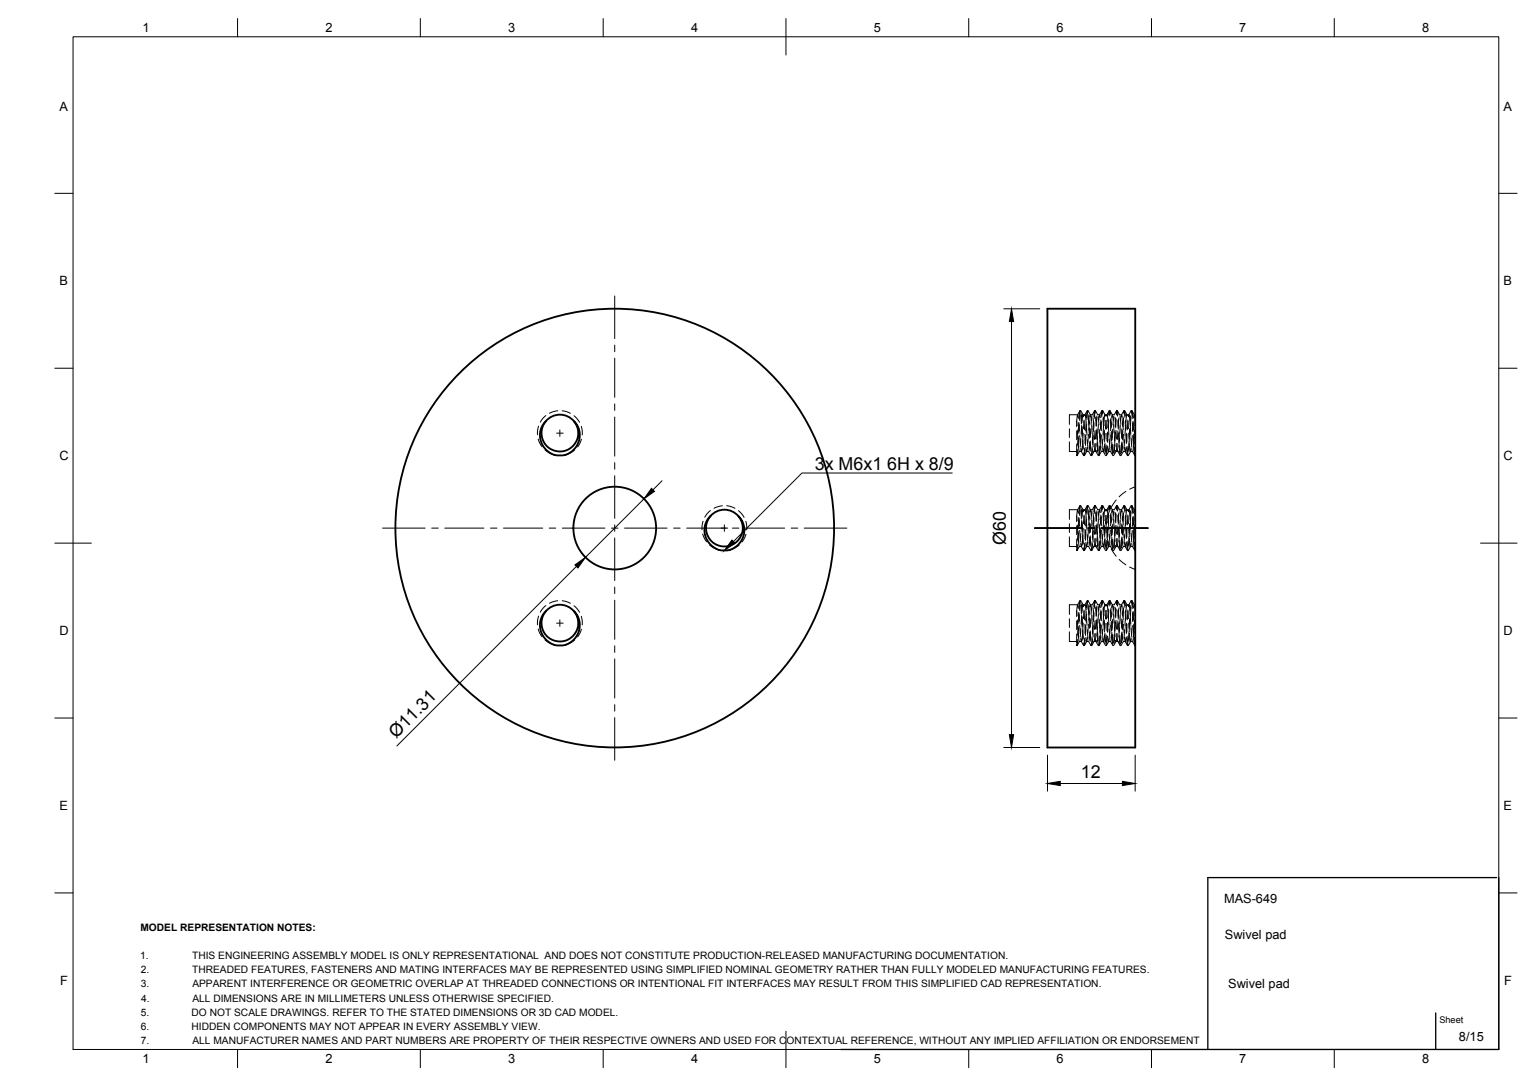
ISO-10303-21;
HEADER;
/* Generated by software containing ST-Developer
 * from STEP Tools, Inc. (www.steptools.com) 
 */

FILE_DESCRIPTION(
/* description */ ('Independent equipment support assembly with bolted 600 x 500 mm welde
d perimeter frame, four adjustable legs and swivel feet. Nominal overa
ll height 518 mm. No load rating assigned.'),
/* implementation_level */ '2;1');

FILE_NAME(
/* name */ 'Swivel pad.step',
/* time_stamp */ '2026-11-07T17:30:39-08:00',
/* author */ (''),
/* organization */ (''),
/* preprocessor_version */ 'ST-DEVELOPER v20.2',
/* originating_system */ 'Autodesk Translation Framework v15.17.0.0',
/* authorisation */ '');

FILE_SCHEMA (('AUTOMOTIVE_DESIGN { 1 0 10303 214 3 1 1 }'));
ENDSEC;

DATA;
#10=MECHANICAL_DESIGN_GEOMETRIC_PRESENTATION_REPRESENTATION('',(#2217),#63755);
#11=SPHERICAL_SURFACE('',#15224,6.);
#273=B_SPLINE_SURFACE_WITH_KNOTS('',3,3,((#49030,#49031,#49032,#49033,#49034,
#49035,#49036,#49037,#49038,#49039,#49040,#49041,#49042,#49043,#49044,#49045,
#49046,#49047,#49048,#49049,#49050,#49051,#49052,#49053,#49054,#49055,#49056,
#49057,#49058,#49059,#49060,#49061,#49062,#49063,#49064,#49065,#49066,#49067,
#49068,#49069,#49070,#49071,#49072,#49073,#49074,#49075,#49076,#49077,#49078,
#49079,#49080,#49081,#49082,#49083,#49084,#49085),(#49086,#49087,#49088,
#49089,#49090,#49091,#49092,#49093,#49094,#49095,#49096,#49097,#49098,#49099,
#49100,#49101,#49102,#49103,#49104,#49105,#49106,#49107,#49108,#49109,#49110,
#49111,#49112,#49113,#49114,#49115,#49116,#49117,#49118,#49119,#49120,#49121,
#49122,#49123,#49124,#49125,#49126,#49127,#49128,#49129,#49130,#49131,#49132,
#49133,#49134,#49135,#49136,#49137,#49138,#49139,#49140,#49141),(#49142,
#49143,#49144,#49145,#49146,#49147,#49148,#49149,#49150,#49151,#49152,#49153,
#49154,#49155,#49156,#49157,#49158,#49159,#49160,#49161,#49162,#49163,#49164,
#49165,#49166,#49167,#49168,#49169,#49170,#49171,#49172,#49173,#49174,#49175,
#49176,#49177,#49178,#49179,#49180,#49181,#49182,#49183,#49184,#49185,#49186,
#49187,#49188,#49189,#49190,#49191,#49192,#49193,#49194,#49195,#49196,#49197),
(#49198,#49199,#49200,#49201,#49202,#49203,#49204,#49205,#49206,#49207,
#49208,#49209,#49210,#49211,#49212,#49213,#49214,#49215,#49216,#49217,#49218,
#49219,#49220,#49221,#49222,#49223,#49224,#49225,#49226,#49227,#49228,#49229,
#49230,#49231,#49232,#49233,#49234,#49235,#49236,#49237,#49238,#49239,#49240,
#49241,#49242,#49243,#49244,#49245,#49246,#49247,#49248,#49249,#49250,#49251,
#49252,#49253)),.UNSPECIFIED.,.F.,.F.,.F.,(4,4),(4,1,1,1,1,1,1,1,1,1,1,
1,1,1,1,1,1,1,1,1,1,1,1,1,1,1,1,1,1,1,1,1,1,1,1,1,1,1,1,1,1,1,1,1,1,1,1,
1,1,1,1,1,1,4),(0.,0.0642013499338865),(11.8589888623078,12.8454497557128,
13.8319106491178,14.8183715425228,15.8048324359278,16.7912933293328,17.7777542227378,
18.7642151161428,19.7506760095478,20.7371369029528,21.7235977963578,22.7100586897628,
23.6965195831678,24.6829804765729,25.6694413699779,26.6559022633829,27.6423631567879,
28.6288240501929,29.6152849435979,30.6017458370029,31.5882067304079,32.5746676238129,
33.5611285172179,34.5475894106229,35.5340503040279,36.5205111974329,37.5069720908379,
38.4934329842429,39.4798938776479,40.4663547710529,41.4528156644579,42.4392765578629,
43.4257374512679,44.4121983446729,45.3986592380779,46.3851201314829,47.3715810248879,
48.3580419182929,49.3445028116979,50.3309637051029,51.3174245985079,52.3038854919129,
53.2903463853179,54.2768072787229,55.2632681721279,56.2497290655329,57.2361899589379,
58.2226508523429,59.2091117457479,60.1955726391529,61.1820335325579,62.1684944259629,
63.154955319368,64.141416212773),.UNSPECIFIED.);
#274=B_SPLINE_SURFACE_WITH_KNOTS('',3,3,((#49370,#49371,#49372,#49373,#49374,
#49375,#49376,#49377,#49378,#49379,#49380,#49381,#49382,#49383,#49384,#49385,
#49386,#49387,#49388,#49389,#49390,#49391,#49392,#49393,#49394,#49395,#49396,
#49397,#49398,#49399,#49400,#49401,#49402,#49403,#49404,#49405,#49406,#49407,
#49408,#49409,#49410,#49411,#49412,#49413,#49414,#49415,#49416,#49417,#49418,
#49419,#49420,#49421,#49422,#49423,#49424,#49425),(#49426,#49427,#49428,
#49429,#49430,#49431,#49432,#49433,#49434,#49435,#49436,#49437,#49438,#49439,
#49440,#49441,#49442,#49443,#49444,#49445,#49446,#49447,#49448,#49449,#49450,
#49451,#49452,#49453,#49454,#49455,#49456,#49457,#49458,#49459,#49460,#49461,
#49462,#49463,#49464,#49465,#49466,#49467,#49468,#49469,#49470,#49471,#49472,
#49473,#49474,#49475,#49476,#49477,#49478,#49479,#49480,#49481),(#49482,
#49483,#49484,#49485,#49486,#49487,#49488,#49489,#49490,#49491,#49492,#49493,
#49494,#49495,#49496,#49497,#49498,#49499,#49500,#49501,#49502,#49503,#49504,
#49505,#49506,#49507,#49508,#49509,#49510,#49511,#49512,#49513,#49514,#49515,
#49516,#49517,#49518,#49519,#49520,#49521,#49522,#49523,#49524,#49525,#49526,
#49527,#49528,#49529,#49530,#49531,#49532,#49533,#49534,#49535,#49536,#49537),
(#49538,#49539,#49540,#49541,#49542,#49543,#49544,#49545,#49546,#49547,
#49548,#49549,#49550,#49551,#49552,#49553,#49554,#49555,#49556,#49557,#49558,
#49559,#49560,#49561,#49562,#49563,#49564,#49565,#49566,#49567,#49568,#49569,
#49570,#49571,#49572,#49573,#49574,#49575,#49576,#49577,#49578,#49579,#49580,
#49581,#49582,#49583,#49584,#49585,#49586,#49587,#49588,#49589,#49590,#49591,
#49592,#49593)),.UNSPECIFIED.,.F.,.F.,.F.,(4,4),(4,1,1,1,1,1,1,1,1,1,1,
1,1,1,1,1,1,1,1,1,1,1,1,1,1,1,1,1,1,1,1,1,1,1,1,1,1,1,1,1,1,1,1,1,1,1,1,
1,1,1,1,1,1,4),(0.,0.0642013499338865),(14.3984001269719,15.3848610203769,
16.3713219137819,17.3577828071869,18.3442437005919,19.3307045939969,20.3171654874019,
21.3036263808069,22.2900872742119,23.2765481676169,24.2630090610219,25.2494699544269,
26.2359308478319,27.2223917412369,28.2088526346419,29.1953135280469,30.1817744214519,
31.1682353148569,32.1546962082619,33.1411571016669,34.1276179950719,35.1140788884769,
36.1005397818819,37.0870006752869,38.0734615686919,39.0599224620969,40.0463833555019,
41.0328442489069,42.0193051423119,43.0057660357169,43.9922269291219,44.9786878225269,
45.9651487159319,46.9516096093369,47.9380705027419,48.9245313961469,49.9109922895519,
50.897453182957,51.883914076362,52.870374969767,53.856835863172,54.843296756577,
55.829757649982,56.816218543387,57.802679436792,58.789140330197,59.775601223602,
60.762062117007,61.748523010412,62.734983903817,63.721444797222,64.707905690627,
65.694366584032,66.680827477437),.UNSPECIFIED.);
#275=B_SPLINE_SURFACE_WITH_KNOTS('',3,3,((#49922,#49923,#49924,#49925,#49926,
#49927,#49928,#49929,#49930,#49931,#49932,#49933,#49934,#49935,#49936,#49937,
#49938,#49939,#49940,#49941,#49942,#49943,#49944,#49945,#49946,#49947,#49948,
#49949,#49950,#49951,#49952,#49953,#49954,#49955,#49956,#49957,#49958,#49959,
#49960,#49961,#49962,#49963,#49964,#49965,#49966,#49967,#49968,#49969,#49970,
#49971,#49972,#49973,#49974,#49975,#49976,#49977),(#49978,#49979,#49980,
#49981,#49982,#49983,#49984,#49985,#49986,#49987,#49988,#49989,#49990,#49991,
#49992,#49993,#49994,#49995,#49996,#49997,#49998,#49999,#50000,#50001,#50002,
#50003,#50004,#50005,#50006,#50007,#50008,#50009,#50010,#50011,#50012,#50013,
#50014,#50015,#50016,#50017,#50018,#50019,#50020,#50021,#50022,#50023,#50024,
#50025,#50026,#50027,#50028,#50029,#50030,#50031,#50032,#50033),(#50034,
#50035,#50036,#50037,#50038,#50039,#50040,#50041,#50042,#50043,#50044,#50045,
#50046,#50047,#50048,#50049,#50050,#50051,#50052,#50053,#50054,#50055,#50056,
#50057,#50058,#50059,#50060,#50061,#50062,#50063,#50064,#50065,#50066,#50067,
#50068,#50069,#50070,#50071,#50072,#50073,#50074,#50075,#50076,#50077,#50078,
#50079,#50080,#50081,#50082,#50083,#50084,#50085,#50086,#50087,#50088,#50089),
(#50090,#50091,#50092,#50093,#50094,#50095,#50096,#50097,#50098,#50099,
#50100,#50101,#50102,#50103,#50104,#50105,#50106,#50107,#50108,#50109,#50110,
#50111,#50112,#50113,#50114,#50115,#50116,#50117,#50118,#50119,#50120,#50121,
#50122,#50123,#50124,#50125,#50126,#50127,#50128,#50129,#50130,#50131,#50132,
#50133,#50134,#50135,#50136,#50137,#50138,#50139,#50140,#50141,#50142,#50143,
#50144,#50145)),.UNSPECIFIED.,.F.,.F.,.F.,(4,4),(4,1,1,1,1,1,1,1,1,1,1,
1,1,1,1,1,1,1,1,1,1,1,1,1,1,1,1,1,1,1,1,1,1,1,1,1,1,1,1,1,1,1,1,1,1,1,1,
1,1,1,1,1,1,4),(0.,0.0642013499338863),(11.8589888623078,12.8454497557128,
13.8319106491178,14.8183715425228,15.8048324359278,16.7912933293328,17.7777542227378,
18.7642151161428,19.7506760095478,20.7371369029528,21.7235977963578,22.7100586897628,
23.6965195831678,24.6829804765729,25.6694413699779,26.6559022633829,27.6423631567879,
28.6288240501929,29.6152849435979,30.6017458370029,31.5882067304079,32.5746676238129,
33.5611285172179,34.5475894106229,35.5340503040279,36.5205111974329,37.5069720908379,
38.4934329842429,39.4798938776479,40.4663547710529,41.4528156644579,42.4392765578629,
43.4257374512679,44.4121983446729,45.3986592380779,46.3851201314829,47.3715810248879,
48.3580419182929,49.3445028116979,50.3309637051029,51.3174245985079,52.3038854919129,
53.2903463853179,54.2768072787229,55.2632681721279,56.2497290655329,57.2361899589379,
58.2226508523429,59.2091117457479,60.1955726391529,61.1820335325579,62.1684944259629,
63.154955319368,64.141416212773),.UNSPECIFIED.);
#276=B_SPLINE_SURFACE_WITH_KNOTS('',3,3,((#50262,#50263,#50264,#50265,#50266,
#50267,#50268,#50269,#50270,#50271,#50272,#50273,#50274,#50275,#50276,#50277,
#50278,#50279,#50280,#50281,#50282,#50283,#50284,#50285,#50286,#50287,#50288,
#50289,#50290,#50291,#50292,#50293,#50294,#50295,#50296,#50297,#50298,#50299,
#50300,#50301,#50302,#50303,#50304,#50305,#50306,#50307,#50308,#50309,#50310,
#50311,#50312,#50313,#50314,#50315,#50316,#50317),(#50318,#50319,#50320,
#50321,#50322,#50323,#50324,#50325,#50326,#50327,#50328,#50329,#50330,#50331,
#50332,#50333,#50334,#50335,#50336,#50337,#50338,#50339,#50340,#50341,#50342,
#50343,#50344,#50345,#50346,#50347,#50348,#50349,#50350,#50351,#50352,#50353,
#50354,#50355,#50356,#50357,#50358,#50359,#50360,#50361,#50362,#50363,#50364,
#50365,#50366,#50367,#50368,#50369,#50370,#50371,#50372,#50373),(#50374,
#50375,#50376,#50377,#50378,#50379,#50380,#50381,#50382,#50383,#50384,#50385,
#50386,#50387,#50388,#50389,#50390,#50391,#50392,#50393,#50394,#50395,#50396,
#50397,#50398,#50399,#50400,#50401,#50402,#50403,#50404,#50405,#50406,#50407,
#50408,#50409,#50410,#50411,#50412,#50413,#50414,#50415,#50416,#50417,#50418,
#50419,#50420,#50421,#50422,#50423,#50424,#50425,#50426,#50427,#50428,#50429),
(#50430,#50431,#50432,#50433,#50434,#50435,#50436,#50437,#50438,#50439,
#50440,#50441,#50442,#50443,#50444,#50445,#50446,#50447,#50448,#50449,#50450,
#50451,#50452,#50453,#50454,#50455,#50456,#50457,#50458,#50459,#50460,#50461,
#50462,#50463,#50464,#50465,#50466,#50467,#50468,#50469,#50470,#50471,#50472,
#50473,#50474,#50475,#50476,#50477,#50478,#50479,#50480,#50481,#50482,#50483,
#50484,#50485)),.UNSPECIFIED.,.F.,.F.,.F.,(4,4),(4,1,1,1,1,1,1,1,1,1,1,
1,1,1,1,1,1,1,1,1,1,1,1,1,1,1,1,1,1,1,1,1,1,1,1,1,1,1,1,1,1,1,1,1,1,1,1,
1,1,1,1,1,1,4),(0.,0.0642013499338863),(14.3984001269719,15.3848610203769,
16.3713219137819,17.3577828071869,18.3442437005919,19.3307045939969,20.3171654874019,
21.3036263808069,22.2900872742119,23.2765481676169,24.2630090610219,25.2494699544269,
26.2359308478319,27.2223917412369,28.2088526346419,29.1953135280469,30.1817744214519,
31.1682353148569,32.1546962082619,33.1411571016669,34.1276179950719,35.1140788884769,
36.1005397818819,37.0870006752869,38.0734615686919,39.0599224620969,40.0463833555019,
41.0328442489069,42.0193051423119,43.0057660357169,43.9922269291219,44.9786878225269,
45.9651487159319,46.9516096093369,47.9380705027419,48.9245313961469,49.9109922895519,
50.897453182957,51.883914076362,52.870374969767,53.856835863172,54.843296756577,
55.829757649982,56.816218543387,57.802679436792,58.789140330197,59.775601223602,
60.762062117007,61.748523010412,62.734983903817,63.721444797222,64.707905690627,
65.694366584032,66.680827477437),.UNSPECIFIED.);
#277=B_SPLINE_SURFACE_WITH_KNOTS('',3,3,((#50814,#50815,#50816,#50817,#50818,
#50819,#50820,#50821,#50822,#50823,#50824,#50825,#50826,#50827,#50828,#50829,
#50830,#50831,#50832,#50833,#50834,#50835,#50836,#50837,#50838,#50839,#50840,
#50841,#50842,#50843,#50844,#50845,#50846,#50847,#50848,#50849,#50850,#50851,
#50852,#50853,#50854,#50855,#50856,#50857,#50858,#50859,#50860,#50861,#50862,
#50863,#50864,#50865,#50866,#50867,#50868,#50869),(#50870,#50871,#50872,
#50873,#50874,#50875,#50876,#50877,#50878,#50879,#50880,#50881,#50882,#50883,
#50884,#50885,#50886,#50887,#50888,#50889,#50890,#50891,#50892,#50893,#50894,
#50895,#50896,#50897,#50898,#50899,#50900,#50901,#50902,#50903,#50904,#50905,
#50906,#50907,#50908,#50909,#50910,#50911,#50912,#50913,#50914,#50915,#50916,
#50917,#50918,#50919,#50920,#50921,#50922,#50923,#50924,#50925),(#50926,
#50927,#50928,#50929,#50930,#50931,#50932,#50933,#50934,#50935,#50936,#50937,
#50938,#50939,#50940,#50941,#50942,#50943,#50944,#50945,#50946,#50947,#50948,
#50949,#50950,#50951,#50952,#50953,#50954,#50955,#50956,#50957,#50958,#50959,
#50960,#50961,#50962,#50963,#50964,#50965,#50966,#50967,#50968,#50969,#50970,
#50971,#50972,#50973,#50974,#50975,#50976,#50977,#50978,#50979,#50980,#50981),
(#50982,#50983,#50984,#50985,#50986,#50987,#50988,#50989,#50990,#50991,
#50992,#50993,#50994,#50995,#50996,#50997,#50998,#50999,#51000,#51001,#51002,
#51003,#51004,#51005,#51006,#51007,#51008,#51009,#51010,#51011,#51012,#51013,
#51014,#51015,#51016,#51017,#51018,#51019,#51020,#51021,#51022,#51023,#51024,
#51025,#51026,#51027,#51028,#51029,#51030,#51031,#51032,#51033,#51034,#51035,
#51036,#51037)),.UNSPECIFIED.,.F.,.F.,.F.,(4,4),(4,1,1,1,1,1,1,1,1,1,1,
1,1,1,1,1,1,1,1,1,1,1,1,1,1,1,1,1,1,1,1,1,1,1,1,1,1,1,1,1,1,1,1,1,1,1,1,
1,1,1,1,1,1,4),(0.,0.0642013499338863),(11.8589888623078,12.8454497557128,
13.8319106491178,14.8183715425228,15.8048324359278,16.7912933293328,17.7777542227378,
18.7642151161429,19.7506760095479,20.7371369029529,21.7235977963579,22.7100586897629,
23.6965195831679,24.6829804765729,25.6694413699779,26.6559022633829,27.6423631567879,
28.6288240501929,29.6152849435979,30.6017458370029,31.5882067304079,32.5746676238129,
33.5611285172179,34.5475894106229,35.5340503040279,36.5205111974329,37.5069720908379,
38.4934329842429,39.4798938776479,40.4663547710529,41.4528156644579,42.4392765578629,
43.4257374512679,44.4121983446729,45.3986592380779,46.3851201314829,47.3715810248879,
48.3580419182929,49.3445028116979,50.3309637051029,51.3174245985079,52.3038854919129,
53.2903463853179,54.2768072787229,55.2632681721279,56.2497290655329,57.2361899589379,
58.222650852343,59.209111745748,60.195572639153,61.182033532558,62.168494425963,
63.154955319368,64.141416212773),.UNSPECIFIED.);
#278=B_SPLINE_SURFACE_WITH_KNOTS('',3,3,((#51154,#51155,#51156,#51157,#51158,
#51159,#51160,#51161,#51162,#51163,#51164,#51165,#51166,#51167,#51168,#51169,
#51170,#51171,#51172,#51173,#51174,#51175,#51176,#51177,#51178,#51179,#51180,
#51181,#51182,#51183,#51184,#51185,#51186,#51187,#51188,#51189,#51190,#51191,
#51192,#51193,#51194,#51195,#51196,#51197,#51198,#51199,#51200,#51201,#51202,
#51203,#51204,#51205,#51206,#51207,#51208,#51209),(#51210,#51211,#51212,
#51213,#51214,#51215,#51216,#51217,#51218,#51219,#51220,#51221,#51222,#51223,
#51224,#51225,#51226,#51227,#51228,#51229,#51230,#51231,#51232,#51233,#51234,
#51235,#51236,#51237,#51238,#51239,#51240,#51241,#51242,#51243,#51244,#51245,
#51246,#51247,#51248,#51249,#51250,#51251,#51252,#51253,#51254,#51255,#51256,
#51257,#51258,#51259,#51260,#51261,#51262,#51263,#51264,#51265),(#51266,
#51267,#51268,#51269,#51270,#51271,#51272,#51273,#51274,#51275,#51276,#51277,
#51278,#51279,#51280,#51281,#51282,#51283,#51284,#51285,#51286,#51287,#51288,
#51289,#51290,#51291,#51292,#51293,#51294,#51295,#51296,#51297,#51298,#51299,
#51300,#51301,#51302,#51303,#51304,#51305,#51306,#51307,#51308,#51309,#51310,
#51311,#51312,#51313,#51314,#51315,#51316,#51317,#51318,#51319,#51320,#51321),
(#51322,#51323,#51324,#51325,#51326,#51327,#51328,#51329,#51330,#51331,
#51332,#51333,#51334,#51335,#51336,#51337,#51338,#51339,#51340,#51341,#51342,
#51343,#51344,#51345,#51346,#51347,#51348,#51349,#51350,#51351,#51352,#51353,
#51354,#51355,#51356,#51357,#51358,#51359,#51360,#51361,#51362,#51363,#51364,
#51365,#51366,#51367,#51368,#51369,#51370,#51371,#51372,#51373,#51374,#51375,
#51376,#51377)),.UNSPECIFIED.,.F.,.F.,.F.,(4,4),(4,1,1,1,1,1,1,1,1,1,1,
1,1,1,1,1,1,1,1,1,1,1,1,1,1,1,1,1,1,1,1,1,1,1,1,1,1,1,1,1,1,1,1,1,1,1,1,
1,1,1,1,1,1,4),(0.,0.0642013499338863),(14.3984001269719,15.3848610203769,
16.3713219137819,17.3577828071869,18.3442437005919,19.3307045939969,20.3171654874019,
21.3036263808069,22.2900872742119,23.2765481676169,24.2630090610219,25.2494699544269,
26.2359308478319,27.2223917412369,28.2088526346419,29.1953135280469,30.1817744214519,
31.1682353148569,32.1546962082619,33.1411571016669,34.1276179950719,35.1140788884769,
36.1005397818819,37.0870006752869,38.0734615686919,39.0599224620969,40.0463833555019,
41.0328442489069,42.0193051423119,43.0057660357169,43.9922269291219,44.978687822527,
45.965148715932,46.951609609337,47.938070502742,48.924531396147,49.910992289552,
50.897453182957,51.883914076362,52.870374969767,53.856835863172,54.843296756577,
55.829757649982,56.816218543387,57.802679436792,58.789140330197,59.775601223602,
60.762062117007,61.748523010412,62.734983903817,63.721444797222,64.707905690627,
65.694366584032,66.680827477437),.UNSPECIFIED.);
#427=CIRCLE('',#15147,2.5175);
#428=CIRCLE('',#15148,2.5175);
#429=CIRCLE('',#15149,2.5175);
#430=CIRCLE('',#15157,2.5175);
#431=CIRCLE('',#15159,3.0735);
#432=CIRCLE('',#15167,3.0735);
#433=CIRCLE('',#15169,2.5175);
#434=CIRCLE('',#15170,2.5175);
#435=CIRCLE('',#15171,2.5175);
#436=CIRCLE('',#15179,2.5175);
#437=CIRCLE('',#15181,3.0735);
#438=CIRCLE('',#15189,3.0735);
#439=CIRCLE('',#15191,2.5175);
#440=CIRCLE('',#15192,2.5175);
#441=CIRCLE('',#15193,2.5175);
#442=CIRCLE('',#15201,2.5175);
#443=CIRCLE('',#15203,3.0735);
#444=CIRCLE('',#15211,3.0735);
#445=CIRCLE('',#15225,5.65685424949238);
#446=CIRCLE('',#15226,6.);
#447=CIRCLE('',#15228,30.);
#448=CIRCLE('',#15229,30.);
#1113=B_SPLINE_CURVE_WITH_KNOTS('',3,(#47159,#47160,#47161,#47162),
 .UNSPECIFIED.,.F.,.F.,(4,4),(51.5750455984138,52.2824273504651),
 .UNSPECIFIED.);
#1114=B_SPLINE_CURVE_WITH_KNOTS('',3,(#47170,#47171,#47172,#47173,#47174,
#47175,#47176,#47177,#47178,#47179),.UNSPECIFIED.,.F.,.F.,(4,3,3,4),(-50.2654824574367,
-49.3230446702501,-48.3365837768451,-47.8312715558982),.UNSPECIFIED.);
#1115=B_SPLINE_CURVE_WITH_KNOTS('',3,(#47184,#47185,#47186,#47187,#47188,
#47189,#47190,#47191,#47192,#47193,#47194,#47195,#47196,#47197,#47198,#47199,
#47200,#47201,#47202,#47203,#47204,#47205,#47206,#47207,#47208),
 .UNSPECIFIED.,.F.,.F.,(4,3,3,3,3,3,3,3,4),(45.2918602912342,45.3772010966301,
46.3636619900351,47.3501228834401,48.3365837768451,49.3230446702501,50.3095055636551,
51.2959664570601,51.5750455984138),.UNSPECIFIED.);
#1116=B_SPLINE_CURVE_WITH_KNOTS('',3,(#47209,#47210,#47211,#47212,#47213,
#47214,#47215,#47216,#47217,#47218,#47219,#47220,#47221,#47222,#47223,#47224,
#47225,#47226,#47227,#47228,#47229,#47230),.UNSPECIFIED.,.F.,.F.,(4,3,3,
3,3,3,3,4),(-47.8312715558982,-47.3501228834401,-46.3636619900351,-45.3772010966301,
-44.3907402032251,-43.4042793098201,-42.4178184164151,-41.5480862487186),
 .UNSPECIFIED.);
#1117=B_SPLINE_CURVE_WITH_KNOTS('',3,(#47235,#47236,#47237,#47238,#47239,
#47240,#47241,#47242,#47243,#47244,#47245,#47246,#47247,#47248,#47249,#47250,
#47251,#47252,#47253,#47254,#47255,#47256),.UNSPECIFIED.,.F.,.F.,(4,3,3,
3,3,3,3,4),(39.0086749840546,39.4584357362001,40.4448966296051,41.4313575230101,
42.4178184164151,43.4042793098201,44.3907402032251,45.2918602912342),
 .UNSPECIFIED.);
#1118=B_SPLINE_CURVE_WITH_KNOTS('',3,(#47257,#47258,#47259,#47260,#47261,
#47262,#47263,#47264,#47265,#47266,#47267,#47268,#47269,#47270,#47271,#47272,
#47273,#47274,#47275,#47276,#47277,#47278,#47279,#47280,#47281),
 .UNSPECIFIED.,.F.,.F.,(4,3,3,3,3,3,3,3,4),(-41.5480862487186,-41.4313575230101,
-40.4448966296051,-39.4584357362001,-38.4719748427951,-37.4855139493901,
-36.4990530559851,-35.5125921625801,-35.264900941539),.UNSPECIFIED.);
#1119=B_SPLINE_CURVE_WITH_KNOTS('',3,(#47286,#47287,#47288,#47289,#47290,
#47291,#47292,#47293,#47294,#47295,#47296,#47297,#47298,#47299,#47300,#47301,
#47302,#47303,#47304,#47305,#47306,#47307),.UNSPECIFIED.,.F.,.F.,(4,3,3,
3,3,3,3,4),(32.725489676875,33.5396703757701,34.5261312691751,35.5125921625801,
36.4990530559851,37.4855139493901,38.4719748427951,39.0086749840546),
 .UNSPECIFIED.);
#1120=B_SPLINE_CURVE_WITH_KNOTS('',3,(#47308,#47309,#47310,#47311,#47312,
#47313,#47314,#47315,#47316,#47317,#47318,#47319,#47320,#47321,#47322,#47323,
#47324,#47325,#47326,#47327,#47328,#47329),.UNSPECIFIED.,.F.,.F.,(4,3,3,
3,3,3,3,4),(-35.264900941539,-34.5261312691751,-33.5396703757701,-32.5532094823651,
-31.5667485889601,-30.5802876955551,-29.5938268021501,-28.9817156343595),
 .UNSPECIFIED.);
#1121=B_SPLINE_CURVE_WITH_KNOTS('',3,(#47334,#47335,#47336,#47337,#47338,
#47339,#47340,#47341,#47342,#47343,#47344,#47345,#47346,#47347,#47348,#47349,
#47350,#47351,#47352,#47353,#47354,#47355,#47356,#47357,#47358),
 .UNSPECIFIED.,.F.,.F.,(4,3,3,3,3,3,3,3,4),(26.4423043696954,26.6344441219351,
27.6209050153401,28.6073659087451,29.5938268021501,30.5802876955551,31.5667485889601,
32.5532094823651,32.725489676875),.UNSPECIFIED.);
#1122=B_SPLINE_CURVE_WITH_KNOTS('',3,(#47359,#47360,#47361,#47362,#47363,
#47364,#47365,#47366,#47367,#47368,#47369,#47370,#47371,#47372,#47373,#47374,
#47375,#47376,#47377,#47378,#47379,#47380),.UNSPECIFIED.,.F.,.F.,(4,3,3,
3,3,3,3,4),(-28.9817156343595,-28.6073659087451,-27.6209050153401,-26.6344441219351,
-25.6479832285301,-24.6615223351251,-23.6750614417201,-22.6985303271799),
 .UNSPECIFIED.);
#1123=B_SPLINE_CURVE_WITH_KNOTS('',3,(#47385,#47386,#47387,#47388,#47389,
#47390,#47391,#47392,#47393,#47394,#47395,#47396,#47397,#47398,#47399,#47400,
#47401,#47402,#47403,#47404,#47405,#47406),.UNSPECIFIED.,.F.,.F.,(4,3,3,
3,3,3,3,4),(20.1591190625158,20.7156787615051,21.7021396549101,22.6886005483151,
23.6750614417201,24.6615223351251,25.6479832285301,26.4423043696954),
 .UNSPECIFIED.);
#1124=B_SPLINE_CURVE_WITH_KNOTS('',3,(#47407,#47408,#47409,#47410,#47411,
#47412,#47413,#47414,#47415,#47416,#47417,#47418,#47419,#47420,#47421,#47422,
#47423,#47424,#47425,#47426,#47427,#47428,#47429,#47430,#47431),
 .UNSPECIFIED.,.F.,.F.,(4,3,3,3,3,3,3,3,4),(-22.6985303271799,-22.6886005483151,
-21.7021396549101,-20.7156787615051,-19.7292178681001,-18.7427569746951,
-17.75629608129,-16.769835187885,-16.4153450200003),.UNSPECIFIED.);
#1125=B_SPLINE_CURVE_WITH_KNOTS('',3,(#47436,#47437,#47438,#47439,#47440,
#47441,#47442,#47443,#47444,#47445,#47446,#47447,#47448,#47449,#47450,#47451,
#47452,#47453,#47454,#47455,#47456,#47457),.UNSPECIFIED.,.F.,.F.,(4,3,3,
3,3,3,3,4),(13.8759337553362,14.796913401075,15.78337429448,16.769835187885,
17.75629608129,18.7427569746951,19.7292178681001,20.1591190625158),
 .UNSPECIFIED.);
#1126=B_SPLINE_CURVE_WITH_KNOTS('',3,(#47458,#47459,#47460,#47461,#47462,
#47463,#47464,#47465,#47466,#47467,#47468,#47469,#47470,#47471,#47472,#47473,
#47474,#47475,#47476,#47477,#47478,#47479),.UNSPECIFIED.,.F.,.F.,(4,3,3,
3,3,3,3,4),(-16.4153450200003,-15.78337429448,-14.796913401075,-13.81045250767,
-12.823991614265,-11.83753072086,-10.851069827455,-10.1321597128207),
 .UNSPECIFIED.);
#1127=B_SPLINE_CURVE_WITH_KNOTS('',3,(#47485,#47486,#47487,#47488,#47489,
#47490,#47491,#47492,#47493,#47494,#47495,#47496,#47497),.UNSPECIFIED.,
 .F.,.F.,(4,3,3,3,4),(-3.84897440564112,-2.95938268021501,-1.97292178681001,
-0.986460893405003,0.),.UNSPECIFIED.);
#1128=B_SPLINE_CURVE_WITH_KNOTS('',3,(#47500,#47501,#47502,#47503,#47504,
#47505,#47506,#47507,#47508,#47509,#47510,#47511,#47512,#47513,#47514,#47515,
#47516,#47517,#47518),.UNSPECIFIED.,.F.,.F.,(4,3,3,3,3,3,4),(2.01694489302844,
2.95938268021501,3.94584357362001,4.93230446702501,5.91876536043001,6.90522625383502,
7.59274844815664),.UNSPECIFIED.);
#1129=B_SPLINE_CURVE_WITH_KNOTS('',3,(#47524,#47525,#47526,#47527,#47528,
#47529,#47530,#47531),.UNSPECIFIED.,.F.,.F.,(4,1,1,1,1,4),(59.6902604182061,
60.195572639153,61.182033532558,62.168494425963,63.154955319368,64.141416212773),
 .UNSPECIFIED.);
#1130=B_SPLINE_CURVE_WITH_KNOTS('',3,(#47534,#47535,#47536,#47537,#47538,
#47539,#47540,#47541,#47542),.UNSPECIFIED.,.F.,.F.,(4,1,1,1,1,1,4),(59.6902604182061,
59.775601223602,60.762062117007,61.748523010412,62.734983903817,63.721444797222,
64.6638825844085),.UNSPECIFIED.);
#1131=B_SPLINE_CURVE_WITH_KNOTS('',3,(#47547,#47548,#47549,#47550,#47551,
#47552,#47553,#47554,#47555,#47556),.UNSPECIFIED.,.F.,.F.,(4,1,1,1,1,1,
1,4),(53.4070751110265,54.2768072787229,55.2632681721279,56.2497290655329,
57.2361899589379,58.222650852343,59.209111745748,59.6902604182061),
 .UNSPECIFIED.);
#1132=B_SPLINE_CURVE_WITH_KNOTS('',3,(#47557,#47558,#47559,#47560,#47561,
#47562,#47563,#47564,#47565,#47566),.UNSPECIFIED.,.F.,.F.,(4,1,1,1,1,1,
1,4),(53.4070751110265,53.856835863172,54.843296756577,55.829757649982,
56.816218543387,57.802679436792,58.789140330197,59.6902604182061),
 .UNSPECIFIED.);
#1133=B_SPLINE_CURVE_WITH_KNOTS('',3,(#47571,#47572,#47573,#47574,#47575,
#47576,#47577,#47578,#47579,#47580,#47581),.UNSPECIFIED.,.F.,.F.,(4,1,1,
1,1,1,1,1,4),(47.1238898038469,47.3715810248879,48.3580419182929,49.3445028116979,
50.3309637051029,51.3174245985079,52.3038854919129,53.2903463853179,53.4070751110265),
 .UNSPECIFIED.);
#1134=B_SPLINE_CURVE_WITH_KNOTS('',3,(#47582,#47583,#47584,#47585,#47586,
#47587,#47588,#47589,#47590,#47591),.UNSPECIFIED.,.F.,.F.,(4,1,1,1,1,1,
1,4),(47.1238898038469,47.938070502742,48.924531396147,49.910992289552,
50.897453182957,51.883914076362,52.870374969767,53.4070751110265),
 .UNSPECIFIED.);
#1135=B_SPLINE_CURVE_WITH_KNOTS('',3,(#47596,#47597,#47598,#47599,#47600,
#47601,#47602,#47603,#47604,#47605),.UNSPECIFIED.,.F.,.F.,(4,1,1,1,1,1,
1,4),(40.8407044966673,41.4528156644579,42.4392765578629,43.4257374512679,
44.4121983446729,45.3986592380779,46.3851201314829,47.1238898038469),
 .UNSPECIFIED.);
#1136=B_SPLINE_CURVE_WITH_KNOTS('',3,(#47606,#47607,#47608,#47609,#47610,
#47611,#47612,#47613,#47614,#47615,#47616),.UNSPECIFIED.,.F.,.F.,(4,1,1,
1,1,1,1,1,4),(40.8407044966673,41.0328442489069,42.0193051423119,43.0057660357169,
43.9922269291219,44.978687822527,45.965148715932,46.951609609337,47.1238898038469),
 .UNSPECIFIED.);
#1137=B_SPLINE_CURVE_WITH_KNOTS('',3,(#47621,#47622,#47623,#47624,#47625,
#47626,#47627,#47628,#47629,#47630),.UNSPECIFIED.,.F.,.F.,(4,1,1,1,1,1,
1,4),(34.5575191894877,35.5340503040279,36.5205111974329,37.5069720908379,
38.4934329842429,39.4798938776479,40.4663547710529,40.8407044966673),
 .UNSPECIFIED.);
#1138=B_SPLINE_CURVE_WITH_KNOTS('',3,(#47631,#47632,#47633,#47634,#47635,
#47636,#47637,#47638,#47639,#47640),.UNSPECIFIED.,.F.,.F.,(4,1,1,1,1,1,
1,4),(34.5575191894877,35.1140788884769,36.1005397818819,37.0870006752869,
38.0734615686919,39.0599224620969,40.0463833555019,40.8407044966673),
 .UNSPECIFIED.);
#1139=B_SPLINE_CURVE_WITH_KNOTS('',3,(#47645,#47646,#47647,#47648,#47649,
#47650,#47651,#47652,#47653,#47654,#47655),.UNSPECIFIED.,.F.,.F.,(4,1,1,
1,1,1,1,1,4),(28.2743338823081,28.6288240501929,29.6152849435979,30.6017458370029,
31.5882067304079,32.5746676238129,33.5611285172179,34.5475894106229,34.5575191894877),
 .UNSPECIFIED.);
#1140=B_SPLINE_CURVE_WITH_KNOTS('',3,(#47656,#47657,#47658,#47659,#47660,
#47661,#47662,#47663,#47664,#47665),.UNSPECIFIED.,.F.,.F.,(4,1,1,1,1,1,
1,4),(28.2743338823081,29.1953135280469,30.1817744214519,31.1682353148569,
32.1546962082619,33.1411571016669,34.1276179950719,34.5575191894877),
 .UNSPECIFIED.);
#1141=B_SPLINE_CURVE_WITH_KNOTS('',3,(#47670,#47671,#47672,#47673,#47674,
#47675,#47676,#47677,#47678,#47679),.UNSPECIFIED.,.F.,.F.,(4,1,1,1,1,1,
1,4),(21.9911485751285,22.7100586897629,23.6965195831679,24.6829804765729,
25.6694413699779,26.6559022633829,27.6423631567879,28.2743338823081),
 .UNSPECIFIED.);
#1142=B_SPLINE_CURVE_WITH_KNOTS('',3,(#47680,#47681,#47682,#47683,#47684,
#47685,#47686,#47687,#47688,#47689,#47690),.UNSPECIFIED.,.F.,.F.,(4,1,1,
1,1,1,1,1,4),(21.9911485751285,22.2900872742119,23.2765481676169,24.2630090610219,
25.2494699544269,26.2359308478319,27.2223917412369,28.2088526346419,28.2743338823081),
 .UNSPECIFIED.);
#1143=B_SPLINE_CURVE_WITH_KNOTS('',3,(#47696,#47697,#47698,#47699,#47700),
 .UNSPECIFIED.,.F.,.F.,(4,1,4),(14.3984001269719,15.3848610203769,15.7079632679489),
 .UNSPECIFIED.);
#1144=B_SPLINE_CURVE_WITH_KNOTS('',3,(#47703,#47704,#47705,#47706,#47707),
 .UNSPECIFIED.,.F.,.F.,(4,1,4),(13.8759337553363,14.8183715425228,15.7079632679489),
 .UNSPECIFIED.);
#1145=B_SPLINE_CURVE_WITH_KNOTS('',3,(#47713,#47714,#47715,#47716),
 .UNSPECIFIED.,.F.,.F.,(4,4),(51.5750455984138,52.2824273504651),
 .UNSPECIFIED.);
#1146=B_SPLINE_CURVE_WITH_KNOTS('',3,(#47724,#47725,#47726,#47727,#47728,
#47729,#47730,#47731,#47732,#47733),.UNSPECIFIED.,.F.,.F.,(4,3,3,4),(-50.2654824574367,
-49.3230446702501,-48.3365837768451,-47.8312715558982),.UNSPECIFIED.);
#1147=B_SPLINE_CURVE_WITH_KNOTS('',3,(#47738,#47739,#47740,#47741,#47742,
#47743,#47744,#47745,#47746,#47747,#47748,#47749,#47750,#47751,#47752,#47753,
#47754,#47755,#47756,#47757,#47758,#47759,#47760,#47761,#47762),
 .UNSPECIFIED.,.F.,.F.,(4,3,3,3,3,3,3,3,4),(45.2918602912342,45.3772010966301,
46.3636619900351,47.3501228834401,48.3365837768451,49.3230446702501,50.3095055636551,
51.2959664570601,51.5750455984138),.UNSPECIFIED.);
#1148=B_SPLINE_CURVE_WITH_KNOTS('',3,(#47763,#47764,#47765,#47766,#47767,
#47768,#47769,#47770,#47771,#47772,#47773,#47774,#47775,#47776,#47777,#47778,
#47779,#47780,#47781,#47782,#47783,#47784),.UNSPECIFIED.,.F.,.F.,(4,3,3,
3,3,3,3,4),(-47.8312715558982,-47.3501228834401,-46.3636619900351,-45.3772010966301,
-44.3907402032251,-43.4042793098201,-42.4178184164151,-41.5480862487186),
 .UNSPECIFIED.);
#1149=B_SPLINE_CURVE_WITH_KNOTS('',3,(#47789,#47790,#47791,#47792,#47793,
#47794,#47795,#47796,#47797,#47798,#47799,#47800,#47801,#47802,#47803,#47804,
#47805,#47806,#47807,#47808,#47809,#47810),.UNSPECIFIED.,.F.,.F.,(4,3,3,
3,3,3,3,4),(39.0086749840546,39.4584357362001,40.4448966296051,41.4313575230101,
42.4178184164151,43.4042793098201,44.3907402032251,45.2918602912342),
 .UNSPECIFIED.);
#1150=B_SPLINE_CURVE_WITH_KNOTS('',3,(#47811,#47812,#47813,#47814,#47815,
#47816,#47817,#47818,#47819,#47820,#47821,#47822,#47823,#47824,#47825,#47826,
#47827,#47828,#47829,#47830,#47831,#47832,#47833,#47834,#47835),
 .UNSPECIFIED.,.F.,.F.,(4,3,3,3,3,3,3,3,4),(-41.5480862487186,-41.4313575230101,
-40.4448966296051,-39.4584357362001,-38.4719748427951,-37.4855139493901,
-36.4990530559851,-35.5125921625801,-35.2649009415391),.UNSPECIFIED.);
#1151=B_SPLINE_CURVE_WITH_KNOTS('',3,(#47840,#47841,#47842,#47843,#47844,
#47845,#47846,#47847,#47848,#47849,#47850,#47851,#47852,#47853,#47854,#47855,
#47856,#47857,#47858,#47859,#47860,#47861),.UNSPECIFIED.,.F.,.F.,(4,3,3,
3,3,3,3,4),(32.725489676875,33.5396703757701,34.5261312691751,35.5125921625801,
36.4990530559851,37.4855139493901,38.4719748427951,39.0086749840546),
 .UNSPECIFIED.);
#1152=B_SPLINE_CURVE_WITH_KNOTS('',3,(#47862,#47863,#47864,#47865,#47866,
#47867,#47868,#47869,#47870,#47871,#47872,#47873,#47874,#47875,#47876,#47877,
#47878,#47879,#47880,#47881,#47882,#47883),.UNSPECIFIED.,.F.,.F.,(4,3,3,
3,3,3,3,4),(-35.2649009415391,-34.5261312691751,-33.5396703757701,-32.5532094823651,
-31.5667485889601,-30.5802876955551,-29.5938268021501,-28.9817156343595),
 .UNSPECIFIED.);
#1153=B_SPLINE_CURVE_WITH_KNOTS('',3,(#47888,#47889,#47890,#47891,#47892,
#47893,#47894,#47895,#47896,#47897,#47898,#47899,#47900,#47901,#47902,#47903,
#47904,#47905,#47906,#47907,#47908,#47909,#47910,#47911,#47912),
 .UNSPECIFIED.,.F.,.F.,(4,3,3,3,3,3,3,3,4),(26.4423043696954,26.6344441219351,
27.6209050153401,28.6073659087451,29.5938268021501,30.5802876955551,31.5667485889601,
32.5532094823651,32.725489676875),.UNSPECIFIED.);
#1154=B_SPLINE_CURVE_WITH_KNOTS('',3,(#47913,#47914,#47915,#47916,#47917,
#47918,#47919,#47920,#47921,#47922,#47923,#47924,#47925,#47926,#47927,#47928,
#47929,#47930,#47931,#47932,#47933,#47934),.UNSPECIFIED.,.F.,.F.,(4,3,3,
3,3,3,3,4),(-28.9817156343595,-28.6073659087451,-27.6209050153401,-26.6344441219351,
-25.6479832285301,-24.6615223351251,-23.6750614417201,-22.6985303271799),
 .UNSPECIFIED.);
#1155=B_SPLINE_CURVE_WITH_KNOTS('',3,(#47939,#47940,#47941,#47942,#47943,
#47944,#47945,#47946,#47947,#47948,#47949,#47950,#47951,#47952,#47953,#47954,
#47955,#47956,#47957,#47958,#47959,#47960),.UNSPECIFIED.,.F.,.F.,(4,3,3,
3,3,3,3,4),(20.1591190625158,20.7156787615051,21.7021396549101,22.6886005483151,
23.6750614417201,24.6615223351251,25.6479832285301,26.4423043696954),
 .UNSPECIFIED.);
#1156=B_SPLINE_CURVE_WITH_KNOTS('',3,(#47961,#47962,#47963,#47964,#47965,
#47966,#47967,#47968,#47969,#47970,#47971,#47972,#47973,#47974,#47975,#47976,
#47977,#47978,#47979,#47980,#47981,#47982,#47983,#47984,#47985),
 .UNSPECIFIED.,.F.,.F.,(4,3,3,3,3,3,3,3,4),(-22.6985303271799,-22.6886005483151,
-21.70213965491,-20.715678761505,-19.7292178681,-18.742756974695,-17.75629608129,
-16.769835187885,-16.4153450200003),.UNSPECIFIED.);
#1157=B_SPLINE_CURVE_WITH_KNOTS('',3,(#47990,#47991,#47992,#47993,#47994,
#47995,#47996,#47997,#47998,#47999,#48000,#48001,#48002,#48003,#48004,#48005,
#48006,#48007,#48008,#48009,#48010,#48011),.UNSPECIFIED.,.F.,.F.,(4,3,3,
3,3,3,3,4),(13.8759337553362,14.796913401075,15.78337429448,16.769835187885,
17.7562960812901,18.7427569746951,19.7292178681001,20.1591190625158),
 .UNSPECIFIED.);
#1158=B_SPLINE_CURVE_WITH_KNOTS('',3,(#48012,#48013,#48014,#48015,#48016,
#48017,#48018,#48019,#48020,#48021,#48022,#48023,#48024,#48025,#48026,#48027,
#48028,#48029,#48030,#48031,#48032,#48033),.UNSPECIFIED.,.F.,.F.,(4,3,3,
3,3,3,3,4),(-16.4153450200003,-15.78337429448,-14.796913401075,-13.81045250767,
-12.823991614265,-11.83753072086,-10.851069827455,-10.1321597128207),
 .UNSPECIFIED.);
#1159=B_SPLINE_CURVE_WITH_KNOTS('',3,(#48039,#48040,#48041,#48042,#48043,
#48044,#48045,#48046,#48047,#48048,#48049,#48050,#48051),.UNSPECIFIED.,
 .F.,.F.,(4,3,3,3,4),(-3.84897440564113,-2.95938268021501,-1.97292178681,
-0.986460893405001,0.),.UNSPECIFIED.);
#1160=B_SPLINE_CURVE_WITH_KNOTS('',3,(#48054,#48055,#48056,#48057,#48058,
#48059,#48060,#48061,#48062,#48063,#48064,#48065,#48066,#48067,#48068,#48069,
#48070,#48071,#48072),.UNSPECIFIED.,.F.,.F.,(4,3,3,3,3,3,4),(2.01694489302845,
2.95938268021501,3.94584357362001,4.93230446702501,5.91876536043002,6.90522625383501,
7.59274844815666),.UNSPECIFIED.);
#1161=B_SPLINE_CURVE_WITH_KNOTS('',3,(#48078,#48079,#48080,#48081,#48082,
#48083,#48084,#48085),.UNSPECIFIED.,.F.,.F.,(4,1,1,1,1,4),(59.6902604182061,
60.1955726391529,61.1820335325579,62.1684944259629,63.154955319368,64.141416212773),
 .UNSPECIFIED.);
#1162=B_SPLINE_CURVE_WITH_KNOTS('',3,(#48088,#48089,#48090,#48091,#48092,
#48093,#48094,#48095,#48096),.UNSPECIFIED.,.F.,.F.,(4,1,1,1,1,1,4),(59.6902604182061,
59.775601223602,60.762062117007,61.748523010412,62.734983903817,63.721444797222,
64.6638825844085),.UNSPECIFIED.);
#1163=B_SPLINE_CURVE_WITH_KNOTS('',3,(#48101,#48102,#48103,#48104,#48105,
#48106,#48107,#48108,#48109,#48110),.UNSPECIFIED.,.F.,.F.,(4,1,1,1,1,1,
1,4),(53.4070751110265,54.2768072787229,55.2632681721279,56.2497290655329,
57.2361899589379,58.2226508523429,59.2091117457479,59.6902604182061),
 .UNSPECIFIED.);
#1164=B_SPLINE_CURVE_WITH_KNOTS('',3,(#48111,#48112,#48113,#48114,#48115,
#48116,#48117,#48118,#48119,#48120),.UNSPECIFIED.,.F.,.F.,(4,1,1,1,1,1,
1,4),(53.4070751110265,53.856835863172,54.843296756577,55.829757649982,
56.816218543387,57.802679436792,58.789140330197,59.6902604182061),
 .UNSPECIFIED.);
#1165=B_SPLINE_CURVE_WITH_KNOTS('',3,(#48125,#48126,#48127,#48128,#48129,
#48130,#48131,#48132,#48133,#48134,#48135),.UNSPECIFIED.,.F.,.F.,(4,1,1,
1,1,1,1,1,4),(47.1238898038469,47.3715810248879,48.3580419182929,49.3445028116979,
50.3309637051029,51.3174245985079,52.3038854919129,53.2903463853179,53.4070751110265),
 .UNSPECIFIED.);
#1166=B_SPLINE_CURVE_WITH_KNOTS('',3,(#48136,#48137,#48138,#48139,#48140,
#48141,#48142,#48143,#48144,#48145),.UNSPECIFIED.,.F.,.F.,(4,1,1,1,1,1,
1,4),(47.1238898038469,47.9380705027419,48.9245313961469,49.9109922895519,
50.897453182957,51.883914076362,52.870374969767,53.4070751110265),
 .UNSPECIFIED.);
#1167=B_SPLINE_CURVE_WITH_KNOTS('',3,(#48150,#48151,#48152,#48153,#48154,
#48155,#48156,#48157,#48158,#48159),.UNSPECIFIED.,.F.,.F.,(4,1,1,1,1,1,
1,4),(40.8407044966673,41.4528156644579,42.4392765578629,43.4257374512679,
44.4121983446729,45.3986592380779,46.3851201314829,47.1238898038469),
 .UNSPECIFIED.);
#1168=B_SPLINE_CURVE_WITH_KNOTS('',3,(#48160,#48161,#48162,#48163,#48164,
#48165,#48166,#48167,#48168,#48169,#48170),.UNSPECIFIED.,.F.,.F.,(4,1,1,
1,1,1,1,1,4),(40.8407044966673,41.0328442489069,42.0193051423119,43.0057660357169,
43.9922269291219,44.9786878225269,45.9651487159319,46.9516096093369,47.1238898038469),
 .UNSPECIFIED.);
#1169=B_SPLINE_CURVE_WITH_KNOTS('',3,(#48175,#48176,#48177,#48178,#48179,
#48180,#48181,#48182,#48183,#48184),.UNSPECIFIED.,.F.,.F.,(4,1,1,1,1,1,
1,4),(34.5575191894877,35.5340503040279,36.5205111974329,37.5069720908379,
38.4934329842429,39.4798938776479,40.4663547710529,40.8407044966673),
 .UNSPECIFIED.);
#1170=B_SPLINE_CURVE_WITH_KNOTS('',3,(#48185,#48186,#48187,#48188,#48189,
#48190,#48191,#48192,#48193,#48194),.UNSPECIFIED.,.F.,.F.,(4,1,1,1,1,1,
1,4),(34.5575191894877,35.1140788884769,36.1005397818819,37.0870006752869,
38.0734615686919,39.0599224620969,40.0463833555019,40.8407044966673),
 .UNSPECIFIED.);
#1171=B_SPLINE_CURVE_WITH_KNOTS('',3,(#48199,#48200,#48201,#48202,#48203,
#48204,#48205,#48206,#48207,#48208,#48209),.UNSPECIFIED.,.F.,.F.,(4,1,1,
1,1,1,1,1,4),(28.2743338823081,28.6288240501929,29.6152849435979,30.6017458370029,
31.5882067304079,32.5746676238129,33.5611285172179,34.5475894106229,34.5575191894877),
 .UNSPECIFIED.);
#1172=B_SPLINE_CURVE_WITH_KNOTS('',3,(#48210,#48211,#48212,#48213,#48214,
#48215,#48216,#48217,#48218,#48219),.UNSPECIFIED.,.F.,.F.,(4,1,1,1,1,1,
1,4),(28.2743338823081,29.1953135280469,30.1817744214519,31.1682353148569,
32.1546962082619,33.1411571016669,34.1276179950719,34.5575191894877),
 .UNSPECIFIED.);
#1173=B_SPLINE_CURVE_WITH_KNOTS('',3,(#48224,#48225,#48226,#48227,#48228,
#48229,#48230,#48231,#48232,#48233),.UNSPECIFIED.,.F.,.F.,(4,1,1,1,1,1,
1,4),(21.9911485751285,22.7100586897628,23.6965195831678,24.6829804765729,
25.6694413699779,26.6559022633829,27.6423631567879,28.2743338823081),
 .UNSPECIFIED.);
#1174=B_SPLINE_CURVE_WITH_KNOTS('',3,(#48234,#48235,#48236,#48237,#48238,
#48239,#48240,#48241,#48242,#48243,#48244),.UNSPECIFIED.,.F.,.F.,(4,1,1,
1,1,1,1,1,4),(21.9911485751285,22.2900872742119,23.2765481676169,24.2630090610219,
25.2494699544269,26.2359308478319,27.2223917412369,28.2088526346419,28.2743338823081),
 .UNSPECIFIED.);
#1175=B_SPLINE_CURVE_WITH_KNOTS('',3,(#48250,#48251,#48252,#48253,#48254),
 .UNSPECIFIED.,.F.,.F.,(4,1,4),(14.3984001269719,15.3848610203769,15.7079632679489),
 .UNSPECIFIED.);
#1176=B_SPLINE_CURVE_WITH_KNOTS('',3,(#48257,#48258,#48259,#48260,#48261),
 .UNSPECIFIED.,.F.,.F.,(4,1,4),(13.8759337553363,14.8183715425228,15.7079632679489),
 .UNSPECIFIED.);
#1177=B_SPLINE_CURVE_WITH_KNOTS('',3,(#48267,#48268,#48269,#48270),
 .UNSPECIFIED.,.F.,.F.,(4,4),(51.5750455984138,52.2824273504651),
 .UNSPECIFIED.);
#1178=B_SPLINE_CURVE_WITH_KNOTS('',3,(#48278,#48279,#48280,#48281,#48282,
#48283,#48284,#48285,#48286,#48287),.UNSPECIFIED.,.F.,.F.,(4,3,3,4),(-50.2654824574367,
-49.3230446702501,-48.3365837768451,-47.8312715558982),.UNSPECIFIED.);
#1179=B_SPLINE_CURVE_WITH_KNOTS('',3,(#48292,#48293,#48294,#48295,#48296,
#48297,#48298,#48299,#48300,#48301,#48302,#48303,#48304,#48305,#48306,#48307,
#48308,#48309,#48310,#48311,#48312,#48313,#48314,#48315,#48316),
 .UNSPECIFIED.,.F.,.F.,(4,3,3,3,3,3,3,3,4),(45.2918602912342,45.3772010966301,
46.3636619900351,47.3501228834401,48.3365837768451,49.3230446702501,50.3095055636551,
51.2959664570601,51.5750455984138),.UNSPECIFIED.);
#1180=B_SPLINE_CURVE_WITH_KNOTS('',3,(#48317,#48318,#48319,#48320,#48321,
#48322,#48323,#48324,#48325,#48326,#48327,#48328,#48329,#48330,#48331,#48332,
#48333,#48334,#48335,#48336,#48337,#48338),.UNSPECIFIED.,.F.,.F.,(4,3,3,
3,3,3,3,4),(-47.8312715558982,-47.3501228834401,-46.3636619900351,-45.3772010966301,
-44.3907402032251,-43.4042793098201,-42.4178184164151,-41.5480862487186),
 .UNSPECIFIED.);
#1181=B_SPLINE_CURVE_WITH_KNOTS('',3,(#48343,#48344,#48345,#48346,#48347,
#48348,#48349,#48350,#48351,#48352,#48353,#48354,#48355,#48356,#48357,#48358,
#48359,#48360,#48361,#48362,#48363,#48364),.UNSPECIFIED.,.F.,.F.,(4,3,3,
3,3,3,3,4),(39.0086749840546,39.4584357362001,40.4448966296051,41.4313575230101,
42.4178184164151,43.4042793098201,44.3907402032251,45.2918602912342),
 .UNSPECIFIED.);
#1182=B_SPLINE_CURVE_WITH_KNOTS('',3,(#48365,#48366,#48367,#48368,#48369,
#48370,#48371,#48372,#48373,#48374,#48375,#48376,#48377,#48378,#48379,#48380,
#48381,#48382,#48383,#48384,#48385,#48386,#48387,#48388,#48389),
 .UNSPECIFIED.,.F.,.F.,(4,3,3,3,3,3,3,3,4),(-41.5480862487186,-41.4313575230101,
-40.4448966296051,-39.4584357362001,-38.4719748427951,-37.4855139493901,
-36.4990530559851,-35.5125921625801,-35.2649009415391),.UNSPECIFIED.);
#1183=B_SPLINE_CURVE_WITH_KNOTS('',3,(#48394,#48395,#48396,#48397,#48398,
#48399,#48400,#48401,#48402,#48403,#48404,#48405,#48406,#48407,#48408,#48409,
#48410,#48411,#48412,#48413,#48414,#48415),.UNSPECIFIED.,.F.,.F.,(4,3,3,
3,3,3,3,4),(32.725489676875,33.5396703757701,34.5261312691751,35.5125921625801,
36.4990530559851,37.4855139493901,38.4719748427951,39.0086749840546),
 .UNSPECIFIED.);
#1184=B_SPLINE_CURVE_WITH_KNOTS('',3,(#48416,#48417,#48418,#48419,#48420,
#48421,#48422,#48423,#48424,#48425,#48426,#48427,#48428,#48429,#48430,#48431,
#48432,#48433,#48434,#48435,#48436,#48437),.UNSPECIFIED.,.F.,.F.,(4,3,3,
3,3,3,3,4),(-35.2649009415391,-34.5261312691751,-33.5396703757701,-32.5532094823651,
-31.5667485889601,-30.5802876955551,-29.5938268021501,-28.9817156343595),
 .UNSPECIFIED.);
#1185=B_SPLINE_CURVE_WITH_KNOTS('',3,(#48442,#48443,#48444,#48445,#48446,
#48447,#48448,#48449,#48450,#48451,#48452,#48453,#48454,#48455,#48456,#48457,
#48458,#48459,#48460,#48461,#48462,#48463,#48464,#48465,#48466),
 .UNSPECIFIED.,.F.,.F.,(4,3,3,3,3,3,3,3,4),(26.4423043696954,26.6344441219351,
27.6209050153401,28.6073659087451,29.5938268021501,30.5802876955551,31.5667485889601,
32.5532094823651,32.725489676875),.UNSPECIFIED.);
#1186=B_SPLINE_CURVE_WITH_KNOTS('',3,(#48467,#48468,#48469,#48470,#48471,
#48472,#48473,#48474,#48475,#48476,#48477,#48478,#48479,#48480,#48481,#48482,
#48483,#48484,#48485,#48486,#48487,#48488),.UNSPECIFIED.,.F.,.F.,(4,3,3,
3,3,3,3,4),(-28.9817156343595,-28.6073659087451,-27.6209050153401,-26.6344441219351,
-25.6479832285301,-24.6615223351251,-23.6750614417201,-22.6985303271799),
 .UNSPECIFIED.);
#1187=B_SPLINE_CURVE_WITH_KNOTS('',3,(#48493,#48494,#48495,#48496,#48497,
#48498,#48499,#48500,#48501,#48502,#48503,#48504,#48505,#48506,#48507,#48508,
#48509,#48510,#48511,#48512,#48513,#48514),.UNSPECIFIED.,.F.,.F.,(4,3,3,
3,3,3,3,4),(20.1591190625158,20.7156787615051,21.7021396549101,22.6886005483151,
23.6750614417201,24.6615223351251,25.6479832285301,26.4423043696954),
 .UNSPECIFIED.);
#1188=B_SPLINE_CURVE_WITH_KNOTS('',3,(#48515,#48516,#48517,#48518,#48519,
#48520,#48521,#48522,#48523,#48524,#48525,#48526,#48527,#48528,#48529,#48530,
#48531,#48532,#48533,#48534,#48535,#48536,#48537,#48538,#48539),
 .UNSPECIFIED.,.F.,.F.,(4,3,3,3,3,3,3,3,4),(-22.6985303271799,-22.6886005483151,
-21.7021396549101,-20.7156787615051,-19.7292178681001,-18.742756974695,
-17.75629608129,-16.769835187885,-16.4153450200003),.UNSPECIFIED.);
#1189=B_SPLINE_CURVE_WITH_KNOTS('',3,(#48544,#48545,#48546,#48547,#48548,
#48549,#48550,#48551,#48552,#48553,#48554,#48555,#48556,#48557,#48558,#48559,
#48560,#48561,#48562,#48563,#48564,#48565),.UNSPECIFIED.,.F.,.F.,(4,3,3,
3,3,3,3,4),(13.8759337553362,14.796913401075,15.78337429448,16.769835187885,
17.75629608129,18.7427569746951,19.7292178681001,20.1591190625158),
 .UNSPECIFIED.);
#1190=B_SPLINE_CURVE_WITH_KNOTS('',3,(#48566,#48567,#48568,#48569,#48570,
#48571,#48572,#48573,#48574,#48575,#48576,#48577,#48578,#48579,#48580,#48581,
#48582,#48583,#48584,#48585,#48586,#48587),.UNSPECIFIED.,.F.,.F.,(4,3,3,
3,3,3,3,4),(-16.4153450200003,-15.78337429448,-14.796913401075,-13.81045250767,
-12.823991614265,-11.83753072086,-10.851069827455,-10.1321597128207),
 .UNSPECIFIED.);
#1191=B_SPLINE_CURVE_WITH_KNOTS('',3,(#48593,#48594,#48595,#48596,#48597,
#48598,#48599,#48600,#48601,#48602,#48603,#48604,#48605),.UNSPECIFIED.,
 .F.,.F.,(4,3,3,3,4),(-3.84897440564113,-2.95938268021501,-1.97292178681001,
-0.986460893405003,0.),.UNSPECIFIED.);
#1192=B_SPLINE_CURVE_WITH_KNOTS('',3,(#48608,#48609,#48610,#48611,#48612,
#48613,#48614,#48615,#48616,#48617,#48618,#48619,#48620,#48621,#48622,#48623,
#48624,#48625,#48626),.UNSPECIFIED.,.F.,.F.,(4,3,3,3,3,3,4),(2.01694489302845,
2.95938268021501,3.94584357362001,4.93230446702502,5.91876536043002,6.90522625383502,
7.59274844815666),.UNSPECIFIED.);
#1193=B_SPLINE_CURVE_WITH_KNOTS('',3,(#48632,#48633,#48634,#48635,#48636,
#48637,#48638,#48639),.UNSPECIFIED.,.F.,.F.,(4,1,1,1,1,4),(59.6902604182061,
60.1955726391529,61.1820335325579,62.1684944259629,63.154955319368,64.141416212773),
 .UNSPECIFIED.);
#1194=B_SPLINE_CURVE_WITH_KNOTS('',3,(#48642,#48643,#48644,#48645,#48646,
#48647,#48648,#48649,#48650),.UNSPECIFIED.,.F.,.F.,(4,1,1,1,1,1,4),(59.6902604182061,
59.775601223602,60.762062117007,61.748523010412,62.734983903817,63.721444797222,
64.6638825844085),.UNSPECIFIED.);
#1195=B_SPLINE_CURVE_WITH_KNOTS('',3,(#48655,#48656,#48657,#48658,#48659,
#48660,#48661,#48662,#48663,#48664),.UNSPECIFIED.,.F.,.F.,(4,1,1,1,1,1,
1,4),(53.4070751110265,54.2768072787229,55.2632681721279,56.2497290655329,
57.2361899589379,58.2226508523429,59.2091117457479,59.6902604182061),
 .UNSPECIFIED.);
#1196=B_SPLINE_CURVE_WITH_KNOTS('',3,(#48665,#48666,#48667,#48668,#48669,
#48670,#48671,#48672,#48673,#48674),.UNSPECIFIED.,.F.,.F.,(4,1,1,1,1,1,
1,4),(53.4070751110265,53.856835863172,54.843296756577,55.829757649982,
56.816218543387,57.802679436792,58.789140330197,59.6902604182061),
 .UNSPECIFIED.);
#1197=B_SPLINE_CURVE_WITH_KNOTS('',3,(#48679,#48680,#48681,#48682,#48683,
#48684,#48685,#48686,#48687,#48688,#48689),.UNSPECIFIED.,.F.,.F.,(4,1,1,
1,1,1,1,1,4),(47.1238898038469,47.3715810248879,48.3580419182929,49.3445028116979,
50.3309637051029,51.3174245985079,52.3038854919129,53.2903463853179,53.4070751110265),
 .UNSPECIFIED.);
#1198=B_SPLINE_CURVE_WITH_KNOTS('',3,(#48690,#48691,#48692,#48693,#48694,
#48695,#48696,#48697,#48698,#48699),.UNSPECIFIED.,.F.,.F.,(4,1,1,1,1,1,
1,4),(47.1238898038469,47.9380705027419,48.9245313961469,49.9109922895519,
50.897453182957,51.883914076362,52.870374969767,53.4070751110265),
 .UNSPECIFIED.);
#1199=B_SPLINE_CURVE_WITH_KNOTS('',3,(#48704,#48705,#48706,#48707,#48708,
#48709,#48710,#48711,#48712,#48713),.UNSPECIFIED.,.F.,.F.,(4,1,1,1,1,1,
1,4),(40.8407044966673,41.4528156644579,42.4392765578629,43.4257374512679,
44.4121983446729,45.3986592380779,46.3851201314829,47.1238898038469),
 .UNSPECIFIED.);
#1200=B_SPLINE_CURVE_WITH_KNOTS('',3,(#48714,#48715,#48716,#48717,#48718,
#48719,#48720,#48721,#48722,#48723,#48724),.UNSPECIFIED.,.F.,.F.,(4,1,1,
1,1,1,1,1,4),(40.8407044966673,41.0328442489069,42.0193051423119,43.0057660357169,
43.9922269291219,44.9786878225269,45.9651487159319,46.9516096093369,47.1238898038469),
 .UNSPECIFIED.);
#1201=B_SPLINE_CURVE_WITH_KNOTS('',3,(#48729,#48730,#48731,#48732,#48733,
#48734,#48735,#48736,#48737,#48738),.UNSPECIFIED.,.F.,.F.,(4,1,1,1,1,1,
1,4),(34.5575191894877,35.5340503040279,36.5205111974329,37.5069720908379,
38.4934329842429,39.4798938776479,40.4663547710529,40.8407044966673),
 .UNSPECIFIED.);
#1202=B_SPLINE_CURVE_WITH_KNOTS('',3,(#48739,#48740,#48741,#48742,#48743,
#48744,#48745,#48746,#48747,#48748),.UNSPECIFIED.,.F.,.F.,(4,1,1,1,1,1,
1,4),(34.5575191894877,35.1140788884769,36.1005397818819,37.0870006752869,
38.0734615686919,39.0599224620969,40.0463833555019,40.8407044966673),
 .UNSPECIFIED.);
#1203=B_SPLINE_CURVE_WITH_KNOTS('',3,(#48753,#48754,#48755,#48756,#48757,
#48758,#48759,#48760,#48761,#48762,#48763),.UNSPECIFIED.,.F.,.F.,(4,1,1,
1,1,1,1,1,4),(28.2743338823081,28.6288240501929,29.6152849435979,30.6017458370029,
31.5882067304079,32.5746676238129,33.5611285172179,34.5475894106229,34.5575191894877),
 .UNSPECIFIED.);
#1204=B_SPLINE_CURVE_WITH_KNOTS('',3,(#48764,#48765,#48766,#48767,#48768,
#48769,#48770,#48771,#48772,#48773),.UNSPECIFIED.,.F.,.F.,(4,1,1,1,1,1,
1,4),(28.2743338823081,29.1953135280469,30.1817744214519,31.1682353148569,
32.1546962082619,33.1411571016669,34.1276179950719,34.5575191894877),
 .UNSPECIFIED.);
#1205=B_SPLINE_CURVE_WITH_KNOTS('',3,(#48778,#48779,#48780,#48781,#48782,
#48783,#48784,#48785,#48786,#48787),.UNSPECIFIED.,.F.,.F.,(4,1,1,1,1,1,
1,4),(21.9911485751285,22.7100586897628,23.6965195831678,24.6829804765729,
25.6694413699779,26.6559022633829,27.6423631567879,28.2743338823081),
 .UNSPECIFIED.);
#1206=B_SPLINE_CURVE_WITH_KNOTS('',3,(#48788,#48789,#48790,#48791,#48792,
#48793,#48794,#48795,#48796,#48797,#48798),.UNSPECIFIED.,.F.,.F.,(4,1,1,
1,1,1,1,1,4),(21.9911485751285,22.2900872742119,23.2765481676169,24.2630090610219,
25.2494699544269,26.2359308478319,27.2223917412369,28.2088526346419,28.2743338823081),
 .UNSPECIFIED.);
#1207=B_SPLINE_CURVE_WITH_KNOTS('',3,(#48804,#48805,#48806,#48807,#48808),
 .UNSPECIFIED.,.F.,.F.,(4,1,4),(14.3984001269719,15.3848610203769,15.7079632679489),
 .UNSPECIFIED.);
#1208=B_SPLINE_CURVE_WITH_KNOTS('',3,(#48811,#48812,#48813,#48814,#48815),
 .UNSPECIFIED.,.F.,.F.,(4,1,4),(13.8759337553363,14.8183715425228,15.7079632679489),
 .UNSPECIFIED.);
#1209=B_SPLINE_CURVE_WITH_KNOTS('',3,(#48817,#48818,#48819,#48820,#48821,
#48822,#48823,#48824,#48825,#48826,#48827,#48828,#48829,#48830,#48831,#48832,
#48833,#48834,#48835,#48836,#48837,#48838,#48839,#48840,#48841,#48842,#48843,
#48844,#48845,#48846,#48847,#48848,#48849,#48850,#48851,#48852,#48853,#48854,
#48855,#48856,#48857,#48858,#48859,#48860,#48861,#48862,#48863,#48864,#48865,
#48866,#48867,#48868,#48869,#48870,#48871,#48872,#48873,#48874,#48875,#48876,
#48877,#48878,#48879,#48880,#48881,#48882,#48883,#48884,#48885,#48886,#48887,
#48888,#48889,#48890,#48891,#48892,#48893,#48894,#48895,#48896,#48897,#48898,
#48899,#48900,#48901,#48902,#48903,#48904,#48905,#48906,#48907,#48908,#48909,
#48910),.UNSPECIFIED.,.F.,.F.,(4,3,3,3,3,3,3,3,3,3,3,3,3,3,3,3,3,3,3,3,
3,3,3,3,3,3,3,3,3,3,3,4),(-0.569248610399453,-0.543562558043411,-0.517250584660783,
-0.510351573265488,-0.504796629765234,-0.477730613871864,-0.456104856148543,
-0.448985761186696,-0.442526474182097,-0.414793258161359,-0.386635508597981,
-0.358697135593994,-0.34520398971682,-0.340863862860947,-0.336326730527656,
-0.307401056922635,-0.304724552085299,-0.276937944371136,-0.248514561286397,
-0.23265772508323,-0.228221590562879,-0.199230787763733,-0.169668272024871,
-0.139872989252767,-0.12408548320274,-0.117715318700335,-0.113354339820942,
-0.0828129568830819,-0.0522455401301121,-0.022270235741096,-0.0135729408525504,
0.),.UNSPECIFIED.);
#1210=B_SPLINE_CURVE_WITH_KNOTS('',3,(#48911,#48912,#48913,#48914,#48915,
#48916,#48917,#48918,#48919,#48920,#48921,#48922,#48923,#48924,#48925,#48926,
#48927,#48928,#48929,#48930,#48931,#48932,#48933,#48934,#48935,#48936,#48937,
#48938,#48939,#48940,#48941,#48942,#48943,#48944,#48945,#48946,#48947,#48948,
#48949,#48950,#48951,#48952,#48953,#48954,#48955,#48956,#48957,#48958,#48959,
#48960,#48961,#48962,#48963,#48964,#48965,#48966,#48967,#48968,#48969,#48970,
#48971,#48972,#48973,#48974,#48975,#48976,#48977,#48978,#48979,#48980,#48981,
#48982,#48983,#48984,#48985,#48986,#48987,#48988,#48989,#48990,#48991,#48992,
#48993,#48994,#48995,#48996,#48997,#48998,#48999,#49000,#49001,#49002,#49003,
#49004,#49005,#49006,#49007),.UNSPECIFIED.,.F.,.F.,(4,3,3,3,3,3,3,3,3,3,
3,3,3,3,3,3,3,3,3,3,3,3,3,3,3,3,3,3,3,3,3,3,4),(-0.566847306048093,-0.536658716403432,
-0.50605373953314,-0.497358803993733,-0.490469668716376,-0.460327091817824,
-0.43729948162817,-0.425273577512184,-0.420376587364543,-0.390957251202536,
-0.362079079161669,-0.333750895422636,-0.319339724142124,-0.312267998605923,
-0.308232630749578,-0.280241862158672,-0.276106210300586,-0.247648696044962,
-0.218090837421661,-0.209492455589693,-0.204737921056362,-0.200614185310069,
-0.172780910553805,-0.145025994944757,-0.117750394973387,-0.104429823984033,
-0.100024823328952,-0.0958388020470428,-0.0691739371857627,-0.0429558817167698,
-0.017514133983365,-0.0111858270585532,0.),.UNSPECIFIED.);
#1211=B_SPLINE_CURVE_WITH_KNOTS('',3,(#49009,#49010,#49011,#49012,#49013,
#49014,#49015,#49016,#49017,#49018,#49019),.UNSPECIFIED.,.F.,.F.,(4,1,1,
1,1,1,1,1,4),(15.7079632679489,15.8048324359278,16.7912933293328,17.7777542227378,
18.7642151161428,19.7506760095478,20.7371369029528,21.7235977963578,21.9911485751285),
 .UNSPECIFIED.);
#1212=B_SPLINE_CURVE_WITH_KNOTS('',3,(#49020,#49021,#49022,#49023,#49024,
#49025,#49026,#49027,#49028,#49029),.UNSPECIFIED.,.F.,.F.,(4,1,1,1,1,1,
1,4),(15.7079632679489,16.3713219137819,17.3577828071869,18.3442437005919,
19.3307045939969,20.3171654874019,21.3036263808069,21.9911485751285),
 .UNSPECIFIED.);
#1213=B_SPLINE_CURVE_WITH_KNOTS('',3,(#49254,#49255,#49256,#49257,#49258,
#49259,#49260,#49261,#49262,#49263,#49264,#49265,#49266,#49267,#49268,#49269,
#49270,#49271,#49272,#49273,#49274,#49275,#49276,#49277,#49278,#49279,#49280,
#49281,#49282,#49283,#49284,#49285,#49286,#49287,#49288,#49289,#49290,#49291,
#49292,#49293,#49294,#49295,#49296,#49297,#49298,#49299,#49300,#49301,#49302,
#49303,#49304,#49305,#49306,#49307,#49308,#49309,#49310,#49311,#49312,#49313,
#49314,#49315,#49316,#49317,#49318,#49319,#49320,#49321,#49322,#49323,#49324,
#49325,#49326,#49327,#49328,#49329,#49330,#49331,#49332,#49333,#49334,#49335,
#49336,#49337,#49338,#49339,#49340,#49341,#49342,#49343,#49344),
 .UNSPECIFIED.,.F.,.F.,(4,3,3,3,3,3,3,3,3,3,3,3,3,3,3,3,3,3,3,3,3,3,3,3,
3,3,3,3,3,3,4),(0.,0.0253755398454445,0.0514213153132464,0.077957584539944,
0.0899764747654525,0.096803871475702,0.102648438541228,0.129953427359202,
0.157705320199216,0.184206857431119,0.195897861719558,0.201348082731475,
0.206600886453667,0.235230947526492,0.263711469126827,0.291580359310597,
0.307939787194046,0.312151069047901,0.340175334720984,0.369258031218753,
0.398694002185391,0.41802365259294,0.423204309536776,0.428148753834381,
0.459444366737233,0.482916076414372,0.491343338637999,0.498388095452059,
0.528903290158942,0.553331205445788,0.566847306048063),.UNSPECIFIED.);
#1214=B_SPLINE_CURVE_WITH_KNOTS('',3,(#49345,#49346,#49347,#49348,#49349,
#49350,#49351,#49352,#49353,#49354,#49355,#49356,#49357,#49358,#49359,#49360,
#49361,#49362,#49363,#49364,#49365,#49366,#49367,#49368,#49369),
 .UNSPECIFIED.,.F.,.F.,(4,3,3,3,3,3,3,3,4),(-10.1321597128207,-9.86460893405002,
-8.87814804064502,-7.89168714724002,-6.90522625383502,-5.91876536043002,
-4.93230446702501,-3.94584357362001,-3.84897440564113),.UNSPECIFIED.);
#1215=B_SPLINE_CURVE_WITH_KNOTS('',3,(#49594,#49595,#49596,#49597,#49598,
#49599,#49600,#49601,#49602,#49603,#49604,#49605,#49606,#49607,#49608,#49609,
#49610,#49611,#49612,#49613,#49614,#49615,#49616,#49617,#49618),
 .UNSPECIFIED.,.F.,.F.,(4,3,3,3,3,3,3,3,4),(7.59274844815666,7.89168714724002,
8.87814804064503,9.86460893405003,10.851069827455,11.83753072086,12.823991614265,
13.81045250767,13.8759337553362),.UNSPECIFIED.);
#1216=B_SPLINE_CURVE_WITH_KNOTS('',3,(#49619,#49620,#49621,#49622,#49623,
#49624,#49625,#49626,#49627,#49628,#49629,#49630,#49631,#49632,#49633,#49634,
#49635,#49636,#49637,#49638,#49639,#49640,#49641,#49642,#49643,#49644,#49645,
#49646,#49647,#49648,#49649,#49650,#49651,#49652,#49653,#49654,#49655,#49656,
#49657,#49658,#49659,#49660,#49661,#49662,#49663,#49664,#49665,#49666,#49667,
#49668,#49669,#49670,#49671,#49672,#49673,#49674,#49675,#49676,#49677,#49678,
#49679,#49680,#49681,#49682,#49683,#49684,#49685,#49686,#49687,#49688,#49689,
#49690,#49691,#49692,#49693,#49694,#49695,#49696,#49697,#49698,#49699,#49700,
#49701,#49702,#49703,#49704,#49705,#49706),.UNSPECIFIED.,.F.,.F.,(4,3,3,
3,3,3,3,3,3,3,3,3,3,3,3,3,3,3,3,3,3,3,3,3,3,3,3,3,3,4),(0.,0.0297349244535721,
0.060121569348429,0.0891410162773849,0.114533032340221,0.120626667476319,
0.15038169425931,0.17997017941563,0.208046920756741,0.230390549968388,0.234466744960236,
0.263371944870156,0.292277144780076,0.321216417936983,0.336017031727334,
0.340284462229876,0.344592011030409,0.372696707961539,0.400818636707195,
0.428516289762568,0.439576354164994,0.44540318305,0.450327524863458,0.477288294894219,
0.497472780816313,0.505235740104314,0.511959381000542,0.537907915849272,
0.558026238582596,0.569248610399449),.UNSPECIFIED.);
#1217=B_SPLINE_CURVE_WITH_KNOTS('',3,(#49709,#49710,#49711,#49712,#49713,
#49714,#49715,#49716,#49717,#49718,#49719,#49720,#49721,#49722,#49723,#49724,
#49725,#49726,#49727,#49728,#49729,#49730,#49731,#49732,#49733,#49734,#49735,
#49736,#49737,#49738,#49739,#49740,#49741,#49742,#49743,#49744,#49745,#49746,
#49747,#49748,#49749,#49750,#49751,#49752,#49753,#49754,#49755,#49756,#49757,
#49758,#49759,#49760,#49761,#49762,#49763,#49764,#49765,#49766,#49767,#49768,
#49769,#49770,#49771,#49772,#49773,#49774,#49775,#49776,#49777,#49778,#49779,
#49780,#49781,#49782,#49783,#49784,#49785,#49786,#49787,#49788,#49789,#49790,
#49791,#49792,#49793,#49794,#49795,#49796,#49797,#49798,#49799,#49800,#49801,
#49802),.UNSPECIFIED.,.F.,.F.,(4,3,3,3,3,3,3,3,3,3,3,3,3,3,3,3,3,3,3,3,
3,3,3,3,3,3,3,3,3,3,3,4),(-0.569248610399449,-0.543563182261633,-0.517251726319563,
-0.510354426439678,-0.50479695498386,-0.477731372271303,-0.456105519748053,
-0.448988869091777,-0.442526350881559,-0.414793531524841,-0.386635753667763,
-0.358697146614525,-0.34520399798222,-0.340863870845798,-0.33632674866549,
-0.307401034118885,-0.304724552085303,-0.276937498904782,-0.248513836066906,
-0.232656079580101,-0.228221193819419,-0.199230039362694,-0.1696673522492,
-0.139872047864531,-0.124084659488033,-0.117720027272243,-0.113355233265148,
-0.0828137979174933,-0.0522463837565239,-0.0222709947806455,-0.0135729408525504,
0.),.UNSPECIFIED.);
#1218=B_SPLINE_CURVE_WITH_KNOTS('',3,(#49803,#49804,#49805,#49806,#49807,
#49808,#49809,#49810,#49811,#49812,#49813,#49814,#49815,#49816,#49817,#49818,
#49819,#49820,#49821,#49822,#49823,#49824,#49825,#49826,#49827,#49828,#49829,
#49830,#49831,#49832,#49833,#49834,#49835,#49836,#49837,#49838,#49839,#49840,
#49841,#49842,#49843,#49844,#49845,#49846,#49847,#49848,#49849,#49850,#49851,
#49852,#49853,#49854,#49855,#49856,#49857,#49858,#49859,#49860,#49861,#49862,
#49863,#49864,#49865,#49866,#49867,#49868,#49869,#49870,#49871,#49872,#49873,
#49874,#49875,#49876,#49877,#49878,#49879,#49880,#49881,#49882,#49883,#49884,
#49885,#49886,#49887,#49888,#49889,#49890,#49891,#49892,#49893,#49894,#49895,
#49896,#49897,#49898,#49899),.UNSPECIFIED.,.F.,.F.,(4,3,3,3,3,3,3,3,3,3,
3,3,3,3,3,3,3,3,3,3,3,3,3,3,3,3,3,3,3,3,3,3,4),(-0.566847306048093,-0.536659041927388,
-0.506054142756331,-0.497359284644658,-0.490469768799004,-0.460327170439997,
-0.43729955042257,-0.425273732599625,-0.420376646332479,-0.390957260247852,
-0.362078935948881,-0.333750632250775,-0.319339526763226,-0.312267682102884,
-0.308232073167884,-0.280241164390834,-0.276106210300581,-0.247648676940529,
-0.218090820705282,-0.209492305755956,-0.204738428044034,-0.200614618605046,
-0.172781361973988,-0.145026407762726,-0.11775064123255,-0.1044300394608,
-0.100025210256123,-0.0958388268874492,-0.0691738559200647,-0.0429555864020897,
-0.0175134923892686,-0.011185827058555,0.),.UNSPECIFIED.);
#1219=B_SPLINE_CURVE_WITH_KNOTS('',3,(#49901,#49902,#49903,#49904,#49905,
#49906,#49907,#49908,#49909,#49910,#49911),.UNSPECIFIED.,.F.,.F.,(4,1,1,
1,1,1,1,1,4),(15.7079632679489,15.8048324359278,16.7912933293328,17.7777542227378,
18.7642151161428,19.7506760095478,20.7371369029528,21.7235977963578,21.9911485751285),
 .UNSPECIFIED.);
#1220=B_SPLINE_CURVE_WITH_KNOTS('',3,(#49912,#49913,#49914,#49915,#49916,
#49917,#49918,#49919,#49920,#49921),.UNSPECIFIED.,.F.,.F.,(4,1,1,1,1,1,
1,4),(15.7079632679489,16.3713219137819,17.3577828071869,18.3442437005919,
19.3307045939969,20.3171654874019,21.3036263808069,21.9911485751285),
 .UNSPECIFIED.);
#1221=B_SPLINE_CURVE_WITH_KNOTS('',3,(#50146,#50147,#50148,#50149,#50150,
#50151,#50152,#50153,#50154,#50155,#50156,#50157,#50158,#50159,#50160,#50161,
#50162,#50163,#50164,#50165,#50166,#50167,#50168,#50169,#50170,#50171,#50172,
#50173,#50174,#50175,#50176,#50177,#50178,#50179,#50180,#50181,#50182,#50183,
#50184,#50185,#50186,#50187,#50188,#50189,#50190,#50191,#50192,#50193,#50194,
#50195,#50196,#50197,#50198,#50199,#50200,#50201,#50202,#50203,#50204,#50205,
#50206,#50207,#50208,#50209,#50210,#50211,#50212,#50213,#50214,#50215,#50216,
#50217,#50218,#50219,#50220,#50221,#50222,#50223,#50224,#50225,#50226,#50227,
#50228,#50229,#50230,#50231,#50232,#50233,#50234,#50235,#50236),
 .UNSPECIFIED.,.F.,.F.,(4,3,3,3,3,3,3,3,3,3,3,3,3,3,3,3,3,3,3,3,3,3,3,3,
3,3,3,3,3,3,4),(0.,0.0253750087516075,0.0514203072172438,0.0779567024559424,
0.0899762332180016,0.0968038780381036,0.10264843024679,0.129953053284425,
0.157704773943122,0.18420644773905,0.195897666391424,0.201348497446843,
0.206600974226724,0.235231090538335,0.263711469126833,0.291580637154729,
0.307940047672921,0.312151253621455,0.340175922185425,0.369258810210864,
0.398694834915773,0.418024381232026,0.42320553295956,0.428148997028943,
0.459444549133158,0.482916213211318,0.491343671374895,0.498388182075807,
0.528903373982295,0.5533312054458,0.566847306048075),.UNSPECIFIED.);
#1222=B_SPLINE_CURVE_WITH_KNOTS('',3,(#50237,#50238,#50239,#50240,#50241,
#50242,#50243,#50244,#50245,#50246,#50247,#50248,#50249,#50250,#50251,#50252,
#50253,#50254,#50255,#50256,#50257,#50258,#50259,#50260,#50261),
 .UNSPECIFIED.,.F.,.F.,(4,3,3,3,3,3,3,3,4),(-10.1321597128207,-9.86460893405002,
-8.87814804064502,-7.89168714724002,-6.90522625383502,-5.91876536043002,
-4.93230446702501,-3.94584357362001,-3.84897440564113),.UNSPECIFIED.);
#1223=B_SPLINE_CURVE_WITH_KNOTS('',3,(#50486,#50487,#50488,#50489,#50490,
#50491,#50492,#50493,#50494,#50495,#50496,#50497,#50498,#50499,#50500,#50501,
#50502,#50503,#50504,#50505,#50506,#50507,#50508,#50509,#50510),
 .UNSPECIFIED.,.F.,.F.,(4,3,3,3,3,3,3,3,4),(7.59274844815666,7.89168714724002,
8.87814804064502,9.86460893405003,10.851069827455,11.83753072086,12.823991614265,
13.81045250767,13.8759337553362),.UNSPECIFIED.);
#1224=B_SPLINE_CURVE_WITH_KNOTS('',3,(#50511,#50512,#50513,#50514,#50515,
#50516,#50517,#50518,#50519,#50520,#50521,#50522,#50523,#50524,#50525,#50526,
#50527,#50528,#50529,#50530,#50531,#50532,#50533,#50534,#50535,#50536,#50537,
#50538,#50539,#50540,#50541,#50542,#50543,#50544,#50545,#50546,#50547,#50548,
#50549,#50550,#50551,#50552,#50553,#50554,#50555,#50556,#50557,#50558,#50559,
#50560,#50561,#50562,#50563,#50564,#50565,#50566,#50567,#50568,#50569,#50570,
#50571,#50572,#50573,#50574,#50575,#50576,#50577,#50578,#50579,#50580,#50581,
#50582,#50583,#50584,#50585,#50586,#50587,#50588,#50589,#50590,#50591,#50592,
#50593,#50594,#50595,#50596,#50597,#50598),.UNSPECIFIED.,.F.,.F.,(4,3,3,
3,3,3,3,3,3,3,3,3,3,3,3,3,3,3,3,3,3,3,3,3,3,3,3,3,3,4),(0.,0.0297343797035864,
0.060120761877283,0.0891403097401323,0.114532414120125,0.120626668186271,
0.150381698992516,0.17997034368319,0.208047043957412,0.230390900373193,
0.234467387186734,0.263372265983406,0.292277144780078,0.32121640004702,
0.336017014955494,0.340284508571086,0.34459204647613,0.372696730262498,
0.400818675119593,0.428516484798209,0.439577058767134,0.445404835481582,
0.450327801888399,0.477288765031749,0.497473133419461,0.505236404100872,
0.511959471749983,0.53790833305976,0.558026238582597,0.56924861039945),
 .UNSPECIFIED.);
#1225=B_SPLINE_CURVE_WITH_KNOTS('',3,(#50601,#50602,#50603,#50604,#50605,
#50606,#50607,#50608,#50609,#50610,#50611,#50612,#50613,#50614,#50615,#50616,
#50617,#50618,#50619,#50620,#50621,#50622,#50623,#50624,#50625,#50626,#50627,
#50628,#50629,#50630,#50631,#50632,#50633,#50634,#50635,#50636,#50637,#50638,
#50639,#50640,#50641,#50642,#50643,#50644,#50645,#50646,#50647,#50648,#50649,
#50650,#50651,#50652,#50653,#50654,#50655,#50656,#50657,#50658,#50659,#50660,
#50661,#50662,#50663,#50664,#50665,#50666,#50667,#50668,#50669,#50670,#50671,
#50672,#50673,#50674,#50675,#50676,#50677,#50678,#50679,#50680,#50681,#50682,
#50683,#50684,#50685,#50686,#50687,#50688,#50689,#50690,#50691,#50692,#50693,
#50694),.UNSPECIFIED.,.F.,.F.,(4,3,3,3,3,3,3,3,3,3,3,3,3,3,3,3,3,3,3,3,
3,3,3,3,3,3,3,3,3,3,3,4),(-0.569248610399439,-0.54356321026788,-0.51725177755219,
-0.510354554433286,-0.504796969238609,-0.477731405971173,-0.456105549235436,
-0.448989007169752,-0.44252634525638,-0.41479354371395,-0.386635764628684,
-0.358697147124577,-0.345203998364752,-0.340863871144016,-0.336326749475397,
-0.307401033120815,-0.304724552085278,-0.27693747898326,-0.248513803621531,
-0.232656005969356,-0.228221175977861,-0.199230005786307,-0.169667310992576,
-0.139872005633123,-0.124084622535551,-0.117720237608985,-0.113355273030534,
-0.0828138353231538,-0.052246421283799,-0.0222710285652406,-0.0135729408525455,
0.),.UNSPECIFIED.);
#1226=B_SPLINE_CURVE_WITH_KNOTS('',3,(#50695,#50696,#50697,#50698,#50699,
#50700,#50701,#50702,#50703,#50704,#50705,#50706,#50707,#50708,#50709,#50710,
#50711,#50712,#50713,#50714,#50715,#50716,#50717,#50718,#50719,#50720,#50721,
#50722,#50723,#50724,#50725,#50726,#50727,#50728,#50729,#50730,#50731,#50732,
#50733,#50734,#50735,#50736,#50737,#50738,#50739,#50740,#50741,#50742,#50743,
#50744,#50745,#50746,#50747,#50748,#50749,#50750,#50751,#50752,#50753,#50754,
#50755,#50756,#50757,#50758,#50759,#50760,#50761,#50762,#50763,#50764,#50765,
#50766,#50767,#50768,#50769,#50770,#50771,#50772,#50773,#50774,#50775,#50776,
#50777,#50778,#50779,#50780,#50781,#50782,#50783,#50784,#50785,#50786,#50787,
#50788,#50789,#50790,#50791),.UNSPECIFIED.,.F.,.F.,(4,3,3,3,3,3,3,3,3,3,
3,3,3,3,3,3,3,3,3,3,3,3,3,3,3,3,3,3,3,3,3,3,4),(-0.566847306048084,-0.536659061903649,
-0.506054167513983,-0.49735931415594,-0.490469774907708,-0.46032717525434,
-0.437299554635119,-0.425273742105126,-0.42037664994689,-0.390957260822939,
-0.362078927205336,-0.333750616169337,-0.319339514702147,-0.312267662800037,
-0.308232039095118,-0.280241121737425,-0.276106210300576,-0.247648675773662,
-0.218090819684273,-0.209492296602851,-0.204738459070877,-0.200614645085577,
-0.172781389578512,-0.145026433045361,-0.117750656382618,-0.10443005271711,
-0.100025234036307,-0.0958388284225397,-0.0691738510173895,-0.0429555684736812,
-0.0175134533592336,-0.0111858270585534,0.),.UNSPECIFIED.);
#1227=B_SPLINE_CURVE_WITH_KNOTS('',3,(#50793,#50794,#50795,#50796,#50797,
#50798,#50799,#50800,#50801,#50802,#50803),.UNSPECIFIED.,.F.,.F.,(4,1,1,
1,1,1,1,1,4),(15.7079632679489,15.8048324359278,16.7912933293328,17.7777542227378,
18.7642151161429,19.7506760095479,20.7371369029529,21.7235977963579,21.9911485751285),
 .UNSPECIFIED.);
#1228=B_SPLINE_CURVE_WITH_KNOTS('',3,(#50804,#50805,#50806,#50807,#50808,
#50809,#50810,#50811,#50812,#50813),.UNSPECIFIED.,.F.,.F.,(4,1,1,1,1,1,
1,4),(15.7079632679489,16.3713219137819,17.3577828071869,18.3442437005919,
19.3307045939969,20.3171654874019,21.3036263808069,21.9911485751285),
 .UNSPECIFIED.);
#1229=B_SPLINE_CURVE_WITH_KNOTS('',3,(#51038,#51039,#51040,#51041,#51042,
#51043,#51044,#51045,#51046,#51047,#51048,#51049,#51050,#51051,#51052,#51053,
#51054,#51055,#51056,#51057,#51058,#51059,#51060,#51061,#51062,#51063,#51064,
#51065,#51066,#51067,#51068,#51069,#51070,#51071,#51072,#51073,#51074,#51075,
#51076,#51077,#51078,#51079,#51080,#51081,#51082,#51083,#51084,#51085,#51086,
#51087,#51088,#51089,#51090,#51091,#51092,#51093,#51094,#51095,#51096,#51097,
#51098,#51099,#51100,#51101,#51102,#51103,#51104,#51105,#51106,#51107,#51108,
#51109,#51110,#51111,#51112,#51113,#51114,#51115,#51116,#51117,#51118,#51119,
#51120,#51121,#51122,#51123,#51124,#51125,#51126,#51127,#51128),
 .UNSPECIFIED.,.F.,.F.,(4,3,3,3,3,3,3,3,3,3,3,3,3,3,3,3,3,3,3,3,3,3,3,3,
3,3,3,3,3,3,4),(0.,0.0253749761808373,0.0514202453857712,0.0779566483534038,
0.0899762183904566,0.0968038784409555,0.102648429733812,0.129953030321501,
0.157704740391969,0.184206422575685,0.195897654370316,0.20134852299372,
0.206600979641336,0.235231099301492,0.263711469126832,0.291580654157613,
0.307940063613124,0.312151264914525,0.340175958120619,0.369258857874792,
0.398694885878799,0.418024425824675,0.423205607838508,0.428149011920458,
0.459444560301794,0.482916221587795,0.491343691753009,0.498388187388185,
0.528903379110968,0.553331205445801,0.566847306048077),.UNSPECIFIED.);
#1230=B_SPLINE_CURVE_WITH_KNOTS('',3,(#51129,#51130,#51131,#51132,#51133,
#51134,#51135,#51136,#51137,#51138,#51139,#51140,#51141,#51142,#51143,#51144,
#51145,#51146,#51147,#51148,#51149,#51150,#51151,#51152,#51153),
 .UNSPECIFIED.,.F.,.F.,(4,3,3,3,3,3,3,3,4),(-10.1321597128207,-9.86460893405003,
-8.87814804064503,-7.89168714724002,-6.90522625383502,-5.91876536043002,
-4.93230446702501,-3.94584357362001,-3.84897440564112),.UNSPECIFIED.);
#1231=B_SPLINE_CURVE_WITH_KNOTS('',3,(#51378,#51379,#51380,#51381,#51382,
#51383,#51384,#51385,#51386,#51387,#51388,#51389,#51390,#51391,#51392,#51393,
#51394,#51395,#51396,#51397,#51398,#51399,#51400,#51401,#51402),
 .UNSPECIFIED.,.F.,.F.,(4,3,3,3,3,3,3,3,4),(7.59274844815664,7.89168714724002,
8.87814804064502,9.86460893405003,10.851069827455,11.83753072086,12.823991614265,
13.81045250767,13.8759337553362),.UNSPECIFIED.);
#1232=B_SPLINE_CURVE_WITH_KNOTS('',3,(#51403,#51404,#51405,#51406,#51407,
#51408,#51409,#51410,#51411,#51412,#51413,#51414,#51415,#51416,#51417,#51418,
#51419,#51420,#51421,#51422,#51423,#51424,#51425,#51426,#51427,#51428,#51429,
#51430,#51431,#51432,#51433,#51434,#51435,#51436,#51437,#51438,#51439,#51440,
#51441,#51442,#51443,#51444,#51445,#51446,#51447,#51448,#51449,#51450,#51451,
#51452,#51453,#51454,#51455,#51456,#51457,#51458,#51459,#51460,#51461,#51462,
#51463,#51464,#51465,#51466,#51467,#51468,#51469,#51470,#51471,#51472,#51473,
#51474,#51475,#51476,#51477,#51478,#51479,#51480,#51481,#51482,#51483,#51484,
#51485,#51486,#51487,#51488,#51489,#51490),.UNSPECIFIED.,.F.,.F.,(4,3,3,
3,3,3,3,3,3,3,3,3,3,3,3,3,3,3,3,3,3,3,3,3,3,3,3,3,3,4),(0.,0.0297343552567438,
0.0601207256243431,0.0891402780188099,0.114532386363968,0.120626668225237,
0.150381699187288,0.179970351010139,0.208047049452624,0.230390915983779,
0.234467415790057,0.263372280285067,0.292277144780078,0.321216399233671,
0.336017014192979,0.340284510578769,0.344592048040137,0.372696731227283,
0.400818676768978,0.428516493390579,0.439577089903316,0.445404908685826,
0.450327814198675,0.477288785913009,0.497473149080406,0.505236433644848,
0.511959475796908,0.537908351627998,0.558026238582596,0.569248610399449),
 .UNSPECIFIED.);
#1938=CYLINDRICAL_SURFACE('',#15146,2.5175);
#1939=CYLINDRICAL_SURFACE('',#15150,2.5175);
#1940=CYLINDRICAL_SURFACE('',#15151,2.5175);
#1941=CYLINDRICAL_SURFACE('',#15152,2.5175);
#1942=CYLINDRICAL_SURFACE('',#15153,2.5175);
#1943=CYLINDRICAL_SURFACE('',#15154,2.5175);
#1944=CYLINDRICAL_SURFACE('',#15155,2.5175);
#1945=CYLINDRICAL_SURFACE('',#15156,2.5175);
#1946=CYLINDRICAL_SURFACE('',#15158,3.0735);
#1947=CYLINDRICAL_SURFACE('',#15160,3.0735);
#1948=CYLINDRICAL_SURFACE('',#15161,3.0735);
#1949=CYLINDRICAL_SURFACE('',#15162,3.0735);
#1950=CYLINDRICAL_SURFACE('',#15163,3.0735);
#1951=CYLINDRICAL_SURFACE('',#15164,3.0735);
#1952=CYLINDRICAL_SURFACE('',#15165,3.0735);
#1953=CYLINDRICAL_SURFACE('',#15166,3.0735);
#1954=CYLINDRICAL_SURFACE('',#15168,2.5175);
#1955=CYLINDRICAL_SURFACE('',#15172,2.5175);
#1956=CYLINDRICAL_SURFACE('',#15173,2.5175);
#1957=CYLINDRICAL_SURFACE('',#15174,2.5175);
#1958=CYLINDRICAL_SURFACE('',#15175,2.5175);
#1959=CYLINDRICAL_SURFACE('',#15176,2.5175);
#1960=CYLINDRICAL_SURFACE('',#15177,2.5175);
#1961=CYLINDRICAL_SURFACE('',#15178,2.5175);
#1962=CYLINDRICAL_SURFACE('',#15180,3.0735);
#1963=CYLINDRICAL_SURFACE('',#15182,3.0735);
#1964=CYLINDRICAL_SURFACE('',#15183,3.0735);
#1965=CYLINDRICAL_SURFACE('',#15184,3.0735);
#1966=CYLINDRICAL_SURFACE('',#15185,3.0735);
#1967=CYLINDRICAL_SURFACE('',#15186,3.0735);
#1968=CYLINDRICAL_SURFACE('',#15187,3.0735);
#1969=CYLINDRICAL_SURFACE('',#15188,3.0735);
#1970=CYLINDRICAL_SURFACE('',#15190,2.5175);
#1971=CYLINDRICAL_SURFACE('',#15194,2.5175);
#1972=CYLINDRICAL_SURFACE('',#15195,2.5175);
#1973=CYLINDRICAL_SURFACE('',#15196,2.5175);
#1974=CYLINDRICAL_SURFACE('',#15197,2.5175);
#1975=CYLINDRICAL_SURFACE('',#15198,2.5175);
#1976=CYLINDRICAL_SURFACE('',#15199,2.5175);
#1977=CYLINDRICAL_SURFACE('',#15200,2.5175);
#1978=CYLINDRICAL_SURFACE('',#15202,3.0735);
#1979=CYLINDRICAL_SURFACE('',#15204,3.0735);
#1980=CYLINDRICAL_SURFACE('',#15205,3.0735);
#1981=CYLINDRICAL_SURFACE('',#15206,3.0735);
#1982=CYLINDRICAL_SURFACE('',#15207,3.0735);
#1983=CYLINDRICAL_SURFACE('',#15208,3.0735);
#1984=CYLINDRICAL_SURFACE('',#15209,3.0735);
#1985=CYLINDRICAL_SURFACE('',#15210,3.0735);
#1986=CYLINDRICAL_SURFACE('',#15213,3.0735);
#1987=CYLINDRICAL_SURFACE('',#15214,2.5175);
#1988=CYLINDRICAL_SURFACE('',#15216,3.0735);
#1989=CYLINDRICAL_SURFACE('',#15217,2.5175);
#1990=CYLINDRICAL_SURFACE('',#15219,3.0735);
#1991=CYLINDRICAL_SURFACE('',#15220,2.5175);
#1992=CYLINDRICAL_SURFACE('',#15227,30.);
#2185=SHAPE_REPRESENTATION_RELATIONSHIP('SRR','None',#63870,#2201);
#2201=ADVANCED_BREP_SHAPE_REPRESENTATION('',(#2233),#63748);
#2217=STYLED_ITEM('',(#63962),#2233);
#2233=MANIFOLD_SOLID_BREP('Body1',#14318);
#2281=FACE_BOUND('',#3638,.T.);
#2282=FACE_BOUND('',#3639,.T.);
#2283=FACE_BOUND('',#3640,.T.);
#2284=FACE_BOUND('',#3641,.T.);
#2768=FACE_OUTER_BOUND('',#3569,.T.);
#2769=FACE_OUTER_BOUND('',#3570,.T.);
#2770=FACE_OUTER_BOUND('',#3571,.T.);
#2771=FACE_OUTER_BOUND('',#3572,.T.);
#2772=FACE_OUTER_BOUND('',#3573,.T.);
#2773=FACE_OUTER_BOUND('',#3574,.T.);
#2774=FACE_OUTER_BOUND('',#3575,.T.);
#2775=FACE_OUTER_BOUND('',#3576,.T.);
#2776=FACE_OUTER_BOUND('',#3577,.T.);
#2777=FACE_OUTER_BOUND('',#3578,.T.);
#2778=FACE_OUTER_BOUND('',#3579,.T.);
#2779=FACE_OUTER_BOUND('',#3580,.T.);
#2780=FACE_OUTER_BOUND('',#3581,.T.);
#2781=FACE_OUTER_BOUND('',#3582,.T.);
#2782=FACE_OUTER_BOUND('',#3583,.T.);
#2783=FACE_OUTER_BOUND('',#3584,.T.);
#2784=FACE_OUTER_BOUND('',#3585,.T.);
#2785=FACE_OUTER_BOUND('',#3586,.T.);
#2786=FACE_OUTER_BOUND('',#3587,.T.);
#2787=FACE_OUTER_BOUND('',#3588,.T.);
#2788=FACE_OUTER_BOUND('',#3589,.T.);
#2789=FACE_OUTER_BOUND('',#3590,.T.);
#2790=FACE_OUTER_BOUND('',#3591,.T.);
#2791=FACE_OUTER_BOUND('',#3592,.T.);
#2792=FACE_OUTER_BOUND('',#3593,.T.);
#2793=FACE_OUTER_BOUND('',#3594,.T.);
#2794=FACE_OUTER_BOUND('',#3595,.T.);
#2795=FACE_OUTER_BOUND('',#3596,.T.);
#2796=FACE_OUTER_BOUND('',#3597,.T.);
#2797=FACE_OUTER_BOUND('',#3598,.T.);
#2798=FACE_OUTER_BOUND('',#3599,.T.);
#2799=FACE_OUTER_BOUND('',#3600,.T.);
#2800=FACE_OUTER_BOUND('',#3601,.T.);
#2801=FACE_OUTER_BOUND('',#3602,.T.);
#2802=FACE_OUTER_BOUND('',#3603,.T.);
#2803=FACE_OUTER_BOUND('',#3604,.T.);
#2804=FACE_OUTER_BOUND('',#3605,.T.);
#2805=FACE_OUTER_BOUND('',#3606,.T.);
#2806=FACE_OUTER_BOUND('',#3607,.T.);
#2807=FACE_OUTER_BOUND('',#3608,.T.);
#2808=FACE_OUTER_BOUND('',#3609,.T.);
#2809=FACE_OUTER_BOUND('',#3610,.T.);
#2810=FACE_OUTER_BOUND('',#3611,.T.);
#2811=FACE_OUTER_BOUND('',#3612,.T.);
#2812=FACE_OUTER_BOUND('',#3613,.T.);
#2813=FACE_OUTER_BOUND('',#3614,.T.);
#2814=FACE_OUTER_BOUND('',#3615,.T.);
#2815=FACE_OUTER_BOUND('',#3616,.T.);
#2816=FACE_OUTER_BOUND('',#3617,.T.);
#2817=FACE_OUTER_BOUND('',#3618,.T.);
#2818=FACE_OUTER_BOUND('',#3619,.T.);
#2819=FACE_OUTER_BOUND('',#3620,.T.);
#2820=FACE_OUTER_BOUND('',#3621,.T.);
#2821=FACE_OUTER_BOUND('',#3622,.T.);
#2822=FACE_OUTER_BOUND('',#3623,.T.);
#2823=FACE_OUTER_BOUND('',#3624,.T.);
#2824=FACE_OUTER_BOUND('',#3625,.T.);
#2825=FACE_OUTER_BOUND('',#3626,.T.);
#2826=FACE_OUTER_BOUND('',#3627,.T.);
#2827=FACE_OUTER_BOUND('',#3628,.T.);
#2828=FACE_OUTER_BOUND('',#3629,.T.);
#2829=FACE_OUTER_BOUND('',#3630,.T.);
#2830=FACE_OUTER_BOUND('',#3631,.T.);
#2831=FACE_OUTER_BOUND('',#3632,.T.);
#2832=FACE_OUTER_BOUND('',#3633,.T.);
#2833=FACE_OUTER_BOUND('',#3634,.T.);
#2834=FACE_OUTER_BOUND('',#3635,.T.);
#2835=FACE_OUTER_BOUND('',#3636,.T.);
#2836=FACE_OUTER_BOUND('',#3637,.T.);
#2837=FACE_OUTER_BOUND('',#3642,.T.);
#3569=EDGE_LOOP('',(#11767,#11768,#11769,#11770,#11771,#11772,#11773,#11774));
#3570=EDGE_LOOP('',(#11775,#11776,#11777,#11778));
#3571=EDGE_LOOP('',(#11779,#11780,#11781,#11782));
#3572=EDGE_LOOP('',(#11783,#11784,#11785,#11786));
#3573=EDGE_LOOP('',(#11787,#11788,#11789,#11790));
#3574=EDGE_LOOP('',(#11791,#11792,#11793,#11794));
#3575=EDGE_LOOP('',(#11795,#11796,#11797,#11798));
#3576=EDGE_LOOP('',(#11799,#11800,#11801,#11802));
#3577=EDGE_LOOP('',(#11803,#11804,#11805,#11806));
#3578=EDGE_LOOP('',(#11807,#11808,#11809,#11810));
#3579=EDGE_LOOP('',(#11811,#11812,#11813,#11814));
#3580=EDGE_LOOP('',(#11815,#11816,#11817,#11818));
#3581=EDGE_LOOP('',(#11819,#11820,#11821,#11822));
#3582=EDGE_LOOP('',(#11823,#11824,#11825,#11826));
#3583=EDGE_LOOP('',(#11827,#11828,#11829,#11830));
#3584=EDGE_LOOP('',(#11831,#11832,#11833,#11834));
#3585=EDGE_LOOP('',(#11835,#11836,#11837,#11838,#11839,#11840,#11841,#11842));
#3586=EDGE_LOOP('',(#11843,#11844,#11845,#11846));
#3587=EDGE_LOOP('',(#11847,#11848,#11849,#11850));
#3588=EDGE_LOOP('',(#11851,#11852,#11853,#11854));
#3589=EDGE_LOOP('',(#11855,#11856,#11857,#11858));
#3590=EDGE_LOOP('',(#11859,#11860,#11861,#11862));
#3591=EDGE_LOOP('',(#11863,#11864,#11865,#11866));
#3592=EDGE_LOOP('',(#11867,#11868,#11869,#11870));
#3593=EDGE_LOOP('',(#11871,#11872,#11873,#11874));
#3594=EDGE_LOOP('',(#11875,#11876,#11877,#11878));
#3595=EDGE_LOOP('',(#11879,#11880,#11881,#11882));
#3596=EDGE_LOOP('',(#11883,#11884,#11885,#11886));
#3597=EDGE_LOOP('',(#11887,#11888,#11889,#11890));
#3598=EDGE_LOOP('',(#11891,#11892,#11893,#11894));
#3599=EDGE_LOOP('',(#11895,#11896,#11897,#11898));
#3600=EDGE_LOOP('',(#11899,#11900,#11901,#11902));
#3601=EDGE_LOOP('',(#11903,#11904,#11905,#11906,#11907,#11908,#11909,#11910));
#3602=EDGE_LOOP('',(#11911,#11912,#11913,#11914));
#3603=EDGE_LOOP('',(#11915,#11916,#11917,#11918));
#3604=EDGE_LOOP('',(#11919,#11920,#11921,#11922));
#3605=EDGE_LOOP('',(#11923,#11924,#11925,#11926));
#3606=EDGE_LOOP('',(#11927,#11928,#11929,#11930));
#3607=EDGE_LOOP('',(#11931,#11932,#11933,#11934));
#3608=EDGE_LOOP('',(#11935,#11936,#11937,#11938));
#3609=EDGE_LOOP('',(#11939,#11940,#11941,#11942));
#3610=EDGE_LOOP('',(#11943,#11944,#11945,#11946));
#3611=EDGE_LOOP('',(#11947,#11948,#11949,#11950));
#3612=EDGE_LOOP('',(#11951,#11952,#11953,#11954));
#3613=EDGE_LOOP('',(#11955,#11956,#11957,#11958));
#3614=EDGE_LOOP('',(#11959,#11960,#11961,#11962));
#3615=EDGE_LOOP('',(#11963,#11964,#11965,#11966));
#3616=EDGE_LOOP('',(#11967,#11968,#11969,#11970));
#3617=EDGE_LOOP('',(#11971,#11972,#11973,#11974,#11975));
#3618=EDGE_LOOP('',(#11976,#11977,#11978,#11979));
#3619=EDGE_LOOP('',(#11980,#11981,#11982,#11983,#11984,#11985,#11986,#11987,
#11988,#11989,#11990,#11991,#11992,#11993,#11994,#11995,#11996,#11997,#11998,
#11999));
#3620=EDGE_LOOP('',(#12000,#12001,#12002,#12003,#12004,#12005,#12006,#12007,
#12008,#12009,#12010,#12011,#12012,#12013,#12014,#12015,#12016,#12017,#12018,
#12019));
#3621=EDGE_LOOP('',(#12020,#12021,#12022,#12023));
#3622=EDGE_LOOP('',(#12024,#12025,#12026,#12027,#12028));
#3623=EDGE_LOOP('',(#12029,#12030,#12031,#12032));
#3624=EDGE_LOOP('',(#12033,#12034,#12035,#12036,#12037,#12038,#12039,#12040,
#12041,#12042,#12043,#12044,#12045,#12046,#12047,#12048,#12049,#12050,#12051,
#12052));
#3625=EDGE_LOOP('',(#12053,#12054,#12055,#12056,#12057,#12058,#12059,#12060,
#12061,#12062,#12063,#12064,#12065,#12066,#12067,#12068,#12069,#12070,#12071,
#12072));
#3626=EDGE_LOOP('',(#12073,#12074,#12075,#12076));
#3627=EDGE_LOOP('',(#12077,#12078,#12079,#12080,#12081));
#3628=EDGE_LOOP('',(#12082,#12083,#12084,#12085));
#3629=EDGE_LOOP('',(#12086,#12087,#12088,#12089,#12090,#12091,#12092,#12093,
#12094,#12095,#12096,#12097,#12098,#12099,#12100,#12101,#12102,#12103,#12104,
#12105));
#3630=EDGE_LOOP('',(#12106,#12107,#12108,#12109,#12110,#12111,#12112,#12113,
#12114,#12115,#12116,#12117,#12118,#12119,#12120,#12121,#12122,#12123,#12124,
#12125));
#3631=EDGE_LOOP('',(#12126,#12127,#12128,#12129));
#3632=EDGE_LOOP('',(#12130));
#3633=EDGE_LOOP('',(#12131));
#3634=EDGE_LOOP('',(#12132));
#3635=EDGE_LOOP('',(#12133,#12134,#12135));
#3636=EDGE_LOOP('',(#12136,#12137,#12138,#12139));
#3637=EDGE_LOOP('',(#12140));
#3638=EDGE_LOOP('',(#12141,#12142,#12143,#12144));
#3639=EDGE_LOOP('',(#12145,#12146,#12147,#12148));
#3640=EDGE_LOOP('',(#12149,#12150,#12151,#12152));
#3641=EDGE_LOOP('',(#12153));
#3642=EDGE_LOOP('',(#12154));
#4438=LINE('',#47157,#5274);
#4439=LINE('',#47166,#5275);
#4440=LINE('',#47183,#5276);
#4441=LINE('',#47234,#5277);
#4442=LINE('',#47285,#5278);
#4443=LINE('',#47333,#5279);
#4444=LINE('',#47384,#5280);
#4445=LINE('',#47435,#5281);
#4446=LINE('',#47483,#5282);
#4447=LINE('',#47522,#5283);
#4448=LINE('',#47546,#5284);
#4449=LINE('',#47570,#5285);
#4450=LINE('',#47595,#5286);
#4451=LINE('',#47620,#5287);
#4452=LINE('',#47644,#5288);
#4453=LINE('',#47669,#5289);
#4454=LINE('',#47694,#5290);
#4455=LINE('',#47711,#5291);
#4456=LINE('',#47720,#5292);
#4457=LINE('',#47737,#5293);
#4458=LINE('',#47788,#5294);
#4459=LINE('',#47839,#5295);
#4460=LINE('',#47887,#5296);
#4461=LINE('',#47938,#5297);
#4462=LINE('',#47989,#5298);
#4463=LINE('',#48037,#5299);
#4464=LINE('',#48076,#5300);
#4465=LINE('',#48100,#5301);
#4466=LINE('',#48124,#5302);
#4467=LINE('',#48149,#5303);
#4468=LINE('',#48174,#5304);
#4469=LINE('',#48198,#5305);
#4470=LINE('',#48223,#5306);
#4471=LINE('',#48248,#5307);
#4472=LINE('',#48265,#5308);
#4473=LINE('',#48274,#5309);
#4474=LINE('',#48291,#5310);
#4475=LINE('',#48342,#5311);
#4476=LINE('',#48393,#5312);
#4477=LINE('',#48441,#5313);
#4478=LINE('',#48492,#5314);
#4479=LINE('',#48543,#5315);
#4480=LINE('',#48591,#5316);
#4481=LINE('',#48630,#5317);
#4482=LINE('',#48654,#5318);
#4483=LINE('',#48678,#5319);
#4484=LINE('',#48703,#5320);
#4485=LINE('',#48728,#5321);
#4486=LINE('',#48752,#5322);
#4487=LINE('',#48777,#5323);
#4488=LINE('',#48802,#5324);
#4489=LINE('',#51504,#5325);
#5274=VECTOR('',#17357,3.);
#5275=VECTOR('',#17360,3.);
#5276=VECTOR('',#17367,3.);
#5277=VECTOR('',#17370,3.);
#5278=VECTOR('',#17373,3.);
#5279=VECTOR('',#17376,3.);
#5280=VECTOR('',#17379,3.);
#5281=VECTOR('',#17382,3.);
#5282=VECTOR('',#17385,3.);
#5283=VECTOR('',#17390,3.0735);
#5284=VECTOR('',#17395,3.0735);
#5285=VECTOR('',#17398,3.0735);
#5286=VECTOR('',#17401,3.0735);
#5287=VECTOR('',#17404,3.0735);
#5288=VECTOR('',#17407,3.0735);
#5289=VECTOR('',#17410,3.0735);
#5290=VECTOR('',#17413,3.0735);
#5291=VECTOR('',#17418,3.);
#5292=VECTOR('',#17421,3.);
#5293=VECTOR('',#17428,3.);
#5294=VECTOR('',#17431,3.);
#5295=VECTOR('',#17434,3.);
#5296=VECTOR('',#17437,3.);
#5297=VECTOR('',#17440,3.);
#5298=VECTOR('',#17443,3.);
#5299=VECTOR('',#17446,3.);
#5300=VECTOR('',#17451,3.0735);
#5301=VECTOR('',#17456,3.0735);
#5302=VECTOR('',#17459,3.0735);
#5303=VECTOR('',#17462,3.0735);
#5304=VECTOR('',#17465,3.0735);
#5305=VECTOR('',#17468,3.0735);
#5306=VECTOR('',#17471,3.0735);
#5307=VECTOR('',#17474,3.0735);
#5308=VECTOR('',#17479,3.);
#5309=VECTOR('',#17482,3.);
#5310=VECTOR('',#17489,3.);
#5311=VECTOR('',#17492,3.);
#5312=VECTOR('',#17495,3.);
#5313=VECTOR('',#17498,3.);
#5314=VECTOR('',#17501,3.);
#5315=VECTOR('',#17504,3.);
#5316=VECTOR('',#17507,3.);
#5317=VECTOR('',#17512,3.0735);
#5318=VECTOR('',#17517,3.0735);
#5319=VECTOR('',#17520,3.0735);
#5320=VECTOR('',#17523,3.0735);
#5321=VECTOR('',#17526,3.0735);
#5322=VECTOR('',#17529,3.0735);
#5323=VECTOR('',#17532,3.0735);
#5324=VECTOR('',#17535,3.0735);
#5325=VECTOR('',#17572,30.);
#6438=VERTEX_POINT('',#47155);
#6439=VERTEX_POINT('',#47156);
#6440=VERTEX_POINT('',#47158);
#6441=VERTEX_POINT('',#47163);
#6442=VERTEX_POINT('',#47165);
#6443=VERTEX_POINT('',#47168);
#6444=VERTEX_POINT('',#47181);
#6445=VERTEX_POINT('',#47182);
#6446=VERTEX_POINT('',#47232);
#6447=VERTEX_POINT('',#47233);
#6448=VERTEX_POINT('',#47283);
#6449=VERTEX_POINT('',#47284);
#6450=VERTEX_POINT('',#47331);
#6451=VERTEX_POINT('',#47332);
#6452=VERTEX_POINT('',#47382);
#6453=VERTEX_POINT('',#47383);
#6454=VERTEX_POINT('',#47433);
#6455=VERTEX_POINT('',#47434);
#6456=VERTEX_POINT('',#47481);
#6457=VERTEX_POINT('',#47482);
#6458=VERTEX_POINT('',#47484);
#6459=VERTEX_POINT('',#47498);
#6460=VERTEX_POINT('',#47520);
#6461=VERTEX_POINT('',#47521);
#6462=VERTEX_POINT('',#47523);
#6463=VERTEX_POINT('',#47532);
#6464=VERTEX_POINT('',#47544);
#6465=VERTEX_POINT('',#47545);
#6466=VERTEX_POINT('',#47568);
#6467=VERTEX_POINT('',#47569);
#6468=VERTEX_POINT('',#47593);
#6469=VERTEX_POINT('',#47594);
#6470=VERTEX_POINT('',#47618);
#6471=VERTEX_POINT('',#47619);
#6472=VERTEX_POINT('',#47642);
#6473=VERTEX_POINT('',#47643);
#6474=VERTEX_POINT('',#47667);
#6475=VERTEX_POINT('',#47668);
#6476=VERTEX_POINT('',#47692);
#6477=VERTEX_POINT('',#47693);
#6478=VERTEX_POINT('',#47695);
#6479=VERTEX_POINT('',#47701);
#6480=VERTEX_POINT('',#47709);
#6481=VERTEX_POINT('',#47710);
#6482=VERTEX_POINT('',#47712);
#6483=VERTEX_POINT('',#47717);
#6484=VERTEX_POINT('',#47719);
#6485=VERTEX_POINT('',#47722);
#6486=VERTEX_POINT('',#47735);
#6487=VERTEX_POINT('',#47736);
#6488=VERTEX_POINT('',#47786);
#6489=VERTEX_POINT('',#47787);
#6490=VERTEX_POINT('',#47837);
#6491=VERTEX_POINT('',#47838);
#6492=VERTEX_POINT('',#47885);
#6493=VERTEX_POINT('',#47886);
#6494=VERTEX_POINT('',#47936);
#6495=VERTEX_POINT('',#47937);
#6496=VERTEX_POINT('',#47987);
#6497=VERTEX_POINT('',#47988);
#6498=VERTEX_POINT('',#48035);
#6499=VERTEX_POINT('',#48036);
#6500=VERTEX_POINT('',#48038);
#6501=VERTEX_POINT('',#48052);
#6502=VERTEX_POINT('',#48074);
#6503=VERTEX_POINT('',#48075);
#6504=VERTEX_POINT('',#48077);
#6505=VERTEX_POINT('',#48086);
#6506=VERTEX_POINT('',#48098);
#6507=VERTEX_POINT('',#48099);
#6508=VERTEX_POINT('',#48122);
#6509=VERTEX_POINT('',#48123);
#6510=VERTEX_POINT('',#48147);
#6511=VERTEX_POINT('',#48148);
#6512=VERTEX_POINT('',#48172);
#6513=VERTEX_POINT('',#48173);
#6514=VERTEX_POINT('',#48196);
#6515=VERTEX_POINT('',#48197);
#6516=VERTEX_POINT('',#48221);
#6517=VERTEX_POINT('',#48222);
#6518=VERTEX_POINT('',#48246);
#6519=VERTEX_POINT('',#48247);
#6520=VERTEX_POINT('',#48249);
#6521=VERTEX_POINT('',#48255);
#6522=VERTEX_POINT('',#48263);
#6523=VERTEX_POINT('',#48264);
#6524=VERTEX_POINT('',#48266);
#6525=VERTEX_POINT('',#48271);
#6526=VERTEX_POINT('',#48273);
#6527=VERTEX_POINT('',#48276);
#6528=VERTEX_POINT('',#48289);
#6529=VERTEX_POINT('',#48290);
#6530=VERTEX_POINT('',#48340);
#6531=VERTEX_POINT('',#48341);
#6532=VERTEX_POINT('',#48391);
#6533=VERTEX_POINT('',#48392);
#6534=VERTEX_POINT('',#48439);
#6535=VERTEX_POINT('',#48440);
#6536=VERTEX_POINT('',#48490);
#6537=VERTEX_POINT('',#48491);
#6538=VERTEX_POINT('',#48541);
#6539=VERTEX_POINT('',#48542);
#6540=VERTEX_POINT('',#48589);
#6541=VERTEX_POINT('',#48590);
#6542=VERTEX_POINT('',#48592);
#6543=VERTEX_POINT('',#48606);
#6544=VERTEX_POINT('',#48628);
#6545=VERTEX_POINT('',#48629);
#6546=VERTEX_POINT('',#48631);
#6547=VERTEX_POINT('',#48640);
#6548=VERTEX_POINT('',#48652);
#6549=VERTEX_POINT('',#48653);
#6550=VERTEX_POINT('',#48676);
#6551=VERTEX_POINT('',#48677);
#6552=VERTEX_POINT('',#48701);
#6553=VERTEX_POINT('',#48702);
#6554=VERTEX_POINT('',#48726);
#6555=VERTEX_POINT('',#48727);
#6556=VERTEX_POINT('',#48750);
#6557=VERTEX_POINT('',#48751);
#6558=VERTEX_POINT('',#48775);
#6559=VERTEX_POINT('',#48776);
#6560=VERTEX_POINT('',#48800);
#6561=VERTEX_POINT('',#48801);
#6562=VERTEX_POINT('',#48803);
#6563=VERTEX_POINT('',#48809);
#6564=VERTEX_POINT('',#51496);
#6565=VERTEX_POINT('',#51498);
#6566=VERTEX_POINT('',#51501);
#6567=VERTEX_POINT('',#51503);
#8306=EDGE_CURVE('',#6438,#6439,#4438,.T.);
#8307=EDGE_CURVE('',#6439,#6440,#1113,.T.);
#8308=EDGE_CURVE('',#6440,#6441,#427,.T.);
#8309=EDGE_CURVE('',#6441,#6442,#4439,.T.);
#8310=EDGE_CURVE('',#6442,#6442,#428,.F.);
#8311=EDGE_CURVE('',#6441,#6443,#429,.T.);
#8312=EDGE_CURVE('',#6443,#6438,#1114,.T.);
#8313=EDGE_CURVE('',#6444,#6445,#4440,.T.);
#8314=EDGE_CURVE('',#6445,#6439,#1115,.T.);
#8315=EDGE_CURVE('',#6438,#6444,#1116,.T.);
#8316=EDGE_CURVE('',#6446,#6447,#4441,.T.);
#8317=EDGE_CURVE('',#6447,#6445,#1117,.T.);
#8318=EDGE_CURVE('',#6444,#6446,#1118,.T.);
#8319=EDGE_CURVE('',#6448,#6449,#4442,.T.);
#8320=EDGE_CURVE('',#6449,#6447,#1119,.T.);
#8321=EDGE_CURVE('',#6446,#6448,#1120,.T.);
#8322=EDGE_CURVE('',#6450,#6451,#4443,.T.);
#8323=EDGE_CURVE('',#6451,#6449,#1121,.T.);
#8324=EDGE_CURVE('',#6448,#6450,#1122,.T.);
#8325=EDGE_CURVE('',#6452,#6453,#4444,.T.);
#8326=EDGE_CURVE('',#6453,#6451,#1123,.T.);
#8327=EDGE_CURVE('',#6450,#6452,#1124,.T.);
#8328=EDGE_CURVE('',#6454,#6455,#4445,.T.);
#8329=EDGE_CURVE('',#6455,#6453,#1125,.T.);
#8330=EDGE_CURVE('',#6452,#6454,#1126,.T.);
#8331=EDGE_CURVE('',#6456,#6457,#4446,.T.);
#8332=EDGE_CURVE('',#6456,#6458,#1127,.T.);
#8333=EDGE_CURVE('',#6459,#6458,#430,.T.);
#8334=EDGE_CURVE('',#6459,#6457,#1128,.T.);
#8335=EDGE_CURVE('',#6460,#6461,#4447,.T.);
#8336=EDGE_CURVE('',#6461,#6462,#1129,.T.);
#8337=EDGE_CURVE('',#6463,#6462,#431,.T.);
#8338=EDGE_CURVE('',#6460,#6463,#1130,.T.);
#8339=EDGE_CURVE('',#6464,#6465,#4448,.T.);
#8340=EDGE_CURVE('',#6465,#6461,#1131,.T.);
#8341=EDGE_CURVE('',#6464,#6460,#1132,.T.);
#8342=EDGE_CURVE('',#6466,#6467,#4449,.T.);
#8343=EDGE_CURVE('',#6467,#6465,#1133,.T.);
#8344=EDGE_CURVE('',#6466,#6464,#1134,.T.);
#8345=EDGE_CURVE('',#6468,#6469,#4450,.T.);
#8346=EDGE_CURVE('',#6469,#6467,#1135,.T.);
#8347=EDGE_CURVE('',#6468,#6466,#1136,.T.);
#8348=EDGE_CURVE('',#6470,#6471,#4451,.T.);
#8349=EDGE_CURVE('',#6471,#6469,#1137,.T.);
#8350=EDGE_CURVE('',#6470,#6468,#1138,.T.);
#8351=EDGE_CURVE('',#6472,#6473,#4452,.T.);
#8352=EDGE_CURVE('',#6473,#6471,#1139,.T.);
#8353=EDGE_CURVE('',#6472,#6470,#1140,.T.);
#8354=EDGE_CURVE('',#6474,#6475,#4453,.T.);
#8355=EDGE_CURVE('',#6475,#6473,#1141,.T.);
#8356=EDGE_CURVE('',#6474,#6472,#1142,.T.);
#8357=EDGE_CURVE('',#6476,#6477,#4454,.T.);
#8358=EDGE_CURVE('',#6478,#6476,#1143,.T.);
#8359=EDGE_CURVE('',#6479,#6478,#432,.T.);
#8360=EDGE_CURVE('',#6479,#6477,#1144,.T.);
#8361=EDGE_CURVE('',#6480,#6481,#4455,.T.);
#8362=EDGE_CURVE('',#6481,#6482,#1145,.T.);
#8363=EDGE_CURVE('',#6482,#6483,#433,.T.);
#8364=EDGE_CURVE('',#6483,#6484,#4456,.T.);
#8365=EDGE_CURVE('',#6484,#6484,#434,.F.);
#8366=EDGE_CURVE('',#6483,#6485,#435,.T.);
#8367=EDGE_CURVE('',#6485,#6480,#1146,.T.);
#8368=EDGE_CURVE('',#6486,#6487,#4457,.T.);
#8369=EDGE_CURVE('',#6487,#6481,#1147,.T.);
#8370=EDGE_CURVE('',#6480,#6486,#1148,.T.);
#8371=EDGE_CURVE('',#6488,#6489,#4458,.T.);
#8372=EDGE_CURVE('',#6489,#6487,#1149,.T.);
#8373=EDGE_CURVE('',#6486,#6488,#1150,.T.);
#8374=EDGE_CURVE('',#6490,#6491,#4459,.T.);
#8375=EDGE_CURVE('',#6491,#6489,#1151,.T.);
#8376=EDGE_CURVE('',#6488,#6490,#1152,.T.);
#8377=EDGE_CURVE('',#6492,#6493,#4460,.T.);
#8378=EDGE_CURVE('',#6493,#6491,#1153,.T.);
#8379=EDGE_CURVE('',#6490,#6492,#1154,.T.);
#8380=EDGE_CURVE('',#6494,#6495,#4461,.T.);
#8381=EDGE_CURVE('',#6495,#6493,#1155,.T.);
#8382=EDGE_CURVE('',#6492,#6494,#1156,.T.);
#8383=EDGE_CURVE('',#6496,#6497,#4462,.T.);
#8384=EDGE_CURVE('',#6497,#6495,#1157,.T.);
#8385=EDGE_CURVE('',#6494,#6496,#1158,.T.);
#8386=EDGE_CURVE('',#6498,#6499,#4463,.T.);
#8387=EDGE_CURVE('',#6498,#6500,#1159,.T.);
#8388=EDGE_CURVE('',#6501,#6500,#436,.T.);
#8389=EDGE_CURVE('',#6501,#6499,#1160,.T.);
#8390=EDGE_CURVE('',#6502,#6503,#4464,.T.);
#8391=EDGE_CURVE('',#6503,#6504,#1161,.T.);
#8392=EDGE_CURVE('',#6505,#6504,#437,.T.);
#8393=EDGE_CURVE('',#6502,#6505,#1162,.T.);
#8394=EDGE_CURVE('',#6506,#6507,#4465,.T.);
#8395=EDGE_CURVE('',#6507,#6503,#1163,.T.);
#8396=EDGE_CURVE('',#6506,#6502,#1164,.T.);
#8397=EDGE_CURVE('',#6508,#6509,#4466,.T.);
#8398=EDGE_CURVE('',#6509,#6507,#1165,.T.);
#8399=EDGE_CURVE('',#6508,#6506,#1166,.T.);
#8400=EDGE_CURVE('',#6510,#6511,#4467,.T.);
#8401=EDGE_CURVE('',#6511,#6509,#1167,.T.);
#8402=EDGE_CURVE('',#6510,#6508,#1168,.T.);
#8403=EDGE_CURVE('',#6512,#6513,#4468,.T.);
#8404=EDGE_CURVE('',#6513,#6511,#1169,.T.);
#8405=EDGE_CURVE('',#6512,#6510,#1170,.T.);
#8406=EDGE_CURVE('',#6514,#6515,#4469,.T.);
#8407=EDGE_CURVE('',#6515,#6513,#1171,.T.);
#8408=EDGE_CURVE('',#6514,#6512,#1172,.T.);
#8409=EDGE_CURVE('',#6516,#6517,#4470,.T.);
#8410=EDGE_CURVE('',#6517,#6515,#1173,.T.);
#8411=EDGE_CURVE('',#6516,#6514,#1174,.T.);
#8412=EDGE_CURVE('',#6518,#6519,#4471,.T.);
#8413=EDGE_CURVE('',#6520,#6518,#1175,.T.);
#8414=EDGE_CURVE('',#6521,#6520,#438,.T.);
#8415=EDGE_CURVE('',#6521,#6519,#1176,.T.);
#8416=EDGE_CURVE('',#6522,#6523,#4472,.T.);
#8417=EDGE_CURVE('',#6523,#6524,#1177,.T.);
#8418=EDGE_CURVE('',#6524,#6525,#439,.T.);
#8419=EDGE_CURVE('',#6525,#6526,#4473,.T.);
#8420=EDGE_CURVE('',#6526,#6526,#440,.F.);
#8421=EDGE_CURVE('',#6525,#6527,#441,.T.);
#8422=EDGE_CURVE('',#6527,#6522,#1178,.T.);
#8423=EDGE_CURVE('',#6528,#6529,#4474,.T.);
#8424=EDGE_CURVE('',#6529,#6523,#1179,.T.);
#8425=EDGE_CURVE('',#6522,#6528,#1180,.T.);
#8426=EDGE_CURVE('',#6530,#6531,#4475,.T.);
#8427=EDGE_CURVE('',#6531,#6529,#1181,.T.);
#8428=EDGE_CURVE('',#6528,#6530,#1182,.T.);
#8429=EDGE_CURVE('',#6532,#6533,#4476,.T.);
#8430=EDGE_CURVE('',#6533,#6531,#1183,.T.);
#8431=EDGE_CURVE('',#6530,#6532,#1184,.T.);
#8432=EDGE_CURVE('',#6534,#6535,#4477,.T.);
#8433=EDGE_CURVE('',#6535,#6533,#1185,.T.);
#8434=EDGE_CURVE('',#6532,#6534,#1186,.T.);
#8435=EDGE_CURVE('',#6536,#6537,#4478,.T.);
#8436=EDGE_CURVE('',#6537,#6535,#1187,.T.);
#8437=EDGE_CURVE('',#6534,#6536,#1188,.T.);
#8438=EDGE_CURVE('',#6538,#6539,#4479,.T.);
#8439=EDGE_CURVE('',#6539,#6537,#1189,.T.);
#8440=EDGE_CURVE('',#6536,#6538,#1190,.T.);
#8441=EDGE_CURVE('',#6540,#6541,#4480,.T.);
#8442=EDGE_CURVE('',#6540,#6542,#1191,.T.);
#8443=EDGE_CURVE('',#6543,#6542,#442,.T.);
#8444=EDGE_CURVE('',#6543,#6541,#1192,.T.);
#8445=EDGE_CURVE('',#6544,#6545,#4481,.T.);
#8446=EDGE_CURVE('',#6545,#6546,#1193,.T.);
#8447=EDGE_CURVE('',#6547,#6546,#443,.T.);
#8448=EDGE_CURVE('',#6544,#6547,#1194,.T.);
#8449=EDGE_CURVE('',#6548,#6549,#4482,.T.);
#8450=EDGE_CURVE('',#6549,#6545,#1195,.T.);
#8451=EDGE_CURVE('',#6548,#6544,#1196,.T.);
#8452=EDGE_CURVE('',#6550,#6551,#4483,.T.);
#8453=EDGE_CURVE('',#6551,#6549,#1197,.T.);
#8454=EDGE_CURVE('',#6550,#6548,#1198,.T.);
#8455=EDGE_CURVE('',#6552,#6553,#4484,.T.);
#8456=EDGE_CURVE('',#6553,#6551,#1199,.T.);
#8457=EDGE_CURVE('',#6552,#6550,#1200,.T.);
#8458=EDGE_CURVE('',#6554,#6555,#4485,.T.);
#8459=EDGE_CURVE('',#6555,#6553,#1201,.T.);
#8460=EDGE_CURVE('',#6554,#6552,#1202,.T.);
#8461=EDGE_CURVE('',#6556,#6557,#4486,.T.);
#8462=EDGE_CURVE('',#6557,#6555,#1203,.T.);
#8463=EDGE_CURVE('',#6556,#6554,#1204,.T.);
#8464=EDGE_CURVE('',#6558,#6559,#4487,.T.);
#8465=EDGE_CURVE('',#6559,#6557,#1205,.T.);
#8466=EDGE_CURVE('',#6558,#6556,#1206,.T.);
#8467=EDGE_CURVE('',#6560,#6561,#4488,.T.);
#8468=EDGE_CURVE('',#6562,#6560,#1207,.T.);
#8469=EDGE_CURVE('',#6563,#6562,#444,.T.);
#8470=EDGE_CURVE('',#6563,#6561,#1208,.T.);
#8471=EDGE_CURVE('',#6524,#6547,#1209,.T.);
#8472=EDGE_CURVE('',#6546,#6527,#1210,.T.);
#8473=EDGE_CURVE('',#6561,#6559,#1211,.T.);
#8474=EDGE_CURVE('',#6560,#6558,#1212,.T.);
#8475=EDGE_CURVE('',#6542,#6563,#1213,.T.);
#8476=EDGE_CURVE('',#6538,#6540,#1214,.T.);
#8477=EDGE_CURVE('',#6541,#6539,#1215,.T.);
#8478=EDGE_CURVE('',#6562,#6543,#1216,.T.);
#8479=EDGE_CURVE('',#6482,#6505,#1217,.T.);
#8480=EDGE_CURVE('',#6504,#6485,#1218,.T.);
#8481=EDGE_CURVE('',#6519,#6517,#1219,.T.);
#8482=EDGE_CURVE('',#6518,#6516,#1220,.T.);
#8483=EDGE_CURVE('',#6500,#6521,#1221,.T.);
#8484=EDGE_CURVE('',#6496,#6498,#1222,.T.);
#8485=EDGE_CURVE('',#6499,#6497,#1223,.T.);
#8486=EDGE_CURVE('',#6520,#6501,#1224,.T.);
#8487=EDGE_CURVE('',#6440,#6463,#1225,.T.);
#8488=EDGE_CURVE('',#6462,#6443,#1226,.T.);
#8489=EDGE_CURVE('',#6477,#6475,#1227,.T.);
#8490=EDGE_CURVE('',#6476,#6474,#1228,.T.);
#8491=EDGE_CURVE('',#6458,#6479,#1229,.T.);
#8492=EDGE_CURVE('',#6454,#6456,#1230,.T.);
#8493=EDGE_CURVE('',#6457,#6455,#1231,.T.);
#8494=EDGE_CURVE('',#6478,#6459,#1232,.T.);
#8495=EDGE_CURVE('',#6564,#6564,#445,.T.);
#8496=EDGE_CURVE('',#6565,#6564,#446,.T.);
#8497=EDGE_CURVE('',#6566,#6566,#447,.T.);
#8498=EDGE_CURVE('',#6566,#6567,#4489,.T.);
#8499=EDGE_CURVE('',#6567,#6567,#448,.T.);
#11767=ORIENTED_EDGE('',*,*,#8306,.T.);
#11768=ORIENTED_EDGE('',*,*,#8307,.T.);
#11769=ORIENTED_EDGE('',*,*,#8308,.T.);
#11770=ORIENTED_EDGE('',*,*,#8309,.T.);
#11771=ORIENTED_EDGE('',*,*,#8310,.T.);
#11772=ORIENTED_EDGE('',*,*,#8309,.F.);
#11773=ORIENTED_EDGE('',*,*,#8311,.T.);
#11774=ORIENTED_EDGE('',*,*,#8312,.T.);
#11775=ORIENTED_EDGE('',*,*,#8313,.T.);
#11776=ORIENTED_EDGE('',*,*,#8314,.T.);
#11777=ORIENTED_EDGE('',*,*,#8306,.F.);
#11778=ORIENTED_EDGE('',*,*,#8315,.T.);
#11779=ORIENTED_EDGE('',*,*,#8316,.T.);
#11780=ORIENTED_EDGE('',*,*,#8317,.T.);
#11781=ORIENTED_EDGE('',*,*,#8313,.F.);
#11782=ORIENTED_EDGE('',*,*,#8318,.T.);
#11783=ORIENTED_EDGE('',*,*,#8319,.T.);
#11784=ORIENTED_EDGE('',*,*,#8320,.T.);
#11785=ORIENTED_EDGE('',*,*,#8316,.F.);
#11786=ORIENTED_EDGE('',*,*,#8321,.T.);
#11787=ORIENTED_EDGE('',*,*,#8322,.T.);
#11788=ORIENTED_EDGE('',*,*,#8323,.T.);
#11789=ORIENTED_EDGE('',*,*,#8319,.F.);
#11790=ORIENTED_EDGE('',*,*,#8324,.T.);
#11791=ORIENTED_EDGE('',*,*,#8325,.T.);
#11792=ORIENTED_EDGE('',*,*,#8326,.T.);
#11793=ORIENTED_EDGE('',*,*,#8322,.F.);
#11794=ORIENTED_EDGE('',*,*,#8327,.T.);
#11795=ORIENTED_EDGE('',*,*,#8328,.T.);
#11796=ORIENTED_EDGE('',*,*,#8329,.T.);
#11797=ORIENTED_EDGE('',*,*,#8325,.F.);
#11798=ORIENTED_EDGE('',*,*,#8330,.T.);
#11799=ORIENTED_EDGE('',*,*,#8331,.F.);
#11800=ORIENTED_EDGE('',*,*,#8332,.T.);
#11801=ORIENTED_EDGE('',*,*,#8333,.F.);
#11802=ORIENTED_EDGE('',*,*,#8334,.T.);
#11803=ORIENTED_EDGE('',*,*,#8335,.T.);
#11804=ORIENTED_EDGE('',*,*,#8336,.T.);
#11805=ORIENTED_EDGE('',*,*,#8337,.F.);
#11806=ORIENTED_EDGE('',*,*,#8338,.F.);
#11807=ORIENTED_EDGE('',*,*,#8339,.T.);
#11808=ORIENTED_EDGE('',*,*,#8340,.T.);
#11809=ORIENTED_EDGE('',*,*,#8335,.F.);
#11810=ORIENTED_EDGE('',*,*,#8341,.F.);
#11811=ORIENTED_EDGE('',*,*,#8342,.T.);
#11812=ORIENTED_EDGE('',*,*,#8343,.T.);
#11813=ORIENTED_EDGE('',*,*,#8339,.F.);
#11814=ORIENTED_EDGE('',*,*,#8344,.F.);
#11815=ORIENTED_EDGE('',*,*,#8345,.T.);
#11816=ORIENTED_EDGE('',*,*,#8346,.T.);
#11817=ORIENTED_EDGE('',*,*,#8342,.F.);
#11818=ORIENTED_EDGE('',*,*,#8347,.F.);
#11819=ORIENTED_EDGE('',*,*,#8348,.T.);
#11820=ORIENTED_EDGE('',*,*,#8349,.T.);
#11821=ORIENTED_EDGE('',*,*,#8345,.F.);
#11822=ORIENTED_EDGE('',*,*,#8350,.F.);
#11823=ORIENTED_EDGE('',*,*,#8351,.T.);
#11824=ORIENTED_EDGE('',*,*,#8352,.T.);
#11825=ORIENTED_EDGE('',*,*,#8348,.F.);
#11826=ORIENTED_EDGE('',*,*,#8353,.F.);
#11827=ORIENTED_EDGE('',*,*,#8354,.T.);
#11828=ORIENTED_EDGE('',*,*,#8355,.T.);
#11829=ORIENTED_EDGE('',*,*,#8351,.F.);
#11830=ORIENTED_EDGE('',*,*,#8356,.F.);
#11831=ORIENTED_EDGE('',*,*,#8357,.F.);
#11832=ORIENTED_EDGE('',*,*,#8358,.F.);
#11833=ORIENTED_EDGE('',*,*,#8359,.F.);
#11834=ORIENTED_EDGE('',*,*,#8360,.T.);
#11835=ORIENTED_EDGE('',*,*,#8361,.T.);
#11836=ORIENTED_EDGE('',*,*,#8362,.T.);
#11837=ORIENTED_EDGE('',*,*,#8363,.T.);
#11838=ORIENTED_EDGE('',*,*,#8364,.T.);
#11839=ORIENTED_EDGE('',*,*,#8365,.T.);
#11840=ORIENTED_EDGE('',*,*,#8364,.F.);
#11841=ORIENTED_EDGE('',*,*,#8366,.T.);
#11842=ORIENTED_EDGE('',*,*,#8367,.T.);
#11843=ORIENTED_EDGE('',*,*,#8368,.T.);
#11844=ORIENTED_EDGE('',*,*,#8369,.T.);
#11845=ORIENTED_EDGE('',*,*,#8361,.F.);
#11846=ORIENTED_EDGE('',*,*,#8370,.T.);
#11847=ORIENTED_EDGE('',*,*,#8371,.T.);
#11848=ORIENTED_EDGE('',*,*,#8372,.T.);
#11849=ORIENTED_EDGE('',*,*,#8368,.F.);
#11850=ORIENTED_EDGE('',*,*,#8373,.T.);
#11851=ORIENTED_EDGE('',*,*,#8374,.T.);
#11852=ORIENTED_EDGE('',*,*,#8375,.T.);
#11853=ORIENTED_EDGE('',*,*,#8371,.F.);
#11854=ORIENTED_EDGE('',*,*,#8376,.T.);
#11855=ORIENTED_EDGE('',*,*,#8377,.T.);
#11856=ORIENTED_EDGE('',*,*,#8378,.T.);
#11857=ORIENTED_EDGE('',*,*,#8374,.F.);
#11858=ORIENTED_EDGE('',*,*,#8379,.T.);
#11859=ORIENTED_EDGE('',*,*,#8380,.T.);
#11860=ORIENTED_EDGE('',*,*,#8381,.T.);
#11861=ORIENTED_EDGE('',*,*,#8377,.F.);
#11862=ORIENTED_EDGE('',*,*,#8382,.T.);
#11863=ORIENTED_EDGE('',*,*,#8383,.T.);
#11864=ORIENTED_EDGE('',*,*,#8384,.T.);
#11865=ORIENTED_EDGE('',*,*,#8380,.F.);
#11866=ORIENTED_EDGE('',*,*,#8385,.T.);
#11867=ORIENTED_EDGE('',*,*,#8386,.F.);
#11868=ORIENTED_EDGE('',*,*,#8387,.T.);
#11869=ORIENTED_EDGE('',*,*,#8388,.F.);
#11870=ORIENTED_EDGE('',*,*,#8389,.T.);
#11871=ORIENTED_EDGE('',*,*,#8390,.T.);
#11872=ORIENTED_EDGE('',*,*,#8391,.T.);
#11873=ORIENTED_EDGE('',*,*,#8392,.F.);
#11874=ORIENTED_EDGE('',*,*,#8393,.F.);
#11875=ORIENTED_EDGE('',*,*,#8394,.T.);
#11876=ORIENTED_EDGE('',*,*,#8395,.T.);
#11877=ORIENTED_EDGE('',*,*,#8390,.F.);
#11878=ORIENTED_EDGE('',*,*,#8396,.F.);
#11879=ORIENTED_EDGE('',*,*,#8397,.T.);
#11880=ORIENTED_EDGE('',*,*,#8398,.T.);
#11881=ORIENTED_EDGE('',*,*,#8394,.F.);
#11882=ORIENTED_EDGE('',*,*,#8399,.F.);
#11883=ORIENTED_EDGE('',*,*,#8400,.T.);
#11884=ORIENTED_EDGE('',*,*,#8401,.T.);
#11885=ORIENTED_EDGE('',*,*,#8397,.F.);
#11886=ORIENTED_EDGE('',*,*,#8402,.F.);
#11887=ORIENTED_EDGE('',*,*,#8403,.T.);
#11888=ORIENTED_EDGE('',*,*,#8404,.T.);
#11889=ORIENTED_EDGE('',*,*,#8400,.F.);
#11890=ORIENTED_EDGE('',*,*,#8405,.F.);
#11891=ORIENTED_EDGE('',*,*,#8406,.T.);
#11892=ORIENTED_EDGE('',*,*,#8407,.T.);
#11893=ORIENTED_EDGE('',*,*,#8403,.F.);
#11894=ORIENTED_EDGE('',*,*,#8408,.F.);
#11895=ORIENTED_EDGE('',*,*,#8409,.T.);
#11896=ORIENTED_EDGE('',*,*,#8410,.T.);
#11897=ORIENTED_EDGE('',*,*,#8406,.F.);
#11898=ORIENTED_EDGE('',*,*,#8411,.F.);
#11899=ORIENTED_EDGE('',*,*,#8412,.F.);
#11900=ORIENTED_EDGE('',*,*,#8413,.F.);
#11901=ORIENTED_EDGE('',*,*,#8414,.F.);
#11902=ORIENTED_EDGE('',*,*,#8415,.T.);
#11903=ORIENTED_EDGE('',*,*,#8416,.T.);
#11904=ORIENTED_EDGE('',*,*,#8417,.T.);
#11905=ORIENTED_EDGE('',*,*,#8418,.T.);
#11906=ORIENTED_EDGE('',*,*,#8419,.T.);
#11907=ORIENTED_EDGE('',*,*,#8420,.T.);
#11908=ORIENTED_EDGE('',*,*,#8419,.F.);
#11909=ORIENTED_EDGE('',*,*,#8421,.T.);
#11910=ORIENTED_EDGE('',*,*,#8422,.T.);
#11911=ORIENTED_EDGE('',*,*,#8423,.T.);
#11912=ORIENTED_EDGE('',*,*,#8424,.T.);
#11913=ORIENTED_EDGE('',*,*,#8416,.F.);
#11914=ORIENTED_EDGE('',*,*,#8425,.T.);
#11915=ORIENTED_EDGE('',*,*,#8426,.T.);
#11916=ORIENTED_EDGE('',*,*,#8427,.T.);
#11917=ORIENTED_EDGE('',*,*,#8423,.F.);
#11918=ORIENTED_EDGE('',*,*,#8428,.T.);
#11919=ORIENTED_EDGE('',*,*,#8429,.T.);
#11920=ORIENTED_EDGE('',*,*,#8430,.T.);
#11921=ORIENTED_EDGE('',*,*,#8426,.F.);
#11922=ORIENTED_EDGE('',*,*,#8431,.T.);
#11923=ORIENTED_EDGE('',*,*,#8432,.T.);
#11924=ORIENTED_EDGE('',*,*,#8433,.T.);
#11925=ORIENTED_EDGE('',*,*,#8429,.F.);
#11926=ORIENTED_EDGE('',*,*,#8434,.T.);
#11927=ORIENTED_EDGE('',*,*,#8435,.T.);
#11928=ORIENTED_EDGE('',*,*,#8436,.T.);
#11929=ORIENTED_EDGE('',*,*,#8432,.F.);
#11930=ORIENTED_EDGE('',*,*,#8437,.T.);
#11931=ORIENTED_EDGE('',*,*,#8438,.T.);
#11932=ORIENTED_EDGE('',*,*,#8439,.T.);
#11933=ORIENTED_EDGE('',*,*,#8435,.F.);
#11934=ORIENTED_EDGE('',*,*,#8440,.T.);
#11935=ORIENTED_EDGE('',*,*,#8441,.F.);
#11936=ORIENTED_EDGE('',*,*,#8442,.T.);
#11937=ORIENTED_EDGE('',*,*,#8443,.F.);
#11938=ORIENTED_EDGE('',*,*,#8444,.T.);
#11939=ORIENTED_EDGE('',*,*,#8445,.T.);
#11940=ORIENTED_EDGE('',*,*,#8446,.T.);
#11941=ORIENTED_EDGE('',*,*,#8447,.F.);
#11942=ORIENTED_EDGE('',*,*,#8448,.F.);
#11943=ORIENTED_EDGE('',*,*,#8449,.T.);
#11944=ORIENTED_EDGE('',*,*,#8450,.T.);
#11945=ORIENTED_EDGE('',*,*,#8445,.F.);
#11946=ORIENTED_EDGE('',*,*,#8451,.F.);
#11947=ORIENTED_EDGE('',*,*,#8452,.T.);
#11948=ORIENTED_EDGE('',*,*,#8453,.T.);
#11949=ORIENTED_EDGE('',*,*,#8449,.F.);
#11950=ORIENTED_EDGE('',*,*,#8454,.F.);
#11951=ORIENTED_EDGE('',*,*,#8455,.T.);
#11952=ORIENTED_EDGE('',*,*,#8456,.T.);
#11953=ORIENTED_EDGE('',*,*,#8452,.F.);
#11954=ORIENTED_EDGE('',*,*,#8457,.F.);
#11955=ORIENTED_EDGE('',*,*,#8458,.T.);
#11956=ORIENTED_EDGE('',*,*,#8459,.T.);
#11957=ORIENTED_EDGE('',*,*,#8455,.F.);
#11958=ORIENTED_EDGE('',*,*,#8460,.F.);
#11959=ORIENTED_EDGE('',*,*,#8461,.T.);
#11960=ORIENTED_EDGE('',*,*,#8462,.T.);
#11961=ORIENTED_EDGE('',*,*,#8458,.F.);
#11962=ORIENTED_EDGE('',*,*,#8463,.F.);
#11963=ORIENTED_EDGE('',*,*,#8464,.T.);
#11964=ORIENTED_EDGE('',*,*,#8465,.T.);
#11965=ORIENTED_EDGE('',*,*,#8461,.F.);
#11966=ORIENTED_EDGE('',*,*,#8466,.F.);
#11967=ORIENTED_EDGE('',*,*,#8467,.F.);
#11968=ORIENTED_EDGE('',*,*,#8468,.F.);
#11969=ORIENTED_EDGE('',*,*,#8469,.F.);
#11970=ORIENTED_EDGE('',*,*,#8470,.T.);
#11971=ORIENTED_EDGE('',*,*,#8418,.F.);
#11972=ORIENTED_EDGE('',*,*,#8471,.T.);
#11973=ORIENTED_EDGE('',*,*,#8447,.T.);
#11974=ORIENTED_EDGE('',*,*,#8472,.T.);
#11975=ORIENTED_EDGE('',*,*,#8421,.F.);
#11976=ORIENTED_EDGE('',*,*,#8467,.T.);
#11977=ORIENTED_EDGE('',*,*,#8473,.T.);
#11978=ORIENTED_EDGE('',*,*,#8464,.F.);
#11979=ORIENTED_EDGE('',*,*,#8474,.F.);
#11980=ORIENTED_EDGE('',*,*,#8472,.F.);
#11981=ORIENTED_EDGE('',*,*,#8446,.F.);
#11982=ORIENTED_EDGE('',*,*,#8450,.F.);
#11983=ORIENTED_EDGE('',*,*,#8453,.F.);
#11984=ORIENTED_EDGE('',*,*,#8456,.F.);
#11985=ORIENTED_EDGE('',*,*,#8459,.F.);
#11986=ORIENTED_EDGE('',*,*,#8462,.F.);
#11987=ORIENTED_EDGE('',*,*,#8465,.F.);
#11988=ORIENTED_EDGE('',*,*,#8473,.F.);
#11989=ORIENTED_EDGE('',*,*,#8470,.F.);
#11990=ORIENTED_EDGE('',*,*,#8475,.F.);
#11991=ORIENTED_EDGE('',*,*,#8442,.F.);
#11992=ORIENTED_EDGE('',*,*,#8476,.F.);
#11993=ORIENTED_EDGE('',*,*,#8440,.F.);
#11994=ORIENTED_EDGE('',*,*,#8437,.F.);
#11995=ORIENTED_EDGE('',*,*,#8434,.F.);
#11996=ORIENTED_EDGE('',*,*,#8431,.F.);
#11997=ORIENTED_EDGE('',*,*,#8428,.F.);
#11998=ORIENTED_EDGE('',*,*,#8425,.F.);
#11999=ORIENTED_EDGE('',*,*,#8422,.F.);
#12000=ORIENTED_EDGE('',*,*,#8471,.F.);
#12001=ORIENTED_EDGE('',*,*,#8417,.F.);
#12002=ORIENTED_EDGE('',*,*,#8424,.F.);
#12003=ORIENTED_EDGE('',*,*,#8427,.F.);
#12004=ORIENTED_EDGE('',*,*,#8430,.F.);
#12005=ORIENTED_EDGE('',*,*,#8433,.F.);
#12006=ORIENTED_EDGE('',*,*,#8436,.F.);
#12007=ORIENTED_EDGE('',*,*,#8439,.F.);
#12008=ORIENTED_EDGE('',*,*,#8477,.F.);
#12009=ORIENTED_EDGE('',*,*,#8444,.F.);
#12010=ORIENTED_EDGE('',*,*,#8478,.F.);
#12011=ORIENTED_EDGE('',*,*,#8468,.T.);
#12012=ORIENTED_EDGE('',*,*,#8474,.T.);
#12013=ORIENTED_EDGE('',*,*,#8466,.T.);
#12014=ORIENTED_EDGE('',*,*,#8463,.T.);
#12015=ORIENTED_EDGE('',*,*,#8460,.T.);
#12016=ORIENTED_EDGE('',*,*,#8457,.T.);
#12017=ORIENTED_EDGE('',*,*,#8454,.T.);
#12018=ORIENTED_EDGE('',*,*,#8451,.T.);
#12019=ORIENTED_EDGE('',*,*,#8448,.T.);
#12020=ORIENTED_EDGE('',*,*,#8441,.T.);
#12021=ORIENTED_EDGE('',*,*,#8477,.T.);
#12022=ORIENTED_EDGE('',*,*,#8438,.F.);
#12023=ORIENTED_EDGE('',*,*,#8476,.T.);
#12024=ORIENTED_EDGE('',*,*,#8363,.F.);
#12025=ORIENTED_EDGE('',*,*,#8479,.T.);
#12026=ORIENTED_EDGE('',*,*,#8392,.T.);
#12027=ORIENTED_EDGE('',*,*,#8480,.T.);
#12028=ORIENTED_EDGE('',*,*,#8366,.F.);
#12029=ORIENTED_EDGE('',*,*,#8412,.T.);
#12030=ORIENTED_EDGE('',*,*,#8481,.T.);
#12031=ORIENTED_EDGE('',*,*,#8409,.F.);
#12032=ORIENTED_EDGE('',*,*,#8482,.F.);
#12033=ORIENTED_EDGE('',*,*,#8480,.F.);
#12034=ORIENTED_EDGE('',*,*,#8391,.F.);
#12035=ORIENTED_EDGE('',*,*,#8395,.F.);
#12036=ORIENTED_EDGE('',*,*,#8398,.F.);
#12037=ORIENTED_EDGE('',*,*,#8401,.F.);
#12038=ORIENTED_EDGE('',*,*,#8404,.F.);
#12039=ORIENTED_EDGE('',*,*,#8407,.F.);
#12040=ORIENTED_EDGE('',*,*,#8410,.F.);
#12041=ORIENTED_EDGE('',*,*,#8481,.F.);
#12042=ORIENTED_EDGE('',*,*,#8415,.F.);
#12043=ORIENTED_EDGE('',*,*,#8483,.F.);
#12044=ORIENTED_EDGE('',*,*,#8387,.F.);
#12045=ORIENTED_EDGE('',*,*,#8484,.F.);
#12046=ORIENTED_EDGE('',*,*,#8385,.F.);
#12047=ORIENTED_EDGE('',*,*,#8382,.F.);
#12048=ORIENTED_EDGE('',*,*,#8379,.F.);
#12049=ORIENTED_EDGE('',*,*,#8376,.F.);
#12050=ORIENTED_EDGE('',*,*,#8373,.F.);
#12051=ORIENTED_EDGE('',*,*,#8370,.F.);
#12052=ORIENTED_EDGE('',*,*,#8367,.F.);
#12053=ORIENTED_EDGE('',*,*,#8479,.F.);
#12054=ORIENTED_EDGE('',*,*,#8362,.F.);
#12055=ORIENTED_EDGE('',*,*,#8369,.F.);
#12056=ORIENTED_EDGE('',*,*,#8372,.F.);
#12057=ORIENTED_EDGE('',*,*,#8375,.F.);
#12058=ORIENTED_EDGE('',*,*,#8378,.F.);
#12059=ORIENTED_EDGE('',*,*,#8381,.F.);
#12060=ORIENTED_EDGE('',*,*,#8384,.F.);
#12061=ORIENTED_EDGE('',*,*,#8485,.F.);
#12062=ORIENTED_EDGE('',*,*,#8389,.F.);
#12063=ORIENTED_EDGE('',*,*,#8486,.F.);
#12064=ORIENTED_EDGE('',*,*,#8413,.T.);
#12065=ORIENTED_EDGE('',*,*,#8482,.T.);
#12066=ORIENTED_EDGE('',*,*,#8411,.T.);
#12067=ORIENTED_EDGE('',*,*,#8408,.T.);
#12068=ORIENTED_EDGE('',*,*,#8405,.T.);
#12069=ORIENTED_EDGE('',*,*,#8402,.T.);
#12070=ORIENTED_EDGE('',*,*,#8399,.T.);
#12071=ORIENTED_EDGE('',*,*,#8396,.T.);
#12072=ORIENTED_EDGE('',*,*,#8393,.T.);
#12073=ORIENTED_EDGE('',*,*,#8386,.T.);
#12074=ORIENTED_EDGE('',*,*,#8485,.T.);
#12075=ORIENTED_EDGE('',*,*,#8383,.F.);
#12076=ORIENTED_EDGE('',*,*,#8484,.T.);
#12077=ORIENTED_EDGE('',*,*,#8308,.F.);
#12078=ORIENTED_EDGE('',*,*,#8487,.T.);
#12079=ORIENTED_EDGE('',*,*,#8337,.T.);
#12080=ORIENTED_EDGE('',*,*,#8488,.T.);
#12081=ORIENTED_EDGE('',*,*,#8311,.F.);
#12082=ORIENTED_EDGE('',*,*,#8357,.T.);
#12083=ORIENTED_EDGE('',*,*,#8489,.T.);
#12084=ORIENTED_EDGE('',*,*,#8354,.F.);
#12085=ORIENTED_EDGE('',*,*,#8490,.F.);
#12086=ORIENTED_EDGE('',*,*,#8488,.F.);
#12087=ORIENTED_EDGE('',*,*,#8336,.F.);
#12088=ORIENTED_EDGE('',*,*,#8340,.F.);
#12089=ORIENTED_EDGE('',*,*,#8343,.F.);
#12090=ORIENTED_EDGE('',*,*,#8346,.F.);
#12091=ORIENTED_EDGE('',*,*,#8349,.F.);
#12092=ORIENTED_EDGE('',*,*,#8352,.F.);
#12093=ORIENTED_EDGE('',*,*,#8355,.F.);
#12094=ORIENTED_EDGE('',*,*,#8489,.F.);
#12095=ORIENTED_EDGE('',*,*,#8360,.F.);
#12096=ORIENTED_EDGE('',*,*,#8491,.F.);
#12097=ORIENTED_EDGE('',*,*,#8332,.F.);
#12098=ORIENTED_EDGE('',*,*,#8492,.F.);
#12099=ORIENTED_EDGE('',*,*,#8330,.F.);
#12100=ORIENTED_EDGE('',*,*,#8327,.F.);
#12101=ORIENTED_EDGE('',*,*,#8324,.F.);
#12102=ORIENTED_EDGE('',*,*,#8321,.F.);
#12103=ORIENTED_EDGE('',*,*,#8318,.F.);
#12104=ORIENTED_EDGE('',*,*,#8315,.F.);
#12105=ORIENTED_EDGE('',*,*,#8312,.F.);
#12106=ORIENTED_EDGE('',*,*,#8487,.F.);
#12107=ORIENTED_EDGE('',*,*,#8307,.F.);
#12108=ORIENTED_EDGE('',*,*,#8314,.F.);
#12109=ORIENTED_EDGE('',*,*,#8317,.F.);
#12110=ORIENTED_EDGE('',*,*,#8320,.F.);
#12111=ORIENTED_EDGE('',*,*,#8323,.F.);
#12112=ORIENTED_EDGE('',*,*,#8326,.F.);
#12113=ORIENTED_EDGE('',*,*,#8329,.F.);
#12114=ORIENTED_EDGE('',*,*,#8493,.F.);
#12115=ORIENTED_EDGE('',*,*,#8334,.F.);
#12116=ORIENTED_EDGE('',*,*,#8494,.F.);
#12117=ORIENTED_EDGE('',*,*,#8358,.T.);
#12118=ORIENTED_EDGE('',*,*,#8490,.T.);
#12119=ORIENTED_EDGE('',*,*,#8356,.T.);
#12120=ORIENTED_EDGE('',*,*,#8353,.T.);
#12121=ORIENTED_EDGE('',*,*,#8350,.T.);
#12122=ORIENTED_EDGE('',*,*,#8347,.T.);
#12123=ORIENTED_EDGE('',*,*,#8344,.T.);
#12124=ORIENTED_EDGE('',*,*,#8341,.T.);
#12125=ORIENTED_EDGE('',*,*,#8338,.T.);
#12126=ORIENTED_EDGE('',*,*,#8331,.T.);
#12127=ORIENTED_EDGE('',*,*,#8493,.T.);
#12128=ORIENTED_EDGE('',*,*,#8328,.F.);
#12129=ORIENTED_EDGE('',*,*,#8492,.T.);
#12130=ORIENTED_EDGE('',*,*,#8365,.F.);
#12131=ORIENTED_EDGE('',*,*,#8420,.F.);
#12132=ORIENTED_EDGE('',*,*,#8310,.F.);
#12133=ORIENTED_EDGE('',*,*,#8495,.F.);
#12134=ORIENTED_EDGE('',*,*,#8496,.F.);
#12135=ORIENTED_EDGE('',*,*,#8496,.T.);
#12136=ORIENTED_EDGE('',*,*,#8497,.F.);
#12137=ORIENTED_EDGE('',*,*,#8498,.T.);
#12138=ORIENTED_EDGE('',*,*,#8499,.T.);
#12139=ORIENTED_EDGE('',*,*,#8498,.F.);
#12140=ORIENTED_EDGE('',*,*,#8497,.T.);
#12141=ORIENTED_EDGE('',*,*,#8478,.T.);
#12142=ORIENTED_EDGE('',*,*,#8443,.T.);
#12143=ORIENTED_EDGE('',*,*,#8475,.T.);
#12144=ORIENTED_EDGE('',*,*,#8469,.T.);
#12145=ORIENTED_EDGE('',*,*,#8486,.T.);
#12146=ORIENTED_EDGE('',*,*,#8388,.T.);
#12147=ORIENTED_EDGE('',*,*,#8483,.T.);
#12148=ORIENTED_EDGE('',*,*,#8414,.T.);
#12149=ORIENTED_EDGE('',*,*,#8494,.T.);
#12150=ORIENTED_EDGE('',*,*,#8333,.T.);
#12151=ORIENTED_EDGE('',*,*,#8491,.T.);
#12152=ORIENTED_EDGE('',*,*,#8359,.T.);
#12153=ORIENTED_EDGE('',*,*,#8495,.T.);
#12154=ORIENTED_EDGE('',*,*,#8499,.F.);
#13508=PLANE('',#15212);
#13509=PLANE('',#15215);
#13510=PLANE('',#15218);
#13511=PLANE('',#15221);
#13512=PLANE('',#15222);
#13513=PLANE('',#15223);
#13514=PLANE('',#15230);
#13515=PLANE('',#15231);
#14014=ADVANCED_FACE('',(#2768),#1938,.F.);
#14015=ADVANCED_FACE('',(#2769),#1939,.F.);
#14016=ADVANCED_FACE('',(#2770),#1940,.F.);
#14017=ADVANCED_FACE('',(#2771),#1941,.F.);
#14018=ADVANCED_FACE('',(#2772),#1942,.F.);
#14019=ADVANCED_FACE('',(#2773),#1943,.F.);
#14020=ADVANCED_FACE('',(#2774),#1944,.F.);
#14021=ADVANCED_FACE('',(#2775),#1945,.F.);
#14022=ADVANCED_FACE('',(#2776),#1946,.F.);
#14023=ADVANCED_FACE('',(#2777),#1947,.F.);
#14024=ADVANCED_FACE('',(#2778),#1948,.F.);
#14025=ADVANCED_FACE('',(#2779),#1949,.F.);
#14026=ADVANCED_FACE('',(#2780),#1950,.F.);
#14027=ADVANCED_FACE('',(#2781),#1951,.F.);
#14028=ADVANCED_FACE('',(#2782),#1952,.F.);
#14029=ADVANCED_FACE('',(#2783),#1953,.F.);
#14030=ADVANCED_FACE('',(#2784),#1954,.F.);
#14031=ADVANCED_FACE('',(#2785),#1955,.F.);
#14032=ADVANCED_FACE('',(#2786),#1956,.F.);
#14033=ADVANCED_FACE('',(#2787),#1957,.F.);
#14034=ADVANCED_FACE('',(#2788),#1958,.F.);
#14035=ADVANCED_FACE('',(#2789),#1959,.F.);
#14036=ADVANCED_FACE('',(#2790),#1960,.F.);
#14037=ADVANCED_FACE('',(#2791),#1961,.F.);
#14038=ADVANCED_FACE('',(#2792),#1962,.F.);
#14039=ADVANCED_FACE('',(#2793),#1963,.F.);
#14040=ADVANCED_FACE('',(#2794),#1964,.F.);
#14041=ADVANCED_FACE('',(#2795),#1965,.F.);
#14042=ADVANCED_FACE('',(#2796),#1966,.F.);
#14043=ADVANCED_FACE('',(#2797),#1967,.F.);
#14044=ADVANCED_FACE('',(#2798),#1968,.F.);
#14045=ADVANCED_FACE('',(#2799),#1969,.F.);
#14046=ADVANCED_FACE('',(#2800),#1970,.F.);
#14047=ADVANCED_FACE('',(#2801),#1971,.F.);
#14048=ADVANCED_FACE('',(#2802),#1972,.F.);
#14049=ADVANCED_FACE('',(#2803),#1973,.F.);
#14050=ADVANCED_FACE('',(#2804),#1974,.F.);
#14051=ADVANCED_FACE('',(#2805),#1975,.F.);
#14052=ADVANCED_FACE('',(#2806),#1976,.F.);
#14053=ADVANCED_FACE('',(#2807),#1977,.F.);
#14054=ADVANCED_FACE('',(#2808),#1978,.F.);
#14055=ADVANCED_FACE('',(#2809),#1979,.F.);
#14056=ADVANCED_FACE('',(#2810),#1980,.F.);
#14057=ADVANCED_FACE('',(#2811),#1981,.F.);
#14058=ADVANCED_FACE('',(#2812),#1982,.F.);
#14059=ADVANCED_FACE('',(#2813),#1983,.F.);
#14060=ADVANCED_FACE('',(#2814),#1984,.F.);
#14061=ADVANCED_FACE('',(#2815),#1985,.F.);
#14062=ADVANCED_FACE('',(#2816),#13508,.T.);
#14063=ADVANCED_FACE('',(#2817),#1986,.F.);
#14064=ADVANCED_FACE('',(#2818),#273,.F.);
#14065=ADVANCED_FACE('',(#2819),#274,.F.);
#14066=ADVANCED_FACE('',(#2820),#1987,.F.);
#14067=ADVANCED_FACE('',(#2821),#13509,.T.);
#14068=ADVANCED_FACE('',(#2822),#1988,.F.);
#14069=ADVANCED_FACE('',(#2823),#275,.F.);
#14070=ADVANCED_FACE('',(#2824),#276,.F.);
#14071=ADVANCED_FACE('',(#2825),#1989,.F.);
#14072=ADVANCED_FACE('',(#2826),#13510,.T.);
#14073=ADVANCED_FACE('',(#2827),#1990,.F.);
#14074=ADVANCED_FACE('',(#2828),#277,.F.);
#14075=ADVANCED_FACE('',(#2829),#278,.F.);
#14076=ADVANCED_FACE('',(#2830),#1991,.F.);
#14077=ADVANCED_FACE('',(#2831),#13511,.F.);
#14078=ADVANCED_FACE('',(#2832),#13512,.F.);
#14079=ADVANCED_FACE('',(#2833),#13513,.F.);
#14080=ADVANCED_FACE('',(#2834),#11,.F.);
#14081=ADVANCED_FACE('',(#2835),#1992,.T.);
#14082=ADVANCED_FACE('',(#2836,#2281,#2282,#2283,#2284),#13514,.T.);
#14083=ADVANCED_FACE('',(#2837),#13515,.F.);
#14318=CLOSED_SHELL('',(#14014,#14015,#14016,#14017,#14018,#14019,#14020,
#14021,#14022,#14023,#14024,#14025,#14026,#14027,#14028,#14029,#14030,#14031,
#14032,#14033,#14034,#14035,#14036,#14037,#14038,#14039,#14040,#14041,#14042,
#14043,#14044,#14045,#14046,#14047,#14048,#14049,#14050,#14051,#14052,#14053,
#14054,#14055,#14056,#14057,#14058,#14059,#14060,#14061,#14062,#14063,#14064,
#14065,#14066,#14067,#14068,#14069,#14070,#14071,#14072,#14073,#14074,#14075,
#14076,#14077,#14078,#14079,#14080,#14081,#14082,#14083));
#15145=AXIS2_PLACEMENT_3D('',#47153,#17353,#17354);
#15146=AXIS2_PLACEMENT_3D('',#47154,#17355,#17356);
#15147=AXIS2_PLACEMENT_3D('',#47164,#17358,#17359);
#15148=AXIS2_PLACEMENT_3D('',#47167,#17361,#17362);
#15149=AXIS2_PLACEMENT_3D('',#47169,#17363,#17364);
#15150=AXIS2_PLACEMENT_3D('',#47180,#17365,#17366);
#15151=AXIS2_PLACEMENT_3D('',#47231,#17368,#17369);
#15152=AXIS2_PLACEMENT_3D('',#47282,#17371,#17372);
#15153=AXIS2_PLACEMENT_3D('',#47330,#17374,#17375);
#15154=AXIS2_PLACEMENT_3D('',#47381,#17377,#17378);
#15155=AXIS2_PLACEMENT_3D('',#47432,#17380,#17381);
#15156=AXIS2_PLACEMENT_3D('',#47480,#17383,#17384);
#15157=AXIS2_PLACEMENT_3D('',#47499,#17386,#17387);
#15158=AXIS2_PLACEMENT_3D('',#47519,#17388,#17389);
#15159=AXIS2_PLACEMENT_3D('',#47533,#17391,#17392);
#15160=AXIS2_PLACEMENT_3D('',#47543,#17393,#17394);
#15161=AXIS2_PLACEMENT_3D('',#47567,#17396,#17397);
#15162=AXIS2_PLACEMENT_3D('',#47592,#17399,#17400);
#15163=AXIS2_PLACEMENT_3D('',#47617,#17402,#17403);
#15164=AXIS2_PLACEMENT_3D('',#47641,#17405,#17406);
#15165=AXIS2_PLACEMENT_3D('',#47666,#17408,#17409);
#15166=AXIS2_PLACEMENT_3D('',#47691,#17411,#17412);
#15167=AXIS2_PLACEMENT_3D('',#47702,#17414,#17415);
#15168=AXIS2_PLACEMENT_3D('',#47708,#17416,#17417);
#15169=AXIS2_PLACEMENT_3D('',#47718,#17419,#17420);
#15170=AXIS2_PLACEMENT_3D('',#47721,#17422,#17423);
#15171=AXIS2_PLACEMENT_3D('',#47723,#17424,#17425);
#15172=AXIS2_PLACEMENT_3D('',#47734,#17426,#17427);
#15173=AXIS2_PLACEMENT_3D('',#47785,#17429,#17430);
#15174=AXIS2_PLACEMENT_3D('',#47836,#17432,#17433);
#15175=AXIS2_PLACEMENT_3D('',#47884,#17435,#17436);
#15176=AXIS2_PLACEMENT_3D('',#47935,#17438,#17439);
#15177=AXIS2_PLACEMENT_3D('',#47986,#17441,#17442);
#15178=AXIS2_PLACEMENT_3D('',#48034,#17444,#17445);
#15179=AXIS2_PLACEMENT_3D('',#48053,#17447,#17448);
#15180=AXIS2_PLACEMENT_3D('',#48073,#17449,#17450);
#15181=AXIS2_PLACEMENT_3D('',#48087,#17452,#17453);
#15182=AXIS2_PLACEMENT_3D('',#48097,#17454,#17455);
#15183=AXIS2_PLACEMENT_3D('',#48121,#17457,#17458);
#15184=AXIS2_PLACEMENT_3D('',#48146,#17460,#17461);
#15185=AXIS2_PLACEMENT_3D('',#48171,#17463,#17464);
#15186=AXIS2_PLACEMENT_3D('',#48195,#17466,#17467);
#15187=AXIS2_PLACEMENT_3D('',#48220,#17469,#17470);
#15188=AXIS2_PLACEMENT_3D('',#48245,#17472,#17473);
#15189=AXIS2_PLACEMENT_3D('',#48256,#17475,#17476);
#15190=AXIS2_PLACEMENT_3D('',#48262,#17477,#17478);
#15191=AXIS2_PLACEMENT_3D('',#48272,#17480,#17481);
#15192=AXIS2_PLACEMENT_3D('',#48275,#17483,#17484);
#15193=AXIS2_PLACEMENT_3D('',#48277,#17485,#17486);
#15194=AXIS2_PLACEMENT_3D('',#48288,#17487,#17488);
#15195=AXIS2_PLACEMENT_3D('',#48339,#17490,#17491);
#15196=AXIS2_PLACEMENT_3D('',#48390,#17493,#17494);
#15197=AXIS2_PLACEMENT_3D('',#48438,#17496,#17497);
#15198=AXIS2_PLACEMENT_3D('',#48489,#17499,#17500);
#15199=AXIS2_PLACEMENT_3D('',#48540,#17502,#17503);
#15200=AXIS2_PLACEMENT_3D('',#48588,#17505,#17506);
#15201=AXIS2_PLACEMENT_3D('',#48607,#17508,#17509);
#15202=AXIS2_PLACEMENT_3D('',#48627,#17510,#17511);
#15203=AXIS2_PLACEMENT_3D('',#48641,#17513,#17514);
#15204=AXIS2_PLACEMENT_3D('',#48651,#17515,#17516);
#15205=AXIS2_PLACEMENT_3D('',#48675,#17518,#17519);
#15206=AXIS2_PLACEMENT_3D('',#48700,#17521,#17522);
#15207=AXIS2_PLACEMENT_3D('',#48725,#17524,#17525);
#15208=AXIS2_PLACEMENT_3D('',#48749,#17527,#17528);
#15209=AXIS2_PLACEMENT_3D('',#48774,#17530,#17531);
#15210=AXIS2_PLACEMENT_3D('',#48799,#17533,#17534);
#15211=AXIS2_PLACEMENT_3D('',#48810,#17536,#17537);
#15212=AXIS2_PLACEMENT_3D('',#48816,#17538,#17539);
#15213=AXIS2_PLACEMENT_3D('',#49008,#17540,#17541);
#15214=AXIS2_PLACEMENT_3D('',#49707,#17542,#17543);
#15215=AXIS2_PLACEMENT_3D('',#49708,#17544,#17545);
#15216=AXIS2_PLACEMENT_3D('',#49900,#17546,#17547);
#15217=AXIS2_PLACEMENT_3D('',#50599,#17548,#17549);
#15218=AXIS2_PLACEMENT_3D('',#50600,#17550,#17551);
#15219=AXIS2_PLACEMENT_3D('',#50792,#17552,#17553);
#15220=AXIS2_PLACEMENT_3D('',#51491,#17554,#17555);
#15221=AXIS2_PLACEMENT_3D('',#51492,#17556,#17557);
#15222=AXIS2_PLACEMENT_3D('',#51493,#17558,#17559);
#15223=AXIS2_PLACEMENT_3D('',#51494,#17560,#17561);
#15224=AXIS2_PLACEMENT_3D('',#51495,#17562,#17563);
#15225=AXIS2_PLACEMENT_3D('',#51497,#17564,#17565);
#15226=AXIS2_PLACEMENT_3D('',#51499,#17566,#17567);
#15227=AXIS2_PLACEMENT_3D('',#51500,#17568,#17569);
#15228=AXIS2_PLACEMENT_3D('',#51502,#17570,#17571);
#15229=AXIS2_PLACEMENT_3D('',#51505,#17573,#17574);
#15230=AXIS2_PLACEMENT_3D('',#51506,#17575,#17576);
#15231=AXIS2_PLACEMENT_3D('',#51507,#17577,#17578);
#17353=DIRECTION('axis',(0.,0.,1.));
#17354=DIRECTION('refdir',(1.,0.,0.));
#17355=DIRECTION('center_axis',(0.,0.,-1.));
#17356=DIRECTION('ref_axis',(1.,0.,0.));
#17357=DIRECTION('',(0.,0.,-1.));
#17358=DIRECTION('center_axis',(0.,0.,1.));
#17359=DIRECTION('ref_axis',(1.,0.,0.));
#17360=DIRECTION('',(0.,0.,-1.));
#17361=DIRECTION('center_axis',(0.,0.,1.));
#17362=DIRECTION('ref_axis',(1.,0.,0.));
#17363=DIRECTION('center_axis',(0.,0.,1.));
#17364=DIRECTION('ref_axis',(1.,0.,0.));
#17365=DIRECTION('center_axis',(0.,0.,-1.));
#17366=DIRECTION('ref_axis',(1.,0.,0.));
#17367=DIRECTION('',(0.,0.,-1.));
#17368=DIRECTION('center_axis',(0.,0.,-1.));
#17369=DIRECTION('ref_axis',(1.,0.,0.));
#17370=DIRECTION('',(0.,0.,-1.));
#17371=DIRECTION('center_axis',(0.,0.,-1.));
#17372=DIRECTION('ref_axis',(1.,0.,0.));
#17373=DIRECTION('',(0.,0.,-1.));
#17374=DIRECTION('center_axis',(0.,0.,-1.));
#17375=DIRECTION('ref_axis',(1.,0.,0.));
#17376=DIRECTION('',(0.,0.,-1.));
#17377=DIRECTION('center_axis',(0.,0.,-1.));
#17378=DIRECTION('ref_axis',(1.,0.,0.));
#17379=DIRECTION('',(0.,0.,-1.));
#17380=DIRECTION('center_axis',(0.,0.,-1.));
#17381=DIRECTION('ref_axis',(1.,0.,0.));
#17382=DIRECTION('',(0.,0.,-1.));
#17383=DIRECTION('center_axis',(0.,0.,-1.));
#17384=DIRECTION('ref_axis',(0.937998542404131,-0.346639199237082,0.));
#17385=DIRECTION('',(0.,0.,-1.));
#17386=DIRECTION('center_axis',(0.,0.,-1.));
#17387=DIRECTION('ref_axis',(1.,0.,0.));
#17388=DIRECTION('center_axis',(0.,0.,-1.));
#17389=DIRECTION('ref_axis',(0.793234457633775,0.608916328589118,0.));
#17390=DIRECTION('',(1.22464679914735E-16,-2.66923102573661E-30,-1.));
#17391=DIRECTION('center_axis',(0.,0.,1.));
#17392=DIRECTION('ref_axis',(1.,-2.16734607052251E-14,0.));
#17393=DIRECTION('center_axis',(0.,0.,-1.));
#17394=DIRECTION('ref_axis',(1.,-2.16734607052251E-14,0.));
#17395=DIRECTION('',(1.22464679914735E-16,-2.66923102573661E-30,-1.));
#17396=DIRECTION('center_axis',(0.,0.,-1.));
#17397=DIRECTION('ref_axis',(1.,-2.16734607052251E-14,0.));
#17398=DIRECTION('',(1.22464679914735E-16,-2.66923102573661E-30,-1.));
#17399=DIRECTION('center_axis',(0.,0.,-1.));
#17400=DIRECTION('ref_axis',(1.,-2.16734607052251E-14,0.));
#17401=DIRECTION('',(1.22464679914735E-16,-2.66923102573661E-30,-1.));
#17402=DIRECTION('center_axis',(0.,0.,-1.));
#17403=DIRECTION('ref_axis',(1.,-2.16734607052251E-14,0.));
#17404=DIRECTION('',(1.22464679914735E-16,-2.66923102573661E-30,-1.));
#17405=DIRECTION('center_axis',(0.,0.,-1.));
#17406=DIRECTION('ref_axis',(1.,-2.16734607052251E-14,0.));
#17407=DIRECTION('',(1.22464679914735E-16,-2.66923102573661E-30,-1.));
#17408=DIRECTION('center_axis',(0.,0.,-1.));
#17409=DIRECTION('ref_axis',(1.,-2.16734607052251E-14,0.));
#17410=DIRECTION('',(1.22464679914735E-16,-2.66923102573661E-30,-1.));
#17411=DIRECTION('center_axis',(0.,0.,-1.));
#17412=DIRECTION('ref_axis',(-0.609099265708522,-0.793093994753042,0.));
#17413=DIRECTION('',(1.22464679914735E-16,-2.66923102573661E-30,-1.));
#17414=DIRECTION('center_axis',(0.,0.,-1.));
#17415=DIRECTION('ref_axis',(1.,-2.16734607052251E-14,0.));
#17416=DIRECTION('center_axis',(0.,0.,-1.));
#17417=DIRECTION('ref_axis',(1.,0.,0.));
#17418=DIRECTION('',(0.,0.,-1.));
#17419=DIRECTION('center_axis',(0.,0.,1.));
#17420=DIRECTION('ref_axis',(1.,0.,0.));
#17421=DIRECTION('',(0.,0.,-1.));
#17422=DIRECTION('center_axis',(0.,0.,1.));
#17423=DIRECTION('ref_axis',(1.,0.,0.));
#17424=DIRECTION('center_axis',(0.,0.,1.));
#17425=DIRECTION('ref_axis',(1.,0.,0.));
#17426=DIRECTION('center_axis',(0.,0.,-1.));
#17427=DIRECTION('ref_axis',(1.,0.,0.));
#17428=DIRECTION('',(0.,0.,-1.));
#17429=DIRECTION('center_axis',(0.,0.,-1.));
#17430=DIRECTION('ref_axis',(1.,0.,0.));
#17431=DIRECTION('',(0.,0.,-1.));
#17432=DIRECTION('center_axis',(0.,0.,-1.));
#17433=DIRECTION('ref_axis',(1.,0.,0.));
#17434=DIRECTION('',(0.,0.,-1.));
#17435=DIRECTION('center_axis',(0.,0.,-1.));
#17436=DIRECTION('ref_axis',(1.,0.,0.));
#17437=DIRECTION('',(0.,0.,-1.));
#17438=DIRECTION('center_axis',(0.,0.,-1.));
#17439=DIRECTION('ref_axis',(1.,0.,0.));
#17440=DIRECTION('',(0.,0.,-1.));
#17441=DIRECTION('center_axis',(0.,0.,-1.));
#17442=DIRECTION('ref_axis',(1.,0.,0.));
#17443=DIRECTION('',(0.,0.,-1.));
#17444=DIRECTION('center_axis',(0.,0.,-1.));
#17445=DIRECTION('ref_axis',(0.937998514609972,-0.346639274447495,0.));
#17446=DIRECTION('',(0.,0.,-1.));
#17447=DIRECTION('center_axis',(0.,0.,-1.));
#17448=DIRECTION('ref_axis',(1.,0.,0.));
#17449=DIRECTION('center_axis',(0.,0.,-1.));
#17450=DIRECTION('ref_axis',(0.793234421148473,0.608916376118468,0.));
#17451=DIRECTION('',(1.22464679914735E-16,-2.66923102573661E-30,-1.));
#17452=DIRECTION('center_axis',(0.,0.,1.));
#17453=DIRECTION('ref_axis',(1.,-2.16734607052251E-14,0.));
#17454=DIRECTION('center_axis',(0.,0.,-1.));
#17455=DIRECTION('ref_axis',(1.,-2.16734607052251E-14,0.));
#17456=DIRECTION('',(1.22464679914735E-16,-2.66923102573661E-30,-1.));
#17457=DIRECTION('center_axis',(0.,0.,-1.));
#17458=DIRECTION('ref_axis',(1.,-2.16734607052251E-14,0.));
#17459=DIRECTION('',(1.22464679914735E-16,-2.66923102573661E-30,-1.));
#17460=DIRECTION('center_axis',(0.,0.,-1.));
#17461=DIRECTION('ref_axis',(1.,-2.16734607052251E-14,0.));
#17462=DIRECTION('',(1.22464679914735E-16,-2.66923102573661E-30,-1.));
#17463=DIRECTION('center_axis',(0.,0.,-1.));
#17464=DIRECTION('ref_axis',(1.,-2.16734607052251E-14,0.));
#17465=DIRECTION('',(1.22464679914735E-16,-2.66923102573661E-30,-1.));
#17466=DIRECTION('center_axis',(0.,0.,-1.));
#17467=DIRECTION('ref_axis',(1.,-2.16734607052251E-14,0.));
#17468=DIRECTION('',(1.22464679914735E-16,-2.66923102573661E-30,-1.));
#17469=DIRECTION('center_axis',(0.,0.,-1.));
#17470=DIRECTION('ref_axis',(1.,-2.16734607052251E-14,0.));
#17471=DIRECTION('',(1.22464679914735E-16,-2.66923102573661E-30,-1.));
#17472=DIRECTION('center_axis',(0.,0.,-1.));
#17473=DIRECTION('ref_axis',(-0.609099316811134,-0.793093955506036,0.));
#17474=DIRECTION('',(1.22464679914735E-16,-2.66923102573661E-30,-1.));
#17475=DIRECTION('center_axis',(0.,0.,-1.));
#17476=DIRECTION('ref_axis',(1.,-2.16734607052251E-14,0.));
#17477=DIRECTION('center_axis',(0.,0.,-1.));
#17478=DIRECTION('ref_axis',(1.,0.,0.));
#17479=DIRECTION('',(0.,0.,-1.));
#17480=DIRECTION('center_axis',(0.,0.,1.));
#17481=DIRECTION('ref_axis',(1.,0.,0.));
#17482=DIRECTION('',(0.,0.,-1.));
#17483=DIRECTION('center_axis',(0.,0.,1.));
#17484=DIRECTION('ref_axis',(1.,0.,0.));
#17485=DIRECTION('center_axis',(0.,0.,1.));
#17486=DIRECTION('ref_axis',(1.,0.,0.));
#17487=DIRECTION('center_axis',(0.,0.,-1.));
#17488=DIRECTION('ref_axis',(1.,0.,0.));
#17489=DIRECTION('',(0.,0.,-1.));
#17490=DIRECTION('center_axis',(0.,0.,-1.));
#17491=DIRECTION('ref_axis',(1.,0.,0.));
#17492=DIRECTION('',(0.,0.,-1.));
#17493=DIRECTION('center_axis',(0.,0.,-1.));
#17494=DIRECTION('ref_axis',(1.,0.,0.));
#17495=DIRECTION('',(0.,0.,-1.));
#17496=DIRECTION('center_axis',(0.,0.,-1.));
#17497=DIRECTION('ref_axis',(1.,0.,0.));
#17498=DIRECTION('',(0.,0.,-1.));
#17499=DIRECTION('center_axis',(0.,0.,-1.));
#17500=DIRECTION('ref_axis',(1.,0.,0.));
#17501=DIRECTION('',(0.,0.,-1.));
#17502=DIRECTION('center_axis',(0.,0.,-1.));
#17503=DIRECTION('ref_axis',(1.,0.,0.));
#17504=DIRECTION('',(0.,0.,-1.));
#17505=DIRECTION('center_axis',(0.,0.,-1.));
#17506=DIRECTION('ref_axis',(0.937997876463511,-0.346641001253376,0.));
#17507=DIRECTION('',(0.,0.,-1.));
#17508=DIRECTION('center_axis',(0.,0.,-1.));
#17509=DIRECTION('ref_axis',(1.,0.,0.));
#17510=DIRECTION('center_axis',(0.,0.,-1.));
#17511=DIRECTION('ref_axis',(0.793233502010203,0.608917573476599,0.));
#17512=DIRECTION('',(1.22464679914735E-16,-2.67208401572961E-30,-1.));
#17513=DIRECTION('center_axis',(0.,0.,1.));
#17514=DIRECTION('ref_axis',(1.,-2.16967571364491E-14,0.));
#17515=DIRECTION('center_axis',(0.,0.,-1.));
#17516=DIRECTION('ref_axis',(1.,-2.16967571364491E-14,0.));
#17517=DIRECTION('',(1.22464679914735E-16,-2.67208401572961E-30,-1.));
#17518=DIRECTION('center_axis',(0.,0.,-1.));
#17519=DIRECTION('ref_axis',(1.,-2.16967571364491E-14,0.));
#17520=DIRECTION('',(1.22464679914735E-16,-2.67208401572961E-30,-1.));
#17521=DIRECTION('center_axis',(0.,0.,-1.));
#17522=DIRECTION('ref_axis',(1.,-2.16967571364491E-14,0.));
#17523=DIRECTION('',(1.22464679914735E-16,-2.67208401572961E-30,-1.));
#17524=DIRECTION('center_axis',(0.,0.,-1.));
#17525=DIRECTION('ref_axis',(1.,-2.16967571364491E-14,0.));
#17526=DIRECTION('',(1.22464679914735E-16,-2.67208401572961E-30,-1.));
#17527=DIRECTION('center_axis',(0.,0.,-1.));
#17528=DIRECTION('ref_axis',(1.,-2.16967571364491E-14,0.));
#17529=DIRECTION('',(1.22464679914735E-16,-2.67208401572961E-30,-1.));
#17530=DIRECTION('center_axis',(0.,0.,-1.));
#17531=DIRECTION('ref_axis',(1.,-2.16967571364491E-14,0.));
#17532=DIRECTION('',(1.22464679914735E-16,-2.67208401572961E-30,-1.));
#17533=DIRECTION('center_axis',(0.,0.,-1.));
#17534=DIRECTION('ref_axis',(-0.609100172155653,-0.793093298597305,0.));
#17535=DIRECTION('',(1.22464679914735E-16,-2.67208401572961E-30,-1.));
#17536=DIRECTION('center_axis',(0.,0.,-1.));
#17537=DIRECTION('ref_axis',(1.,-2.16967571364491E-14,0.));
#17538=DIRECTION('center_axis',(0.,0.,1.));
#17539=DIRECTION('ref_axis',(1.,0.,0.));
#17540=DIRECTION('center_axis',(0.,0.,-1.));
#17541=DIRECTION('ref_axis',(1.,-2.16967571364491E-14,0.));
#17542=DIRECTION('center_axis',(0.,0.,-1.));
#17543=DIRECTION('ref_axis',(1.,0.,0.));
#17544=DIRECTION('center_axis',(0.,0.,1.));
#17545=DIRECTION('ref_axis',(1.,0.,0.));
#17546=DIRECTION('center_axis',(0.,0.,-1.));
#17547=DIRECTION('ref_axis',(1.,-2.16734607052251E-14,0.));
#17548=DIRECTION('center_axis',(0.,0.,-1.));
#17549=DIRECTION('ref_axis',(1.,0.,0.));
#17550=DIRECTION('center_axis',(0.,0.,1.));
#17551=DIRECTION('ref_axis',(1.,0.,0.));
#17552=DIRECTION('center_axis',(0.,0.,-1.));
#17553=DIRECTION('ref_axis',(1.,-2.16734607052251E-14,0.));
#17554=DIRECTION('center_axis',(0.,0.,-1.));
#17555=DIRECTION('ref_axis',(1.,0.,0.));
#17556=DIRECTION('center_axis',(0.,0.,-1.));
#17557=DIRECTION('ref_axis',(1.,0.,0.));
#17558=DIRECTION('center_axis',(0.,0.,-1.));
#17559=DIRECTION('ref_axis',(1.,0.,0.));
#17560=DIRECTION('center_axis',(0.,0.,-1.));
#17561=DIRECTION('ref_axis',(1.,0.,0.));
#17562=DIRECTION('center_axis',(6.12323399573677E-17,0.,1.));
#17563=DIRECTION('ref_axis',(1.,0.,0.));
#17564=DIRECTION('center_axis',(0.,0.,-1.));
#17565=DIRECTION('ref_axis',(0.,1.,0.));
#17566=DIRECTION('center_axis',(-1.22464679914735E-16,1.,0.));
#17567=DIRECTION('ref_axis',(-1.,-1.22464679914735E-16,0.));
#17568=DIRECTION('center_axis',(0.,0.,1.));
#17569=DIRECTION('ref_axis',(1.,0.,0.));
#17570=DIRECTION('center_axis',(0.,0.,1.));
#17571=DIRECTION('ref_axis',(1.,0.,0.));
#17572=DIRECTION('',(0.,0.,-1.));
#17573=DIRECTION('center_axis',(0.,0.,1.));
#17574=DIRECTION('ref_axis',(1.,0.,0.));
#17575=DIRECTION('center_axis',(0.,0.,1.));
#17576=DIRECTION('ref_axis',(1.,0.,0.));
#17577=DIRECTION('center_axis',(0.,0.,1.));
#17578=DIRECTION('ref_axis',(1.,0.,0.));
#47153=CARTESIAN_POINT('',(0.,0.,0.));
#47154=CARTESIAN_POINT('Origin',(-7.50000000000001,-12.9903810567666,7.5));
#47155=CARTESIAN_POINT('',(-10.0135514395051,-12.9904666377399,4.38741669750803));
#47156=CARTESIAN_POINT('',(-10.0159862278212,-12.9935669321582,4.11258330249198));
#47157=CARTESIAN_POINT('',(-10.0175,-12.9903810567666,7.5));
#47158=CARTESIAN_POINT('',(-9.41346599666503,-11.3543938533916,4.));
#47159=CARTESIAN_POINT('Ctrl Pts',(-10.0159862278212,-12.9935669321582,
4.11258330249198));
#47160=CARTESIAN_POINT('Ctrl Pts',(-10.0108023762528,-12.4010697429433,
4.07505553499466));
#47161=CARTESIAN_POINT('Ctrl Pts',(-9.79922182808404,-11.8055774964621,
4.03752776749733));
#47162=CARTESIAN_POINT('Ctrl Pts',(-9.41346599666503,-11.3543938533916,
4.));
#47163=CARTESIAN_POINT('',(-10.0175,-12.9903810567666,4.));
#47164=CARTESIAN_POINT('Origin',(-7.50000000000001,-12.9903810567666,4.));
#47165=CARTESIAN_POINT('',(-10.0175,-12.9903810567666,3.));
#47166=CARTESIAN_POINT('',(-10.0175,-12.9903810567666,7.5));
#47167=CARTESIAN_POINT('Origin',(-7.50000000000001,-12.9903810567666,3.));
#47168=CARTESIAN_POINT('',(-5.58300636833058,-11.3520706988407,4.));
#47169=CARTESIAN_POINT('Origin',(-7.50000000000001,-12.9903810567666,4.));
#47170=CARTESIAN_POINT('Ctrl Pts',(-5.58299257280548,-11.3520616136783,
4.));
#47171=CARTESIAN_POINT('Ctrl Pts',(-6.09671565847252,-10.7549231085896,
4.04999787746244));
#47172=CARTESIAN_POINT('Ctrl Pts',(-6.91408826359173,-10.4146529403296,
4.09999575492489));
#47173=CARTESIAN_POINT('Ctrl Pts',(-7.6991792943871,-10.4769907523554,4.14999363238733));
#47174=CARTESIAN_POINT('Ctrl Pts',(-8.52094345767964,-10.5422404851016,
4.20232700817142));
#47175=CARTESIAN_POINT('Ctrl Pts',(-9.30733973752043,-11.0485898984475,
4.2546603839555));
#47176=CARTESIAN_POINT('Ctrl Pts',(-9.70625816906456,-11.7696982113955,
4.30699375973958));
#47177=CARTESIAN_POINT('Ctrl Pts',(-9.91060317652291,-12.1390842109776,
4.3338014056624));
#47178=CARTESIAN_POINT('Ctrl Pts',(-10.0132749267868,-12.5648224302545,
4.36060905158521));
#47179=CARTESIAN_POINT('Ctrl Pts',(-10.0135514395051,-12.9904666377399,
4.38741669750803));
#47180=CARTESIAN_POINT('Origin',(-7.50000000000001,-12.9903810567666,7.5));
#47181=CARTESIAN_POINT('',(-10.0201378128903,-12.991921413328,5.38741669750803));
#47182=CARTESIAN_POINT('',(-10.020701946345,-12.9891728119784,5.11258330249198));
#47183=CARTESIAN_POINT('',(-10.0175,-12.9903810567666,7.5));
#47184=CARTESIAN_POINT('Ctrl Pts',(-10.020701946345,-12.9891728119784,5.11258330249198));
#47185=CARTESIAN_POINT('Ctrl Pts',(-10.0211241641948,-12.9178130461518,
5.10805583214991));
#47186=CARTESIAN_POINT('Ctrl Pts',(-10.0183502770585,-12.846486861832,5.10352836180784));
#47187=CARTESIAN_POINT('Ctrl Pts',(-10.0122725294143,-12.775443667658,5.09900089146577));
#47188=CARTESIAN_POINT('Ctrl Pts',(-9.94201937978509,-11.9542499553417,
5.04666751568169));
#47189=CARTESIAN_POINT('Ctrl Pts',(-9.43032999980707,-11.170867192649,4.99433413989761));
#47190=CARTESIAN_POINT('Ctrl Pts',(-8.70662199025935,-10.7764184817432,
4.94200076411352));
#47191=CARTESIAN_POINT('Ctrl Pts',(-7.98291398071162,-10.3819697708373,
4.88966738832944));
#47192=CARTESIAN_POINT('Ctrl Pts',(-7.04718734159418,-10.3764551117184,
4.83733401254535));
#47193=CARTESIAN_POINT('Ctrl Pts',(-6.31898112841336,-10.7625629528365,
4.78500063676127));
#47194=CARTESIAN_POINT('Ctrl Pts',(-5.59077491523255,-11.1486707939545,
4.73266726097718));
#47195=CARTESIAN_POINT('Ctrl Pts',(-5.07008912798835,-11.9264011353096,
4.6803338851931));
#47196=CARTESIAN_POINT('Ctrl Pts',(-4.99037287718051,-12.7466319075856,
4.62800050940901));
#47197=CARTESIAN_POINT('Ctrl Pts',(-4.91065662637267,-13.5668626798615,
4.57566713362493));
#47198=CARTESIAN_POINT('Ctrl Pts',(-5.27190991200121,-14.4295938830583,
4.52333375784085));
#47199=CARTESIAN_POINT('Ctrl Pts',(-5.9121672709983,-14.948847615037,4.47100038205676));
#47200=CARTESIAN_POINT('Ctrl Pts',(-6.55242462999539,-15.4681013470158,
4.41866700627267));
#47201=CARTESIAN_POINT('Ctrl Pts',(-7.47168606236103,-15.6438776077765,
4.36633363048859));
#47202=CARTESIAN_POINT('Ctrl Pts',(-8.25780335304795,-15.3956944886946,
4.31400025470451));
#47203=CARTESIAN_POINT('Ctrl Pts',(-9.04392064373486,-15.1475113696128,
4.26166687892042));
#47204=CARTESIAN_POINT('Ctrl Pts',(-9.69689379274305,-14.4753688706883,
4.20933350313634));
#47205=CARTESIAN_POINT('Ctrl Pts',(-9.92376658082896,-13.6843861063472,
4.15700012735226));
#47206=CARTESIAN_POINT('Ctrl Pts',(-9.98795104401328,-13.460609581425,4.1421945190655));
#47207=CARTESIAN_POINT('Ctrl Pts',(-10.0180313821391,-13.2273213460105,
4.12738891077874));
#47208=CARTESIAN_POINT('Ctrl Pts',(-10.0159862278212,-12.9935669321582,
4.11258330249198));
#47209=CARTESIAN_POINT('Ctrl Pts',(-10.0135514395051,-12.9904666377399,
4.38741669750803));
#47210=CARTESIAN_POINT('Ctrl Pts',(-10.013814729649,-13.3957569451608,4.41294242736929));
#47211=CARTESIAN_POINT('Ctrl Pts',(-9.92124152424158,-13.8009620169255,
4.43846815723057));
#47212=CARTESIAN_POINT('Ctrl Pts',(-9.73520854233975,-14.1573521883653,
4.46399388709184));
#47213=CARTESIAN_POINT('Ctrl Pts',(-9.35379990082332,-14.8880306398367,
4.51632726287592));
#47214=CARTESIAN_POINT('Ctrl Pts',(-8.57954203454297,-15.4135203302294,
4.56866063866001));
#47215=CARTESIAN_POINT('Ctrl Pts',(-7.75970075309617,-15.4983926191754,
4.62099401444409));
#47216=CARTESIAN_POINT('Ctrl Pts',(-6.93985947164937,-15.5832649081213,
4.67332739022818));
#47217=CARTESIAN_POINT('Ctrl Pts',(-6.07443477503611,-15.2275197956205,
4.72566076601226));
#47218=CARTESIAN_POINT('Ctrl Pts',(-5.5513808289996,-14.5905667824841,4.77799414179634));
#47219=CARTESIAN_POINT('Ctrl Pts',(-5.02832688296309,-13.9536137693476,
4.83032751758043));
#47220=CARTESIAN_POINT('Ctrl Pts',(-4.84764368750334,-13.0354528555755,
4.88266089336451));
#47221=CARTESIAN_POINT('Ctrl Pts',(-5.09037368993613,-12.2477921509444,
4.93499426914859));
#47222=CARTESIAN_POINT('Ctrl Pts',(-5.33310369236891,-11.4601314463133,
4.98732764493268));
#47223=CARTESIAN_POINT('Ctrl Pts',(-5.99924689269421,-10.8029709508232,
5.03966102071677));
#47224=CARTESIAN_POINT('Ctrl Pts',(-6.79011830096555,-10.5709280850384,
5.09199439650085));
#47225=CARTESIAN_POINT('Ctrl Pts',(-7.58098970923688,-10.3388852192536,
5.14432777228494));
#47226=CARTESIAN_POINT('Ctrl Pts',(-8.49658932545427,-10.5319599831741,
5.19666114806902));
#47227=CARTESIAN_POINT('Ctrl Pts',(-9.1264120969476,-11.0635984608226,5.2489945238531));
#47228=CARTESIAN_POINT('Ctrl Pts',(-9.68170742388623,-11.532327721848,5.29513524840475));
#47229=CARTESIAN_POINT('Ctrl Pts',(-10.0148568228205,-12.2642362843572,
5.34127597295639));
#47230=CARTESIAN_POINT('Ctrl Pts',(-10.0201378128903,-12.991921413328,5.38741669750803));
#47231=CARTESIAN_POINT('Origin',(-7.50000000000001,-12.9903810567666,7.5));
#47232=CARTESIAN_POINT('',(-10.0170829580245,-12.9882144302548,6.38741669750803));
#47233=CARTESIAN_POINT('',(-10.0137189064297,-12.9898141627747,6.11258330249198));
#47234=CARTESIAN_POINT('',(-10.0175,-12.9903810567666,7.5));
#47235=CARTESIAN_POINT('Ctrl Pts',(-10.0137189064297,-12.9898141627747,
6.11258330249198));
#47236=CARTESIAN_POINT('Ctrl Pts',(-10.0144984482212,-12.6110466544282,
6.08872275352109));
#47237=CARTESIAN_POINT('Ctrl Pts',(-9.93406605373638,-12.2325935036327,
6.06486220455019));
#47238=CARTESIAN_POINT('Ctrl Pts',(-9.77069376862533,-11.8941805898436,
6.04100165557929));
#47239=CARTESIAN_POINT('Ctrl Pts',(-9.41236910476912,-11.151939067693,5.98866827979521));
#47240=CARTESIAN_POINT('Ctrl Pts',(-8.65505620083081,-10.6023139521363,
5.93633490401113));
#47241=CARTESIAN_POINT('Ctrl Pts',(-7.83829991591844,-10.4917303363644,
5.88400152822705));
#47242=CARTESIAN_POINT('Ctrl Pts',(-7.02154363100607,-10.3811467205925,
5.83166815244296));
#47243=CARTESIAN_POINT('Ctrl Pts',(-6.14534396511963,-10.7096046046056,
5.77933477665887));
#47244=CARTESIAN_POINT('Ctrl Pts',(-5.60254926887142,-11.3298421637022,
5.72700140087479));
#47245=CARTESIAN_POINT('Ctrl Pts',(-5.05975457262321,-11.9500797227988,
5.6746680250907));
#47246=CARTESIAN_POINT('Ctrl Pts',(-4.8503648460132,-12.862096956979,5.62233464930662));
#47247=CARTESIAN_POINT('Ctrl Pts',(-5.06826092360056,-13.6569790435728,
5.57000127352254));
#47248=CARTESIAN_POINT('Ctrl Pts',(-5.28615700118792,-14.4518611301666,
5.51766789773845));
#47249=CARTESIAN_POINT('Ctrl Pts',(-5.93133888297262,-15.129608069174,5.46533452195437));
#47250=CARTESIAN_POINT('Ctrl Pts',(-6.71453628267279,-15.3863634879565,
5.41300114617028));
#47251=CARTESIAN_POINT('Ctrl Pts',(-7.49773368237297,-15.6431189067389,
5.3606677703862));
#47252=CARTESIAN_POINT('Ctrl Pts',(-8.41894659998862,-15.4788828052965,
5.30833439460211));
#47253=CARTESIAN_POINT('Ctrl Pts',(-9.06514459915626,-14.9672624236053,
5.25600101881803));
#47254=CARTESIAN_POINT('Ctrl Pts',(-9.65543865112952,-14.4999033965431,
5.20819511337601));
#47255=CARTESIAN_POINT('Ctrl Pts',(-10.0162437157927,-13.7426660344013,
5.160389207934));
#47256=CARTESIAN_POINT('Ctrl Pts',(-10.020701946345,-12.9891728119784,5.11258330249198));
#47257=CARTESIAN_POINT('Ctrl Pts',(-10.0201378128903,-12.991921413328,5.38741669750803));
#47258=CARTESIAN_POINT('Ctrl Pts',(-10.0208465865384,-13.0895856839813,
5.39360934874047));
#47259=CARTESIAN_POINT('Ctrl Pts',(-10.0156494886519,-13.1871738782112,
5.39980199997292));
#47260=CARTESIAN_POINT('Ctrl Pts',(-10.004290929159,-13.2840395347951,5.40599465120536));
#47261=CARTESIAN_POINT('Ctrl Pts',(-9.90830106310784,-14.1026399397423,
5.45832802698944));
#47262=CARTESIAN_POINT('Ctrl Pts',(-9.37227540423617,-14.8696385582602,
5.51066140277353));
#47263=CARTESIAN_POINT('Ctrl Pts',(-8.63654582863995,-15.2411510354214,
5.56299477855761));
#47264=CARTESIAN_POINT('Ctrl Pts',(-7.90081625304375,-15.6126635125827,
5.61532815434169));
#47265=CARTESIAN_POINT('Ctrl Pts',(-6.96538276072302,-15.5886898483873,
5.66766153012578));
#47266=CARTESIAN_POINT('Ctrl Pts',(-6.24965032039424,-15.1799771379828,
5.71999490590986));
#47267=CARTESIAN_POINT('Ctrl Pts',(-5.53391788006544,-14.7712644275784,
5.77232828169395));
#47268=CARTESIAN_POINT('Ctrl Pts',(-5.03788649172861,-13.9778126709648,
5.82466165747803));
#47269=CARTESIAN_POINT('Ctrl Pts',(-4.9839547824182,-13.1553705931073,5.87699503326212));
#47270=CARTESIAN_POINT('Ctrl Pts',(-4.9300230731078,-12.3329285152499,5.9293284090462));
#47271=CARTESIAN_POINT('Ctrl Pts',(-5.31819104282381,-11.4814961161485,
5.98166178483029));
#47272=CARTESIAN_POINT('Ctrl Pts',(-5.97442142669028,-10.9828167750565,
6.03399516061437));
#47273=CARTESIAN_POINT('Ctrl Pts',(-6.63065181055676,-10.4841374339645,
6.08632853639846));
#47274=CARTESIAN_POINT('Ctrl Pts',(-7.5549446085737,-10.338211150882,6.13866191218254));
#47275=CARTESIAN_POINT('Ctrl Pts',(-8.33288886120492,-10.6104648899579,
6.19099528796662));
#47276=CARTESIAN_POINT('Ctrl Pts',(-9.11083311383614,-10.8827186290339,
6.24332866375071));
#47277=CARTESIAN_POINT('Ctrl Pts',(-9.74242882108165,-11.5731523902683,
6.29566203953479));
#47278=CARTESIAN_POINT('Ctrl Pts',(-9.94449694127237,-12.3722067750024,
6.34799541531888));
#47279=CARTESIAN_POINT('Ctrl Pts',(-9.9952343802911,-12.5728419522874,6.36113584271526));
#47280=CARTESIAN_POINT('Ctrl Pts',(-10.0188915771041,-12.7803252875989,
6.37427627011165));
#47281=CARTESIAN_POINT('Ctrl Pts',(-10.0170829580245,-12.9882144302548,
6.38741669750803));
#47282=CARTESIAN_POINT('Origin',(-7.50000000000001,-12.9903810567666,7.5));
#47283=CARTESIAN_POINT('',(-10.0145082114167,-12.9918189296441,7.38741669750803));
#47284=CARTESIAN_POINT('',(-10.018916148665,-12.992363782792,7.11258330249199));
#47285=CARTESIAN_POINT('',(-10.0175,-12.9903810567666,7.5));
#47286=CARTESIAN_POINT('Ctrl Pts',(-10.018916148665,-12.992363782792,7.11258330249199));
#47287=CARTESIAN_POINT('Ctrl Pts',(-10.0130304015467,-12.3102957636159,
7.06938967489226));
#47288=CARTESIAN_POINT('Ctrl Pts',(-9.72554857159998,-11.6238530781169,
7.02619604729253));
#47289=CARTESIAN_POINT('Ctrl Pts',(-9.23088494583046,-11.1568755721922,
6.98300241969281));
#47290=CARTESIAN_POINT('Ctrl Pts',(-8.63155076501069,-10.5910858791674,
6.93066904390873));
#47291=CARTESIAN_POINT('Ctrl Pts',(-7.72807925079087,-10.3474651982644,
6.87833566812465));
#47292=CARTESIAN_POINT('Ctrl Pts',(-6.92554619007859,-10.5352419954014,
6.82600229234057));
#47293=CARTESIAN_POINT('Ctrl Pts',(-6.12301312936631,-10.7230187925383,
6.77366891655648));
#47294=CARTESIAN_POINT('Ctrl Pts',(-5.42141852216156,-11.342193067715,6.72133554077239));
#47295=CARTESIAN_POINT('Ctrl Pts',(-5.13532567649039,-12.1151551330277,
6.6690021649883));
#47296=CARTESIAN_POINT('Ctrl Pts',(-4.84923283081922,-12.8881171983403,
6.61666878920422));
#47297=CARTESIAN_POINT('Ctrl Pts',(-4.97864174668163,-13.8148670537889,
6.56433541342015));
#47298=CARTESIAN_POINT('Ctrl Pts',(-5.46553131494727,-14.4798918223762,
6.51200203763606));
#47299=CARTESIAN_POINT('Ctrl Pts',(-5.95242088321289,-15.1449165909636,
6.45966866185198));
#47300=CARTESIAN_POINT('Ctrl Pts',(-6.79679110388174,-15.5482162726898,
6.40733528606788));
#47301=CARTESIAN_POINT('Ctrl Pts',(-7.62006454012935,-15.5089697827308,
6.3550019102838));
#47302=CARTESIAN_POINT('Ctrl Pts',(-8.44333797637697,-15.4697232927718,
6.30266853449971));
#47303=CARTESIAN_POINT('Ctrl Pts',(-9.24551462820336,-14.9879306311276,
6.25033515871564));
#47304=CARTESIAN_POINT('Ctrl Pts',(-9.6669347422295,-14.2796053359332,6.19800178293155));
#47305=CARTESIAN_POINT('Ctrl Pts',(-9.89621522991991,-13.8942294041248,
6.16952895611836));
#47306=CARTESIAN_POINT('Ctrl Pts',(-10.012788678108,-13.4417979658618,6.14105612930517));
#47307=CARTESIAN_POINT('Ctrl Pts',(-10.0137189064297,-12.9898141627747,
6.11258330249198));
#47308=CARTESIAN_POINT('Ctrl Pts',(-10.0170829580245,-12.9882144302548,
6.38741669750803));
#47309=CARTESIAN_POINT('Ctrl Pts',(-10.0116885281401,-13.6082694857485,
6.42660964589573));
#47310=CARTESIAN_POINT('Ctrl Pts',(-9.77974909684708,-14.2319346209584,
6.46580259428343));
#47311=CARTESIAN_POINT('Ctrl Pts',(-9.36410112291705,-14.688271412029,6.50499554267113));
#47312=CARTESIAN_POINT('Ctrl Pts',(-8.80909665123509,-15.2976066560878,
6.55732891845521));
#47313=CARTESIAN_POINT('Ctrl Pts',(-7.92654717473526,-15.6086021359717,
6.6096622942393));
#47314=CARTESIAN_POINT('Ctrl Pts',(-7.11214796457486,-15.4818215077834,
6.66199567002339));
#47315=CARTESIAN_POINT('Ctrl Pts',(-6.29774875441446,-15.3550408795951,
6.71432904580747));
#47316=CARTESIAN_POINT('Ctrl Pts',(-5.55149981059349,-14.7904841433347,
6.76666242159156));
#47317=CARTESIAN_POINT('Ctrl Pts',(-5.20798543690379,-14.041273034435,6.81899579737564));
#47318=CARTESIAN_POINT('Ctrl Pts',(-4.8644710632141,-13.2920619255352,6.87132917315972));
#47319=CARTESIAN_POINT('Ctrl Pts',(-4.92369125965567,-12.3581964439962,
6.92366254894381));
#47320=CARTESIAN_POINT('Ctrl Pts',(-5.35909436185687,-11.6583796505146,
6.97599592472789));
#47321=CARTESIAN_POINT('Ctrl Pts',(-5.79449746405807,-10.958562857033,7.02832930051198));
#47322=CARTESIAN_POINT('Ctrl Pts',(-6.60608347201889,-10.4927947516089,
7.08066267629606));
#47323=CARTESIAN_POINT('Ctrl Pts',(-7.42997390874126,-10.469904702335,7.13299605208014));
#47324=CARTESIAN_POINT('Ctrl Pts',(-8.25386434546363,-10.4470146530611,
7.18532942786423));
#47325=CARTESIAN_POINT('Ctrl Pts',(-9.09005921094755,-10.8670026599375,
7.23766280364831));
#47326=CARTESIAN_POINT('Ctrl Pts',(-9.56364652484227,-11.5415650835207,
7.2899961794324));
#47327=CARTESIAN_POINT('Ctrl Pts',(-9.8575133022249,-11.9601393986381,7.32246968545761));
#47328=CARTESIAN_POINT('Ctrl Pts',(-10.0117632716449,-12.4767339212603,
7.35494319148282));
#47329=CARTESIAN_POINT('Ctrl Pts',(-10.0145082114167,-12.9918189296441,
7.38741669750803));
#47330=CARTESIAN_POINT('Origin',(-7.50000000000001,-12.9903810567666,7.5));
#47331=CARTESIAN_POINT('',(-10.0214372954169,-12.9905287409231,8.38741669750803));
#47332=CARTESIAN_POINT('',(-10.0184392382435,-12.988301844852,8.11258330249199));
#47333=CARTESIAN_POINT('',(-10.0175,-12.9903810567666,7.5));
#47334=CARTESIAN_POINT('Ctrl Pts',(-10.0184392382435,-12.988301844852,8.11258330249199));
#47335=CARTESIAN_POINT('Ctrl Pts',(-10.0198619759554,-12.8272606230119,
8.10238997204752));
#47336=CARTESIAN_POINT('Ctrl Pts',(-10.0057050234181,-12.6664683956915,
8.09219664160306));
#47337=CARTESIAN_POINT('Ctrl Pts',(-9.97504897913497,-12.5088858958898,
8.08200331115859));
#47338=CARTESIAN_POINT('Ctrl Pts',(-9.81765838984107,-11.699844707237,8.02966993537451));
#47339=CARTESIAN_POINT('Ctrl Pts',(-9.22537188297354,-10.9754080177822,
7.97733655959042));
#47340=CARTESIAN_POINT('Ctrl Pts',(-8.46374395491092,-10.660380492594,7.92500318380633));
#47341=CARTESIAN_POINT('Ctrl Pts',(-7.70211602684831,-10.3453529674058,
7.87266980802225));
#47342=CARTESIAN_POINT('Ctrl Pts',(-6.77114667759061,-10.4397346064841,
7.82033643223817));
#47343=CARTESIAN_POINT('Ctrl Pts',(-6.0882404805551,-10.9012089485628,7.76800305645409));
#47344=CARTESIAN_POINT('Ctrl Pts',(-5.4053342835196,-11.3626832906415,7.71566968067));
#47345=CARTESIAN_POINT('Ctrl Pts',(-4.97049123870628,-12.1912503357206,
7.66333630488591));
#47346=CARTESIAN_POINT('Ctrl Pts',(-4.97867531110115,-13.0154180759185,
7.61100292910183));
#47347=CARTESIAN_POINT('Ctrl Pts',(-4.98685938349602,-13.8395858161164,
7.55866955331774));
#47348=CARTESIAN_POINT('Ctrl Pts',(-5.43807057309907,-14.6593542514331,
7.50633617753366));
#47349=CARTESIAN_POINT('Ctrl Pts',(-6.130006178679,-15.1071762692505,7.45400280174958));
#47350=CARTESIAN_POINT('Ctrl Pts',(-6.82194178425893,-15.554998287068,7.40166942596549));
#47351=CARTESIAN_POINT('Ctrl Pts',(-7.75460180581574,-15.6308738873863,
7.3493360501814));
#47352=CARTESIAN_POINT('Ctrl Pts',(-8.509823648947,-15.3007838855131,7.29700267439732));
#47353=CARTESIAN_POINT('Ctrl Pts',(-9.26504549207826,-14.9706938836398,
7.24466929861323));
#47354=CARTESIAN_POINT('Ctrl Pts',(-9.84282915678396,-14.2346382795751,
7.19233592282916));
#47355=CARTESIAN_POINT('Ctrl Pts',(-9.98412256542695,-13.4226311249693,
7.14000254704507));
#47356=CARTESIAN_POINT('Ctrl Pts',(-10.0087987143617,-13.2808183562381,
7.13086279886071));
#47357=CARTESIAN_POINT('Ctrl Pts',(-10.0201615695645,-13.1366890058931,
7.12172305067635));
#47358=CARTESIAN_POINT('Ctrl Pts',(-10.018916148665,-12.992363782792,7.11258330249199));
#47359=CARTESIAN_POINT('Ctrl Pts',(-10.0145082114167,-12.9918189296441,
7.38741669750803));
#47360=CARTESIAN_POINT('Ctrl Pts',(-10.0161869382632,-13.306830224492,7.4072765672669));
#47361=CARTESIAN_POINT('Ctrl Pts',(-9.96119980531574,-13.6212769313365,
7.42713643702578));
#47362=CARTESIAN_POINT('Ctrl Pts',(-9.84682750368121,-13.9123926462011,
7.44699630678465));
#47363=CARTESIAN_POINT('Ctrl Pts',(-9.54544140631991,-14.6795209450086,
7.49932968256874));
#47364=CARTESIAN_POINT('Ctrl Pts',(-8.83168944929182,-15.2846407023335,
7.55166305835282));
#47365=CARTESIAN_POINT('Ctrl Pts',(-8.02558574588715,-15.4564435717975,
7.60399643413691));
#47366=CARTESIAN_POINT('Ctrl Pts',(-7.21948204248248,-15.6282464412614,
7.65632980992099));
#47367=CARTESIAN_POINT('Ctrl Pts',(-6.32102659270125,-15.3667324228643,
7.70866318570508));
#47368=CARTESIAN_POINT('Ctrl Pts',(-5.73304620733022,-14.789152581525,7.76099656148916));
#47369=CARTESIAN_POINT('Ctrl Pts',(-5.1450658219592,-14.2115727401857,7.81332993727324));
#47370=CARTESIAN_POINT('Ctrl Pts',(-4.86756050099838,-13.3179270759042,
7.86566331305732));
#47371=CARTESIAN_POINT('Ctrl Pts',(-5.02495108614128,-12.5088859085888,
7.91799668884141));
#47372=CARTESIAN_POINT('Ctrl Pts',(-5.18234167128417,-11.6998447412735,
7.9703300646255));
#47373=CARTESIAN_POINT('Ctrl Pts',(-5.77462816253079,-10.9754080709243,
8.02266344040959));
#47374=CARTESIAN_POINT('Ctrl Pts',(-6.53625607050644,-10.6603805540446,
8.07499681619367));
#47375=CARTESIAN_POINT('Ctrl Pts',(-7.29788397848209,-10.3453530371649,
8.12733019197775));
#47376=CARTESIAN_POINT('Ctrl Pts',(-8.22885330318678,-10.4397346737546,
8.17966356776183));
#47377=CARTESIAN_POINT('Ctrl Pts',(-8.91175948221152,-10.9012090036623,
8.23199694354592));
#47378=CARTESIAN_POINT('Ctrl Pts',(-9.5877914836703,-11.3580381032537,8.28380352819995));
#47379=CARTESIAN_POINT('Ctrl Pts',(-10.0207292434803,-12.1746067346983,
8.33561011285399));
#47380=CARTESIAN_POINT('Ctrl Pts',(-10.0214372954169,-12.9905287409231,
8.38741669750803));
#47381=CARTESIAN_POINT('Origin',(-7.50000000000001,-12.9903810567666,7.5));
#47382=CARTESIAN_POINT('',(-10.014824715197,-12.9887562509003,9.38741669750802));
#47383=CARTESIAN_POINT('',(-10.0138589040853,-12.9911961164478,9.11258330249198));
#47384=CARTESIAN_POINT('',(-10.0175,-12.9903810567666,7.5));
#47385=CARTESIAN_POINT('Ctrl Pts',(-10.0138589040853,-12.9911961164478,
9.11258330249198));
#47386=CARTESIAN_POINT('Ctrl Pts',(-10.0124667099841,-12.5225530777913,
9.08305689341869));
#47387=CARTESIAN_POINT('Ctrl Pts',(-9.88655945291767,-12.0532151702485,
9.05353048434541));
#47388=CARTESIAN_POINT('Ctrl Pts',(-9.64090569460772,-11.6583796153827,
9.02400407527212));
#47389=CARTESIAN_POINT('Ctrl Pts',(-9.20550258092411,-10.9585628034427,
8.97167069948803));
#47390=CARTESIAN_POINT('Ctrl Pts',(-8.39391655155678,-10.4927946857384,
8.91933732370393));
#47391=CARTESIAN_POINT('Ctrl Pts',(-7.57002609310491,-10.4699046358618,
8.86700394791985));
#47392=CARTESIAN_POINT('Ctrl Pts',(-6.74613563465304,-10.4470145859851,
8.81467057213576));
#47393=CARTESIAN_POINT('Ctrl Pts',(-5.90994074711664,-10.8670026039362,
8.7623371963517));
#47394=CARTESIAN_POINT('Ctrl Pts',(-5.43635342073195,-11.5415650453096,
8.71000382056761));
#47395=CARTESIAN_POINT('Ctrl Pts',(-4.96276609434725,-12.216127486683,8.65767044478353));
#47396=CARTESIAN_POINT('Ctrl Pts',(-4.85178632911427,-13.1452643514787,
8.60533706899943));
#47397=CARTESIAN_POINT('Ctrl Pts',(-5.15317243442415,-13.9123926705184,
8.55300369321534));
#47398=CARTESIAN_POINT('Ctrl Pts',(-5.45455853973402,-14.6795209895581,
8.50067031743125));
#47399=CARTESIAN_POINT('Ctrl Pts',(-6.16831051558674,-15.2846407628417,
8.44833694164718));
#47400=CARTESIAN_POINT('Ctrl Pts',(-6.97441424025143,-15.4564436368365,
8.3960035658631));
#47401=CARTESIAN_POINT('Ctrl Pts',(-7.78051796491612,-15.6282465108314,
8.34367019007902));
#47402=CARTESIAN_POINT('Ctrl Pts',(-8.67897343839277,-15.3667324855376,
8.29133681429492));
#47403=CARTESIAN_POINT('Ctrl Pts',(-9.26695383927095,-14.7891526289653,
8.23900343851084));
#47404=CARTESIAN_POINT('Ctrl Pts',(-9.74040926576667,-14.324071961446,8.19686339317122));
#47405=CARTESIAN_POINT('Ctrl Pts',(-10.0125575264699,-13.6540591679237,
8.15472334783161));
#47406=CARTESIAN_POINT('Ctrl Pts',(-10.0184392382435,-12.988301844852,8.11258330249199));
#47407=CARTESIAN_POINT('Ctrl Pts',(-10.0214372954169,-12.9905287409231,
8.38741669750803));
#47408=CARTESIAN_POINT('Ctrl Pts',(-10.0214444951867,-12.9988253788613,
8.38794348863808));
#47409=CARTESIAN_POINT('Ctrl Pts',(-10.0214070037996,-13.0071219499406,
8.38847027976813));
#47410=CARTESIAN_POINT('Ctrl Pts',(-10.0213246224021,-13.0154180752574,
8.38899707089817));
#47411=CARTESIAN_POINT('Ctrl Pts',(-10.0131405502232,-13.8395857937195,
8.44133044668226));
#47412=CARTESIAN_POINT('Ctrl Pts',(-9.56192937252059,-14.6593542074181,
8.49366382246634));
#47413=CARTESIAN_POINT('Ctrl Pts',(-8.86999378518945,-15.1071762134239,
8.54599719825042));
#47414=CARTESIAN_POINT('Ctrl Pts',(-8.17805819785831,-15.5549982194297,
8.59833057403451));
#47415=CARTESIAN_POINT('Ctrl Pts',(-7.24539820089864,-15.6308738177427,
8.6506639498186));
#47416=CARTESIAN_POINT('Ctrl Pts',(-6.49017637768564,-15.300783824577,8.70299732560268));
#47417=CARTESIAN_POINT('Ctrl Pts',(-5.73495455447264,-14.9706938314114,
8.75533070138677));
#47418=CARTESIAN_POINT('Ctrl Pts',(-5.15717090500631,-14.2346382467671,
8.80766407717085));
#47419=CARTESIAN_POINT('Ctrl Pts',(-5.01587750008917,-13.4226311135736,
8.85999745295493));
#47420=CARTESIAN_POINT('Ctrl Pts',(-4.87458409517204,-12.6106239803801,
8.91233082873901));
#47421=CARTESIAN_POINT('Ctrl Pts',(-5.16978093480409,-11.7226652986374,
8.96466420452309));
#47422=CARTESIAN_POINT('Ctrl Pts',(-5.76911509981821,-11.1568756205409,
9.01699758030718));
#47423=CARTESIAN_POINT('Ctrl Pts',(-6.36844926483233,-10.5910859424444,
9.06933095609127));
#47424=CARTESIAN_POINT('Ctrl Pts',(-7.27192075522852,-10.3474652679941,
9.12166433187536));
#47425=CARTESIAN_POINT('Ctrl Pts',(-8.07445379477299,-10.5352420601668,
9.17399770765945));
#47426=CARTESIAN_POINT('Ctrl Pts',(-8.87698683431745,-10.7230188523395,
9.22633108344353));
#47427=CARTESIAN_POINT('Ctrl Pts',(-9.5785814230102,-11.3421931111353,9.27866445922761));
#47428=CARTESIAN_POINT('Ctrl Pts',(-9.86467426114011,-12.1151551560838,
9.33099783501169));
#47429=CARTESIAN_POINT('Ctrl Pts',(-9.96748330192147,-12.3929233341375,
9.34980412251047));
#47430=CARTESIAN_POINT('Ctrl Pts',(-10.0166359465243,-12.6905511117478,
9.36861041000925));
#47431=CARTESIAN_POINT('Ctrl Pts',(-10.014824715197,-12.9887562509003,9.38741669750802));
#47432=CARTESIAN_POINT('Origin',(-7.50000000000001,-12.9903810567666,7.5));
#47433=CARTESIAN_POINT('',(-10.0166114900998,-12.9925168768863,10.387416697508));
#47434=CARTESIAN_POINT('',(-10.0209920718673,-12.9913179799917,10.112583302492));
#47435=CARTESIAN_POINT('',(-10.0175,-12.9903810567666,7.5));
#47436=CARTESIAN_POINT('Ctrl Pts',(-10.0209920718673,-12.9913179799917,
10.112583302492));
#47437=CARTESIAN_POINT('Ctrl Pts',(-10.0172626706847,-12.2214467116455,
10.0637238147899));
#47438=CARTESIAN_POINT('Ctrl Pts',(-9.63824845828795,-11.4483937541634,
10.0148643270877));
#47439=CARTESIAN_POINT('Ctrl Pts',(-9.02557861358329,-10.9828167220247,
9.96600483938563));
#47440=CARTESIAN_POINT('Ctrl Pts',(-8.36934821243818,-10.4841373677117,
9.91367146360155));
#47441=CARTESIAN_POINT('Ctrl Pts',(-7.44505538997194,-10.3382110809426,
9.86133808781746));
#47442=CARTESIAN_POINT('Ctrl Pts',(-6.66711111680735,-10.6104648272364,
9.80900471203337));
#47443=CARTESIAN_POINT('Ctrl Pts',(-5.88916684364275,-10.8827185735301,
9.75667133624929));
#47444=CARTESIAN_POINT('Ctrl Pts',(-5.2575711197798,-11.5731523528866,9.70433796046521));
#47445=CARTESIAN_POINT('Ctrl Pts',(-5.05550299426883,-12.3722067586746,
9.65200458468113));
#47446=CARTESIAN_POINT('Ctrl Pts',(-4.85343486875787,-13.1712611644625,
9.59967120889704));
#47447=CARTESIAN_POINT('Ctrl Pts',(-5.08089434159889,-14.0789361966818,
9.54733783311295));
#47448=CARTESIAN_POINT('Ctrl Pts',(-5.63589882791342,-14.6882714568219,
9.49500445732887));
#47449=CARTESIAN_POINT('Ctrl Pts',(-6.19090331422795,-15.297606716962,9.44267108154478));
#47450=CARTESIAN_POINT('Ctrl Pts',(-7.07345281401599,-15.6086022050228,
9.3903377057607));
#47451=CARTESIAN_POINT('Ctrl Pts',(-7.88785204565785,-15.4818215734849,
9.33800432997662));
#47452=CARTESIAN_POINT('Ctrl Pts',(-8.70225127729972,-15.3550409419471,
9.28567095419253));
#47453=CARTESIAN_POINT('Ctrl Pts',(-9.44850024079541,-14.7904841908106,
9.23333757840844));
#47454=CARTESIAN_POINT('Ctrl Pts',(-9.79201462354332,-14.0412730621545,
9.18100420262436));
#47455=CARTESIAN_POINT('Ctrl Pts',(-9.94171872679729,-13.7147656848908,
9.15819723591356));
#47456=CARTESIAN_POINT('Ctrl Pts',(-10.0149342710371,-13.3531881946364,
9.13539026920277));
#47457=CARTESIAN_POINT('Ctrl Pts',(-10.0138589040853,-12.9911961164478,
9.11258330249198));
#47458=CARTESIAN_POINT('Ctrl Pts',(-10.014824715197,-12.9887562509003,9.38741669750802));
#47459=CARTESIAN_POINT('Ctrl Pts',(-10.0115957252851,-13.5203843049831,
9.42094378579333));
#47460=CARTESIAN_POINT('Ctrl Pts',(-9.84639173717802,-14.053847347733,9.45447087407864));
#47461=CARTESIAN_POINT('Ctrl Pts',(-9.53446863140466,-14.4798917831418,
9.48799796236395));
#47462=CARTESIAN_POINT('Ctrl Pts',(-9.04757907597225,-15.1449165341501,
9.54033133814803));
#47463=CARTESIAN_POINT('Ctrl Pts',(-8.20320887754036,-15.5482162050654,
9.59266471393211));
#47464=CARTESIAN_POINT('Ctrl Pts',(-7.37993546302102,-15.5089697162145,
9.6449980897162));
#47465=CARTESIAN_POINT('Ctrl Pts',(-6.55666204850167,-15.4697232273637,
9.69733146550028));
#47466=CARTESIAN_POINT('Ctrl Pts',(-5.75448541789485,-14.9879305787468,
9.74966484128437));
#47467=CARTESIAN_POINT('Ctrl Pts',(-5.3330653149527,-14.2796053021006,9.80199821706846));
#47468=CARTESIAN_POINT('Ctrl Pts',(-4.91164521201054,-13.5712800254544,
9.85433159285254));
#47469=CARTESIAN_POINT('Ctrl Pts',(-4.87098163673303,-12.636422120779,9.90666496863662));
#47470=CARTESIAN_POINT('Ctrl Pts',(-5.22930629119846,-11.8941806184447,
9.95899834442071));
#47471=CARTESIAN_POINT('Ctrl Pts',(-5.58763094566388,-11.1519391161105,
10.0113317202048));
#47472=CARTESIAN_POINT('Ctrl Pts',(-6.34494382987224,-10.6023140161175,
10.0636650959889));
#47473=CARTESIAN_POINT('Ctrl Pts',(-7.1617000931268,-10.4917304028291,10.115998471773));
#47474=CARTESIAN_POINT('Ctrl Pts',(-7.97845635638136,-10.3811467895407,
10.168331847557));
#47475=CARTESIAN_POINT('Ctrl Pts',(-8.85465599868212,-10.7096046629569,
10.2206652233411));
#47476=CARTESIAN_POINT('Ctrl Pts',(-9.39745068084417,-11.3298422064682,
10.2729985991252));
#47477=CARTESIAN_POINT('Ctrl Pts',(-9.79302701821837,-11.781857128182,10.3111379652528));
#47478=CARTESIAN_POINT('Ctrl Pts',(-10.0115266235871,-12.3888409214585,
10.3492773313804));
#47479=CARTESIAN_POINT('Ctrl Pts',(-10.0166114900998,-12.9925168768863,
10.387416697508));
#47480=CARTESIAN_POINT('Origin',(-7.50000000000001,-12.9903810567666,7.5));
#47481=CARTESIAN_POINT('',(-10.0205077525331,-12.989132710429,11.387416697508));
#47482=CARTESIAN_POINT('',(-10.0159021674261,-12.9883695445715,11.112583302492));
#47483=CARTESIAN_POINT('',(-10.0175,-12.9903810567666,7.5));
#47484=CARTESIAN_POINT('',(-5.5865340033349,-11.3543938533917,12.));
#47485=CARTESIAN_POINT('Ctrl Pts',(-10.0205077525331,-12.989132710429,11.387416697508));
#47486=CARTESIAN_POINT('Ctrl Pts',(-10.0157036585105,-13.732988657673,11.4346110043198));
#47487=CARTESIAN_POINT('Ctrl Pts',(-9.66521749773701,-14.4805837586295,
11.4818053111315));
#47488=CARTESIAN_POINT('Ctrl Pts',(-9.08783263489828,-14.9488474815931,
11.5289996179432));
#47489=CARTESIAN_POINT('Ctrl Pts',(-8.44757534455355,-15.468101244079,11.5813329937273));
#47490=CARTESIAN_POINT('Ctrl Pts',(-7.52831414497493,-15.6438777379762,
11.6336663695114));
#47491=CARTESIAN_POINT('Ctrl Pts',(-6.74219676859447,-15.395694540416,11.6859997452955));
#47492=CARTESIAN_POINT('Ctrl Pts',(-5.956079392214,-15.1475113428559,11.7383331210796));
#47493=CARTESIAN_POINT('Ctrl Pts',(-5.3031058390317,-14.4753684538384,11.7906664968637));
#47494=CARTESIAN_POINT('Ctrl Pts',(-5.07623304195856,-13.6843856961865,
11.8429998726477));
#47495=CARTESIAN_POINT('Ctrl Pts',(-4.84936024488542,-12.8934029385347,
11.8953332484318));
#47496=CARTESIAN_POINT('Ctrl Pts',(-5.04858820392145,-11.9835803122485,
11.9476666242159));
#47497=CARTESIAN_POINT('Ctrl Pts',(-5.5865340033349,-11.3543938533917,12.));
#47498=CARTESIAN_POINT('',(-9.41699369782473,-11.3520708274328,12.));
#47499=CARTESIAN_POINT('Origin',(-7.50000000000001,-12.9903810567666,12.));
#47500=CARTESIAN_POINT('Ctrl Pts',(-9.41700750114216,-11.3520617378123,
12.));
#47501=CARTESIAN_POINT('Ctrl Pts',(-8.90328443334769,-10.7549233049312,
11.9500021225376));
#47502=CARTESIAN_POINT('Ctrl Pts',(-8.08591177198773,-10.4146528382252,
11.9000042450751));
#47503=CARTESIAN_POINT('Ctrl Pts',(-7.30082070365003,-10.4769905890799,
11.8500063676127));
#47504=CARTESIAN_POINT('Ctrl Pts',(-6.47905650106146,-10.5422402577977,
11.7976729918286));
#47505=CARTESIAN_POINT('Ctrl Pts',(-5.69266020241076,-11.048589867075,11.7453396160445));
#47506=CARTESIAN_POINT('Ctrl Pts',(-5.29374176559417,-11.769698237016,11.6930062402604));
#47507=CARTESIAN_POINT('Ctrl Pts',(-4.89482332877758,-12.4908066069571,
11.6406728644763));
#47508=CARTESIAN_POINT('Ctrl Pts',(-4.88338275379511,-13.4266737375619,
11.5883394886922));
#47509=CARTESIAN_POINT('Ctrl Pts',(-5.2647914049726,-14.1573521857831,11.5360061129082));
#47510=CARTESIAN_POINT('Ctrl Pts',(-5.64620005615009,-14.8880306340043,
11.4836727371241));
#47511=CARTESIAN_POINT('Ctrl Pts',(-6.42045793348755,-15.413520399842,11.43133936134));
#47512=CARTESIAN_POINT('Ctrl Pts',(-7.24029923554721,-15.4983927042523,
11.3790059855559));
#47513=CARTESIAN_POINT('Ctrl Pts',(-8.06014053760687,-15.5832650086627,
11.3266726097718));
#47514=CARTESIAN_POINT('Ctrl Pts',(-8.92556526438873,-15.2275198516459,
11.2743392339877));
#47515=CARTESIAN_POINT('Ctrl Pts',(-9.44861922536103,-14.5905668140585,
11.2220058582037));
#47516=CARTESIAN_POINT('Ctrl Pts',(-9.81316607095874,-14.146637051602,11.1855316729664));
#47517=CARTESIAN_POINT('Ctrl Pts',(-10.0114059764305,-13.566110281377,11.1490574877292));
#47518=CARTESIAN_POINT('Ctrl Pts',(-10.0159021674261,-12.9883695445715,
11.112583302492));
#47519=CARTESIAN_POINT('Origin',(-7.50000000000001,-12.9903810567666,14.2084234471775));
#47520=CARTESIAN_POINT('',(-10.5774091090731,-12.9889059662574,4.79157655282255));
#47521=CARTESIAN_POINT('',(-10.5686793840393,-12.990485538642,4.70842344717746));
#47522=CARTESIAN_POINT('',(-10.5735,-12.9903810567665,14.2084234471775));
#47523=CARTESIAN_POINT('',(-6.7062007174672,-15.9596040105123,4.));
#47524=CARTESIAN_POINT('Ctrl Pts',(-10.5686793840393,-12.990485538642,4.70842344717746));
#47525=CARTESIAN_POINT('Ctrl Pts',(-10.568341802375,-12.4708360960575,4.68161580125464));
#47526=CARTESIAN_POINT('Ctrl Pts',(-10.1982941291361,-10.9363980734526,
4.60247477954775));
#47527=CARTESIAN_POINT('Ctrl Pts',(-7.78634786537746,-9.38338007605921,
4.47100038205676));
#47528=CARTESIAN_POINT('Ctrl Pts',(-4.64704854581202,-10.7599538374027,
4.31400025470451));
#47529=CARTESIAN_POINT('Ctrl Pts',(-4.0706083548489,-14.143375884847,4.15700012735225));
#47530=CARTESIAN_POINT('Ctrl Pts',(-5.72985994157699,-15.6985866940351,
4.05233337578409));
#47531=CARTESIAN_POINT('Ctrl Pts',(-6.7062007174672,-15.9596040105123,4.));
#47532=CARTESIAN_POINT('',(-8.29574206058843,-15.9643807808206,4.));
#47533=CARTESIAN_POINT('Origin',(-7.50000000000001,-12.9903810567666,4.));
#47534=CARTESIAN_POINT('Ctrl Pts',(-10.5774091090731,-12.9889059662574,
4.79157655282255));
#47535=CARTESIAN_POINT('Ctrl Pts',(-10.5779245754331,-12.90178610915,4.78704908248048));
#47536=CARTESIAN_POINT('Ctrl Pts',(-10.5353931215559,-11.8081560623987,
4.73018823635433));
#47537=CARTESIAN_POINT('Ctrl Pts',(-9.23195310627391,-9.81262424147309,
4.62099401444409));
#47538=CARTESIAN_POINT('Ctrl Pts',(-5.80479621412607,-9.79242646017958,
4.46399388709183));
#47539=CARTESIAN_POINT('Ctrl Pts',(-3.89775220169895,-12.6409121056472,
4.30699375973959));
#47540=CARTESIAN_POINT('Ctrl Pts',(-5.20118245874298,-15.7537141165304,
4.15232913070897));
#47541=CARTESIAN_POINT('Ctrl Pts',(-7.3659421433414,-16.2099240527811,4.04999787746244));
#47542=CARTESIAN_POINT('Ctrl Pts',(-8.2957496623611,-15.9643994715412,4.));
#47543=CARTESIAN_POINT('Origin',(-7.50000000000001,-12.9903810567666,14.2084234471775));
#47544=CARTESIAN_POINT('',(-10.5688838367077,-12.9896889619566,5.79157655282255));
#47545=CARTESIAN_POINT('',(-10.576720384476,-12.9922616072697,5.70842344717746));
#47546=CARTESIAN_POINT('',(-10.5735,-12.9903810567665,14.2084234471775));
#47547=CARTESIAN_POINT('Ctrl Pts',(-10.576720384476,-12.9922616072697,5.70842344717746));
#47548=CARTESIAN_POINT('Ctrl Pts',(-10.5702730665099,-12.1038642909273,
5.66228272262582));
#47549=CARTESIAN_POINT('Ctrl Pts',(-9.70223177580237,-10.196831424253,5.56380862229009));
#47550=CARTESIAN_POINT('Ctrl Pts',(-6.48106313838945,-9.51757559757857,
5.41300114617028));
#47551=CARTESIAN_POINT('Ctrl Pts',(-4.04127232265978,-11.9244666993329,
5.25600101881803));
#47552=CARTESIAN_POINT('Ctrl Pts',(-4.70303574023142,-15.2872880321773,
5.09900089146577));
#47553=CARTESIAN_POINT('Ctrl Pts',(-7.87270740462966,-16.5902265862243,
4.94200076411352));
#47554=CARTESIAN_POINT('Ctrl Pts',(-10.2242698683325,-14.9942184798723,
4.81180828268408));
#47555=CARTESIAN_POINT('Ctrl Pts',(-10.5690008228703,-13.4852858404724,
4.73394917703873));
#47556=CARTESIAN_POINT('Ctrl Pts',(-10.5686793840393,-12.990485538642,4.70842344717746));
#47557=CARTESIAN_POINT('Ctrl Pts',(-10.5688838367077,-12.9896889619566,
5.79157655282255));
#47558=CARTESIAN_POINT('Ctrl Pts',(-10.5698355434391,-12.5272691260468,
5.76771600385165));
#47559=CARTESIAN_POINT('Ctrl Pts',(-10.2562654399242,-11.0518487505808,
5.69152207909667));
#47560=CARTESIAN_POINT('Ctrl Pts',(-7.98558650367391,-9.40388769480238,
5.56299477855761));
#47561=CARTESIAN_POINT('Ctrl Pts',(-4.77645084555843,-10.6068850809164,
5.40599465120535));
#47562=CARTESIAN_POINT('Ctrl Pts',(-4.00954797596254,-13.9472048059447,
5.24899452385311));
#47563=CARTESIAN_POINT('Ctrl Pts',(-6.37256666156175,-16.4294950347898,
5.09199439650084));
#47564=CARTESIAN_POINT('Ctrl Pts',(-9.64926888537511,-15.8453165147797,
4.93952173949067));
#47565=CARTESIAN_POINT('Ctrl Pts',(-10.5719662603729,-13.908811197287,4.83938245826456));
#47566=CARTESIAN_POINT('Ctrl Pts',(-10.5774091090731,-12.9889059662574,
4.79157655282255));
#47567=CARTESIAN_POINT('Origin',(-7.50000000000001,-12.9903810567666,14.2084234471775));
#47568=CARTESIAN_POINT('',(-10.5752289107932,-12.9928016758089,6.79157655282255));
#47569=CARTESIAN_POINT('',(-10.5729908526269,-12.9877359220758,6.70842344717746));
#47570=CARTESIAN_POINT('',(-10.5735,-12.9903810567665,14.2084234471775));
#47571=CARTESIAN_POINT('Ctrl Pts',(-10.5729908526269,-12.9877359220758,
6.70842344717746));
#47572=CARTESIAN_POINT('Ctrl Pts',(-10.5751989125043,-12.733933626166,6.69528301978108));
#47573=CARTESIAN_POINT('Ctrl Pts',(-10.4312908590873,-11.4718008748884,
6.62980921660061));
#47574=CARTESIAN_POINT('Ctrl Pts',(-8.69550592617927,-9.57431407095109,
6.51200203763606));
#47575=CARTESIAN_POINT('Ctrl Pts',(-5.31022618670948,-10.1087781397346,
6.3550019102838));
#47576=CARTESIAN_POINT('Ctrl Pts',(-3.88853690576949,-13.2272021460562,
6.19800178293155));
#47577=CARTESIAN_POINT('Ctrl Pts',(-5.70528265200966,-16.133268450666,6.0410016555793));
#47578=CARTESIAN_POINT('Ctrl Pts',(-9.13136587582039,-16.22107348372,5.88400152822704));
#47579=CARTESIAN_POINT('Ctrl Pts',(-10.5176208014685,-14.2374825953214,
5.77314212542643));
#47580=CARTESIAN_POINT('Ctrl Pts',(-10.5775856936348,-13.1114954248875,
5.7146160984099));
#47581=CARTESIAN_POINT('Ctrl Pts',(-10.576720384476,-12.9922616072697,5.70842344717746));
#47582=CARTESIAN_POINT('Ctrl Pts',(-10.5752289107932,-12.9928016758089,
6.79157655282255));
#47583=CARTESIAN_POINT('Ctrl Pts',(-10.5680432727522,-12.1600961914245,
6.74838292522283));
#47584=CARTESIAN_POINT('Ctrl Pts',(-9.79183080592196,-10.3066734191141,
6.65285592183901));
#47585=CARTESIAN_POINT('Ctrl Pts',(-6.67544463886838,-9.46634131342536,
6.50499554267114));
#47586=CARTESIAN_POINT('Ctrl Pts',(-4.10581084513197,-11.7341055256468,
6.34799541531887));
#47587=CARTESIAN_POINT('Ctrl Pts',(-4.57977903131249,-15.1283843904584,
6.19099528796663));
#47588=CARTESIAN_POINT('Ctrl Pts',(-7.67233737080682,-16.6054945057935,
6.03399516061437));
#47589=CARTESIAN_POINT('Ctrl Pts',(-10.1638447789511,-15.1090784945035,
5.90085558223301));
#47590=CARTESIAN_POINT('Ctrl Pts',(-10.56774816372,-13.5414952057652,5.82004937963574));
#47591=CARTESIAN_POINT('Ctrl Pts',(-10.5688838367077,-12.9896889619566,
5.79157655282255));
#47592=CARTESIAN_POINT('Origin',(-7.50000000000001,-12.9903810567666,14.2084234471775));
#47593=CARTESIAN_POINT('',(-10.574646672787,-12.9878426425384,7.79157655282256));
#47594=CARTESIAN_POINT('',(-10.5698474628756,-12.992136489652,7.70842344717746));
#47595=CARTESIAN_POINT('',(-10.5735,-12.9903810567665,14.2084234471775));
#47596=CARTESIAN_POINT('Ctrl Pts',(-10.5698474628756,-12.9921364896521,
7.70842344717746));
#47597=CARTESIAN_POINT('Ctrl Pts',(-10.5664962921154,-12.3632928855735,
7.67594994115225));
#47598=CARTESIAN_POINT('Ctrl Pts',(-10.0746937830591,-10.7162100151804,
7.59114305934296));
#47599=CARTESIAN_POINT('Ctrl Pts',(-7.39948645351245,-9.37255790644949,
7.45400280174957));
#47600=CARTESIAN_POINT('Ctrl Pts',(-4.42700232783115,-11.078462500715,7.29700267439732));
#47601=CARTESIAN_POINT('Ctrl Pts',(-4.21010468283033,-14.4988027877182,
7.14000254704507));
#47602=CARTESIAN_POINT('Ctrl Pts',(-6.94328775591919,-16.5665268737914,
6.98300241969282));
#47603=CARTESIAN_POINT('Ctrl Pts',(-9.90513870920436,-15.5228207892163,
6.83914271973694));
#47604=CARTESIAN_POINT('Ctrl Pts',(-10.566405041207,-13.7447326303419,6.74761639556516));
#47605=CARTESIAN_POINT('Ctrl Pts',(-10.5729908526269,-12.9877359220758,
6.70842344717746));
#47606=CARTESIAN_POINT('Ctrl Pts',(-10.574646672787,-12.9878426425384,7.79157655282256));
#47607=CARTESIAN_POINT('Ctrl Pts',(-10.5763836278447,-12.7912348191717,
7.78138322237809));
#47608=CARTESIAN_POINT('Ctrl Pts',(-10.4703648087191,-11.5870913412493,
7.71885651614955));
#47609=CARTESIAN_POINT('Ctrl Pts',(-8.88333183851511,-9.64596167231467,
7.60399643413689));
#47610=CARTESIAN_POINT('Ctrl Pts',(-5.47359881574229,-9.99164028328652,
7.44699630678467));
#47611=CARTESIAN_POINT('Ctrl Pts',(-3.88095917534459,-13.0263185113509,
7.28999617943238));
#47612=CARTESIAN_POINT('Ctrl Pts',(-5.53354816193247,-16.0287712850697,
7.13299605208016));
#47613=CARTESIAN_POINT('Ctrl Pts',(-8.94947337693327,-16.3066703804957,
6.97599592472788));
#47614=CARTESIAN_POINT('Ctrl Pts',(-10.4834449578808,-14.3524988668243,
6.86218942497536));
#47615=CARTESIAN_POINT('Ctrl Pts',(-10.5767493879072,-13.1690017048858,
6.80071630100692));
#47616=CARTESIAN_POINT('Ctrl Pts',(-10.5752289107932,-12.9928016758089,
6.79157655282255));
#47617=CARTESIAN_POINT('Origin',(-7.50000000000001,-12.9903810567666,14.2084234471775));
#47618=CARTESIAN_POINT('',(-10.5690547534087,-12.9913761256565,8.79157655282255));
#47619=CARTESIAN_POINT('',(-10.5783068629449,-12.9905613575631,8.70842344717746));
#47620=CARTESIAN_POINT('',(-10.5735,-12.9903810567665,14.2084234471775));
#47621=CARTESIAN_POINT('Ctrl Pts',(-10.5783068629449,-12.9905613575631,
8.70842344717747));
#47622=CARTESIAN_POINT('Ctrl Pts',(-10.5774424348904,-11.99443969475,8.65661686252343));
#47623=CARTESIAN_POINT('Ctrl Pts',(-9.51496026706992,-9.99048048802178,
8.55247690208529));
#47624=CARTESIAN_POINT('Ctrl Pts',(-6.11666819796815,-9.64596176051859,
8.3960035658631));
#47625=CARTESIAN_POINT('Ctrl Pts',(-3.94738216319582,-12.2992560282264,
8.23900343851084));
#47626=CARTESIAN_POINT('Ctrl Pts',(-4.96376262473273,-15.5722887382593,
8.0820033111586));
#47627=CARTESIAN_POINT('Ctrl Pts',(-8.25441147268027,-16.5301000616477,
7.92500318380633));
#47628=CARTESIAN_POINT('Ctrl Pts',(-10.3278659516785,-14.7722228904523,
7.80047656247929));
#47629=CARTESIAN_POINT('Ctrl Pts',(-10.5718969432977,-13.3767192958943,
7.72828331693634));
#47630=CARTESIAN_POINT('Ctrl Pts',(-10.5698474628756,-12.9921364896521,
7.70842344717746));
#47631=CARTESIAN_POINT('Ctrl Pts',(-10.5690547534086,-12.9913761256565,
8.79157655282255));
#47632=CARTESIAN_POINT('Ctrl Pts',(-10.5673550876409,-12.4192313871019,
8.76205014374926));
#47633=CARTESIAN_POINT('Ctrl Pts',(-10.1411933372985,-10.8306504836598,
8.6801903588919));
#47634=CARTESIAN_POINT('Ctrl Pts',(-7.60051354913579,-9.37255781103892,
8.54599719825042));
#47635=CARTESIAN_POINT('Ctrl Pts',(-4.53789787464541,-10.9107899935683,
8.38899707089818));
#47636=CARTESIAN_POINT('Ctrl Pts',(-4.13142759646044,-14.3138114282651,
8.23199694354591));
#47637=CARTESIAN_POINT('Ctrl Pts',(-6.74558850742372,-16.5301001550025,
8.07499681619368));
#47638=CARTESIAN_POINT('Ctrl Pts',(-9.82259002330375,-15.634475301008,7.92819001928586));
#47639=CARTESIAN_POINT('Ctrl Pts',(-10.5674659613129,-13.8006351479846,
7.83371659816217));
#47640=CARTESIAN_POINT('Ctrl Pts',(-10.574646672787,-12.9878426425384,7.79157655282256));
#47641=CARTESIAN_POINT('Origin',(-7.50000000000001,-12.9903810567666,14.2084234471775));
#47642=CARTESIAN_POINT('',(-10.5777633099838,-12.991524903254,9.79157655282255));
#47643=CARTESIAN_POINT('',(-10.5702338677887,-12.98839740599,9.70842344717746));
#47644=CARTESIAN_POINT('',(-10.5735,-12.9903810567665,14.2084234471775));
#47645=CARTESIAN_POINT('Ctrl Pts',(-10.5702338677887,-12.98839740599,9.70842344717746));
#47646=CARTESIAN_POINT('Ctrl Pts',(-10.5724451168391,-12.6243324625202,
9.68961715967868));
#47647=CARTESIAN_POINT('Ctrl Pts',(-10.3454485117827,-11.2498286970771,
9.61847749639582));
#47648=CARTESIAN_POINT('Ctrl Pts',(-8.32455533939524,-9.46634140643289,
9.49500445732887));
#47649=CARTESIAN_POINT('Ctrl Pts',(-5.01553493137219,-10.3586172470561,
9.33800432997662));
#47650=CARTESIAN_POINT('Ctrl Pts',(-3.93435818466818,-13.6108210305748,
9.18100420262436));
#47651=CARTESIAN_POINT('Ctrl Pts',(-6.05052666129351,-16.3066702930228,
9.02400407527212));
#47652=CARTESIAN_POINT('Ctrl Pts',(-9.46645178620579,-16.0287712049414,
8.86700394791984));
#47653=CARTESIAN_POINT('Ctrl Pts',(-10.5737227704402,-14.0170617812033,
8.76181040522164));
#47654=CARTESIAN_POINT('Ctrl Pts',(-10.5783156528128,-13.0006903413578,
8.70895023830751));
#47655=CARTESIAN_POINT('Ctrl Pts',(-10.5783068629449,-12.9905613575631,
8.70842344717747));
#47656=CARTESIAN_POINT('Ctrl Pts',(-10.5777633099838,-12.991524903254,9.79157655282255));
#47657=CARTESIAN_POINT('Ctrl Pts',(-10.5732102555509,-12.0516244689892,
9.74271706512043));
#47658=CARTESIAN_POINT('Ctrl Pts',(-9.61486894310576,-10.0969521595311,
9.64152420163424));
#47659=CARTESIAN_POINT('Ctrl Pts',(-6.30449404219616,-9.57431398106461,
9.48799796236394));
#47660=CARTESIAN_POINT('Ctrl Pts',(-3.99123550321764,-12.1030705501041,
9.33099783501171));
#47661=CARTESIAN_POINT('Ctrl Pts',(-4.82431993989319,-15.4274866909495,
9.17399770765942));
#47662=CARTESIAN_POINT('Ctrl Pts',(-8.05671225877921,-16.5665269680756,
9.0169975803072));
#47663=CARTESIAN_POINT('Ctrl Pts',(-10.2758761800147,-14.8876717402662,
8.88952386202821));
#47664=CARTESIAN_POINT('Ctrl Pts',(-10.5703676194767,-13.4333156101897,
8.81438351953334));
#47665=CARTESIAN_POINT('Ctrl Pts',(-10.5690547534086,-12.9913761256565,
8.79157655282255));
#47666=CARTESIAN_POINT('Origin',(-7.50000000000001,-12.9903810567666,14.2084234471775));
#47667=CARTESIAN_POINT('',(-10.5715492796759,-12.9879252940133,10.7915765528226));
#47668=CARTESIAN_POINT('',(-10.5724152591149,-12.9929885813497,10.7084234471775));
#47669=CARTESIAN_POINT('',(-10.5735,-12.9903810567665,14.2084234471775));
#47670=CARTESIAN_POINT('Ctrl Pts',(-10.5724152591149,-12.9929885813497,
10.7084234471775));
#47671=CARTESIAN_POINT('Ctrl Pts',(-10.5662073793823,-12.2559883632733,
10.6702840810499));
#47672=CARTESIAN_POINT('Ctrl Pts',(-9.93341873530542,-10.4981249983676,
10.5798113391382));
#47673=CARTESIAN_POINT('Ctrl Pts',(-7.01441350972263,-9.40388779191504,
10.4370052214424));
#47674=CARTESIAN_POINT('Ctrl Pts',(-4.2407080682755,-11.4169238334189,10.2800050940901));
#47675=CARTESIAN_POINT('Ctrl Pts',(-4.38964093653616,-14.8408989317544,
10.1230049667379));
#47676=CARTESIAN_POINT('Ctrl Pts',(-7.32766263366035,-16.6054944100355,
9.96600483938563));
#47677=CARTESIAN_POINT('Ctrl Pts',(-10.049778264125,-15.305320221038,9.82781099953216));
#47678=CARTESIAN_POINT('Ctrl Pts',(-10.5662917424682,-13.6374376539438,
9.74195053546276));
#47679=CARTESIAN_POINT('Ctrl Pts',(-10.5702338677887,-12.98839740599,9.70842344717746));
#47680=CARTESIAN_POINT('Ctrl Pts',(-10.5715492796759,-12.9879252940133,
10.7915765528226));
#47681=CARTESIAN_POINT('Ctrl Pts',(-10.5739360130587,-12.6812405681054,
10.7757173622757));
#47682=CARTESIAN_POINT('Ctrl Pts',(-10.3919168575192,-11.3652990254922,
10.7075247959448));
#47683=CARTESIAN_POINT('Ctrl Pts',(-8.51893689306524,-9.51757549146244,
10.5869988538297));
#47684=CARTESIAN_POINT('Ctrl Pts',(-5.16549637569413,-10.2247238388162,
10.4299987264775));
#47685=CARTESIAN_POINT('Ctrl Pts',(-3.90540678666615,-13.4118934459175,
10.2729985991252));
#47686=CARTESIAN_POINT('Ctrl Pts',(-5.86863408021139,-16.2210735713392,
10.115998471773));
#47687=CARTESIAN_POINT('Ctrl Pts',(-9.29471739586239,-16.133268532241,9.9589983444207));
#47688=CARTESIAN_POINT('Ctrl Pts',(-10.5460797704268,-14.1315894099677,
9.85085770477056));
#47689=CARTESIAN_POINT('Ctrl Pts',(-10.5780870301511,-13.0583514106611,
9.79505044090451));
#47690=CARTESIAN_POINT('Ctrl Pts',(-10.5777633099838,-12.991524903254,9.79157655282255));
#47691=CARTESIAN_POINT('Origin',(-7.50000000000001,-12.9903810567666,14.2084234471775));
#47692=CARTESIAN_POINT('',(-10.5702205181091,-12.9936861301783,11.7915765528225));
#47693=CARTESIAN_POINT('',(-10.5771720267767,-12.9888570081198,11.7084234471775));
#47694=CARTESIAN_POINT('',(-10.5735,-12.9903810567665,14.2084234471775));
#47695=CARTESIAN_POINT('',(-8.29379928253297,-15.9596040105122,12.));
#47696=CARTESIAN_POINT('Ctrl Pts',(-8.29379928253297,-15.9596040105122,
12.));
#47697=CARTESIAN_POINT('Ctrl Pts',(-9.27014005842316,-15.698586694035,11.9476666242159));
#47698=CARTESIAN_POINT('Ctrl Pts',(-10.3714986866323,-14.6662860075735,
11.8781921418234));
#47699=CARTESIAN_POINT('Ctrl Pts',(-10.5724951032558,-13.3253966136884,
11.8087176594309));
#47700=CARTESIAN_POINT('Ctrl Pts',(-10.5702205181091,-12.9936861301783,
11.7915765528225));
#47701=CARTESIAN_POINT('',(-6.70425809489808,-15.964380864449,12.));
#47702=CARTESIAN_POINT('Origin',(-7.50000000000001,-12.9903810567666,12.));
#47703=CARTESIAN_POINT('Ctrl Pts',(-6.70425049788239,-15.9643995452956,
12.));
#47704=CARTESIAN_POINT('Ctrl Pts',(-7.63405808481853,-16.2099241868245,
11.9500021225376));
#47705=CARTESIAN_POINT('Ctrl Pts',(-9.69010316575102,-15.7766245762052,
11.8528099382634));
#47706=CARTESIAN_POINT('Ctrl Pts',(-10.571306929268,-13.8969965329875,11.7556177539892));
#47707=CARTESIAN_POINT('Ctrl Pts',(-10.5771720267767,-12.9888570081198,
11.7084234471775));
#47708=CARTESIAN_POINT('Origin',(-7.5,12.9903810567666,7.5));
#47709=CARTESIAN_POINT('',(-10.0135512354019,12.9902955808623,4.38741669750803));
#47710=CARTESIAN_POINT('',(-10.0159871075715,12.98719611739,4.11258330249198));
#47711=CARTESIAN_POINT('',(-10.0175,12.9903810567666,7.5));
#47712=CARTESIAN_POINT('',(-9.41346599666504,14.6263682601415,4.));
#47713=CARTESIAN_POINT('Ctrl Pts',(-10.0159871075715,12.98719611739,4.11258330249198));
#47714=CARTESIAN_POINT('Ctrl Pts',(-10.0108029441705,13.5796929638899,4.07505553499465));
#47715=CARTESIAN_POINT('Ctrl Pts',(-9.79922182808404,14.175184617071,4.03752776749733));
#47716=CARTESIAN_POINT('Ctrl Pts',(-9.41346599666504,14.6263682601416,4.));
#47717=CARTESIAN_POINT('',(-10.0175,12.9903810567666,4.));
#47718=CARTESIAN_POINT('Origin',(-7.5,12.9903810567666,4.));
#47719=CARTESIAN_POINT('',(-10.0175,12.9903810567666,3.));
#47720=CARTESIAN_POINT('',(-10.0175,12.9903810567666,7.5));
#47721=CARTESIAN_POINT('Origin',(-7.5,12.9903810567666,3.));
#47722=CARTESIAN_POINT('',(-5.58300657818904,14.6286918237334,4.));
#47723=CARTESIAN_POINT('Origin',(-7.5,12.9903810567666,4.));
#47724=CARTESIAN_POINT('Ctrl Pts',(-5.58299280741585,14.6287008947316,4.));
#47725=CARTESIAN_POINT('Ctrl Pts',(-6.09671594976083,15.225839628633,4.04999787746244));
#47726=CARTESIAN_POINT('Ctrl Pts',(-6.91408837638834,15.566108849254,4.09999575492489));
#47727=CARTESIAN_POINT('Ctrl Pts',(-7.69917928811933,15.5037708430362,4.14999363238733));
#47728=CARTESIAN_POINT('Ctrl Pts',(-8.52094332678579,15.4385209070269,4.20232700817142));
#47729=CARTESIAN_POINT('Ctrl Pts',(-9.30733954710939,14.9321721158988,4.2546603839555));
#47730=CARTESIAN_POINT('Ctrl Pts',(-9.7062579619942,14.2110639837978,4.30699375973958));
#47731=CARTESIAN_POINT('Ctrl Pts',(-9.91060296091885,13.8416780768541,4.3338014056624));
#47732=CARTESIAN_POINT('Ctrl Pts',(-10.0132747138948,13.4159398344011,4.36060905158521));
#47733=CARTESIAN_POINT('Ctrl Pts',(-10.0135512354019,12.9902955808623,4.38741669750803));
#47734=CARTESIAN_POINT('Origin',(-7.5,12.9903810567666,7.5));
#47735=CARTESIAN_POINT('',(-10.0201376030965,12.9888406983805,5.38741669750803));
#47736=CARTESIAN_POINT('',(-10.0207017684327,12.9915893349038,5.11258330249198));
#47737=CARTESIAN_POINT('',(-10.0175,12.9903810567666,7.5));
#47738=CARTESIAN_POINT('Ctrl Pts',(-10.0207017684327,12.9915893349038,5.11258330249198));
#47739=CARTESIAN_POINT('Ctrl Pts',(-10.021123985829,13.062949094674,5.10805583214991));
#47740=CARTESIAN_POINT('Ctrl Pts',(-10.0183500982852,13.1342752724561,5.10352836180784));
#47741=CARTESIAN_POINT('Ctrl Pts',(-10.0122723502588,13.2053184595532,5.09900089146578));
#47742=CARTESIAN_POINT('Ctrl Pts',(-9.94201919621031,14.0265120900682,5.04666751568169));
#47743=CARTESIAN_POINT('Ctrl Pts',(-9.43032981516091,14.8098946989374,4.99433413989761));
#47744=CARTESIAN_POINT('Ctrl Pts',(-8.7066218792309,15.204343412931,4.94200076411352));
#47745=CARTESIAN_POINT('Ctrl Pts',(-7.98291394330089,15.5987921269246,4.88966738832944));
#47746=CARTESIAN_POINT('Ctrl Pts',(-7.04718745249026,15.6043069460425,4.83733401254535));
#47747=CARTESIAN_POINT('Ctrl Pts',(-6.31898125676283,15.2181990815764,4.78500063676127));
#47748=CARTESIAN_POINT('Ctrl Pts',(-5.59077506103539,14.8320912171102,4.73266726097718));
#47749=CARTESIAN_POINT('Ctrl Pts',(-5.07008916039116,14.0543606690598,4.6803338851931));
#47750=CARTESIAN_POINT('Ctrl Pts',(-4.99037298951262,13.2341300396427,4.62800050940902));
#47751=CARTESIAN_POINT('Ctrl Pts',(-4.91065681863409,12.4138994102257,4.57566713362493));
#47752=CARTESIAN_POINT('Ctrl Pts',(-5.27191037752124,11.5511686994419,4.52333375784085));
#47753=CARTESIAN_POINT('Ctrl Pts',(-5.91216754016691,11.0319148801645,4.47100038205676));
#47754=CARTESIAN_POINT('Ctrl Pts',(-6.55242470281257,10.5126610608871,4.41866700627268));
#47755=CARTESIAN_POINT('Ctrl Pts',(-7.47168546921673,10.336884133116,4.36633363048859));
#47756=CARTESIAN_POINT('Ctrl Pts',(-8.25780300491658,10.5850674765643,4.31400025470451));
#47757=CARTESIAN_POINT('Ctrl Pts',(-9.04392054061644,10.8332508200125,4.26166687892042));
#47758=CARTESIAN_POINT('Ctrl Pts',(-9.696894845612,11.50539443468,4.20933350313634));
#47759=CARTESIAN_POINT('Ctrl Pts',(-9.92376765947752,12.2963771799981,4.15700012735225));
#47760=CARTESIAN_POINT('Ctrl Pts',(-9.98795212995513,12.5201536995385,4.1421945190655));
#47761=CARTESIAN_POINT('Ctrl Pts',(-10.0180323849149,12.7534418387471,4.12738891077874));
#47762=CARTESIAN_POINT('Ctrl Pts',(-10.0159871075715,12.98719611739,4.11258330249198));
#47763=CARTESIAN_POINT('Ctrl Pts',(-10.0135512354019,12.9902955808623,4.38741669750803));
#47764=CARTESIAN_POINT('Ctrl Pts',(-10.0138145339143,12.5850052295903,4.4129424273693));
#47765=CARTESIAN_POINT('Ctrl Pts',(-9.92124134238478,12.1798000932329,4.43846815723057));
#47766=CARTESIAN_POINT('Ctrl Pts',(-9.73520837540778,11.8234099166911,4.46399388709184));
#47767=CARTESIAN_POINT('Ctrl Pts',(-9.35379976449056,11.0927314547595,4.51632726287592));
#47768=CARTESIAN_POINT('Ctrl Pts',(-8.57954193321014,10.5672420039701,4.56866063866001));
#47769=CARTESIAN_POINT('Ctrl Pts',(-7.75970071708304,10.482369764132,4.62099401444409));
#47770=CARTESIAN_POINT('Ctrl Pts',(-6.93985950095593,10.3974975242939,4.67332739022817));
#47771=CARTESIAN_POINT('Ctrl Pts',(-6.07443489998217,10.7532424954071,4.72566076601226));
#47772=CARTESIAN_POINT('Ctrl Pts',(-5.55138100127894,11.3901954309976,4.77799414179634));
#47773=CARTESIAN_POINT('Ctrl Pts',(-5.02832710257572,12.0271483665881,4.83032751758043));
#47774=CARTESIAN_POINT('Ctrl Pts',(-4.84764390614303,12.945309266656,4.88266089336452));
#47775=CARTESIAN_POINT('Ctrl Pts',(-5.09037388542358,13.7329699193423,4.9349942691486));
#47776=CARTESIAN_POINT('Ctrl Pts',(-5.33310386470412,14.5206305720287,4.98732764493268));
#47777=CARTESIAN_POINT('Ctrl Pts',(-5.9992470196979,15.1777909773334,5.03966102071676));
#47778=CARTESIAN_POINT('Ctrl Pts',(-6.79011836385736,15.4098338158843,5.09199439650085));
#47779=CARTESIAN_POINT('Ctrl Pts',(-7.58098970801682,15.6418766544352,5.14432777228493));
#47780=CARTESIAN_POINT('Ctrl Pts',(-8.49658924134195,15.4488019262325,5.19666114806902));
#47781=CARTESIAN_POINT('Ctrl Pts',(-9.12641195891838,14.9171634974037,5.24899452385311));
#47782=CARTESIAN_POINT('Ctrl Pts',(-9.68170723832013,14.4484342794212,5.29513524840475));
#47783=CARTESIAN_POINT('Ctrl Pts',(-10.0148566122412,13.7165257701398,5.34127597295639));
#47784=CARTESIAN_POINT('Ctrl Pts',(-10.0201376030965,12.9888406983805,5.38741669750803));
#47785=CARTESIAN_POINT('Origin',(-7.5,12.9903810567666,7.5));
#47786=CARTESIAN_POINT('',(-10.0170827477036,12.9925476830062,6.38741669750803));
#47787=CARTESIAN_POINT('',(-10.0137187170915,12.9909479514162,6.11258330249198));
#47788=CARTESIAN_POINT('',(-10.0175,12.9903810567666,7.5));
#47789=CARTESIAN_POINT('Ctrl Pts',(-10.0137187170915,12.9909479514162,6.11258330249198));
#47790=CARTESIAN_POINT('Ctrl Pts',(-10.0144982588899,13.3697154315319,6.08872275352109));
#47791=CARTESIAN_POINT('Ctrl Pts',(-9.93406587049998,13.7481685539756,6.06486220455019));
#47792=CARTESIAN_POINT('Ctrl Pts',(-9.77069359762705,14.0865814419388,6.0410016555793));
#47793=CARTESIAN_POINT('Ctrl Pts',(-9.41236896061271,14.8288229074456,5.98866827979521));
#47794=CARTESIAN_POINT('Ctrl Pts',(-8.65505611306826,15.3784479785104,5.93633490401113));
#47795=CARTESIAN_POINT('Ctrl Pts',(-7.83829989006264,15.4890315871854,5.88400152822704));
#47796=CARTESIAN_POINT('Ctrl Pts',(-7.02154366705702,15.5996151958603,5.83166815244296));
#47797=CARTESIAN_POINT('Ctrl Pts',(-6.14534406859022,15.2711573421455,5.77933477665887));
#47798=CARTESIAN_POINT('Ctrl Pts',(-5.60254941260429,14.6509198275943,5.72700140087479));
#47799=CARTESIAN_POINT('Ctrl Pts',(-5.05975475661836,14.0306823130431,5.6746680250907));
#47800=CARTESIAN_POINT('Ctrl Pts',(-4.8503650431133,13.1186651376555,5.62233464930662));
#47801=CARTESIAN_POINT('Ctrl Pts',(-5.06826110556232,12.3237831148942,5.57000127352254));
#47802=CARTESIAN_POINT('Ctrl Pts',(-5.28615716801134,11.5289010921329,5.51766789773845));
#47803=CARTESIAN_POINT('Ctrl Pts',(-5.93133900641445,10.8511542219977,5.46533452195436));
#47804=CARTESIAN_POINT('Ctrl Pts',(-6.71453634454677,10.5943988157391,5.41300114617028));
#47805=CARTESIAN_POINT('Ctrl Pts',(-7.49773368267909,10.3376434094805,5.3606677703862));
#47806=CARTESIAN_POINT('Ctrl Pts',(-8.41894652054063,10.5018794670985,5.30833439460211));
#47807=CARTESIAN_POINT('Ctrl Pts',(-9.06514447594766,11.0134998219879,5.25600101881803));
#47808=CARTESIAN_POINT('Ctrl Pts',(-9.65543848794614,11.4808588245671,5.20819511337601));
#47809=CARTESIAN_POINT('Ctrl Pts',(-10.0162435426697,12.2380961764306,5.160389207934));
#47810=CARTESIAN_POINT('Ctrl Pts',(-10.0207017684327,12.9915893349038,5.11258330249198));
#47811=CARTESIAN_POINT('Ctrl Pts',(-10.0201376030965,12.9888406983805,5.38741669750803));
#47812=CARTESIAN_POINT('Ctrl Pts',(-10.02084637685,12.8911764354056,5.39360934874047));
#47813=CARTESIAN_POINT('Ctrl Pts',(-10.0156492795336,12.793588248926,5.39980199997291));
#47814=CARTESIAN_POINT('Ctrl Pts',(-10.0042907210835,12.6967226001492,5.40599465120536));
#47815=CARTESIAN_POINT('Ctrl Pts',(-9.90830086384453,11.8781222611782,5.45832802698944));
#47816=CARTESIAN_POINT('Ctrl Pts',(-9.37227524753879,11.1111237126909,5.51066140277353));
#47817=CARTESIAN_POINT('Ctrl Pts',(-8.63654573295752,10.739611267924,5.56299477855761));
#47818=CARTESIAN_POINT('Ctrl Pts',(-7.90081621837627,10.368098823157,5.6153281543417));
#47819=CARTESIAN_POINT('Ctrl Pts',(-6.96538280551948,10.3920724821103,5.66766153012578));
#47820=CARTESIAN_POINT('Ctrl Pts',(-6.24965042528476,10.8007851576184,5.71999490590986));
#47821=CARTESIAN_POINT('Ctrl Pts',(-5.53391804505003,11.2094978331266,5.77232828169395));
#47822=CARTESIAN_POINT('Ctrl Pts',(-5.03788669743737,12.0029495251895,5.82466165747803));
#47823=CARTESIAN_POINT('Ctrl Pts',(-4.98395499247446,12.8253915347154,5.87699503326212));
#47824=CARTESIAN_POINT('Ctrl Pts',(-4.93002328751154,13.6478335442413,5.9293284090462));
#47825=CARTESIAN_POINT('Ctrl Pts',(-5.31819122519835,14.4992658712303,5.98166178483029));
#47826=CARTESIAN_POINT('Ctrl Pts',(-5.97442155431181,14.997945170426,6.03399516061437));
#47827=CARTESIAN_POINT('Ctrl Pts',(-6.63065188342527,15.4966244696218,6.08632853639846));
#47828=CARTESIAN_POINT('Ctrl Pts',(-7.55494460396538,15.6425507410243,6.13866191218253));
#47829=CARTESIAN_POINT('Ctrl Pts',(-8.33288879152928,15.3702970248207,6.19099528796662));
#47830=CARTESIAN_POINT('Ctrl Pts',(-9.11083297909318,15.0980433086171,6.2433286637507));
#47831=CARTESIAN_POINT('Ctrl Pts',(-9.74242863368087,14.4076096048073,6.2956620395348));
#47832=CARTESIAN_POINT('Ctrl Pts',(-9.94449673701248,13.6085552867894,6.34799541531888));
#47833=CARTESIAN_POINT('Ctrl Pts',(-9.99523417179805,13.4079201262562,6.36113584271526));
#47834=CARTESIAN_POINT('Ctrl Pts',(-10.0188913666349,13.2004368082823,6.37427627011165));
#47835=CARTESIAN_POINT('Ctrl Pts',(-10.0170827477036,12.9925476830062,6.38741669750803));
#47836=CARTESIAN_POINT('Origin',(-7.5,12.9903810567666,7.5));
#47837=CARTESIAN_POINT('',(-10.0145080012689,12.9889431840086,7.38741669750803));
#47838=CARTESIAN_POINT('',(-10.0189159587739,12.9883983308864,7.11258330249199));
#47839=CARTESIAN_POINT('',(-10.0175,12.9903810567666,7.5));
#47840=CARTESIAN_POINT('Ctrl Pts',(-10.0189159587739,12.9883983308864,7.11258330249199));
#47841=CARTESIAN_POINT('Ctrl Pts',(-10.0130302121016,13.6704662986594,7.06938967489226));
#47842=CARTESIAN_POINT('Ctrl Pts',(-9.72554840383075,14.3569089324365,7.02619604729254));
#47843=CARTESIAN_POINT('Ctrl Pts',(-9.2308848153494,14.8238864031427,6.98300241969281));
#47844=CARTESIAN_POINT('Ctrl Pts',(-8.63155067970796,15.3896760534967,6.93066904390873));
#47845=CARTESIAN_POINT('Ctrl Pts',(-7.72807923358486,15.6332967159553,6.87833566812465));
#47846=CARTESIAN_POINT('Ctrl Pts',(-6.9255462333781,15.4455199330078,6.82600229234057));
#47847=CARTESIAN_POINT('Ctrl Pts',(-6.12301323317133,15.2577431500604,6.77366891655648));
#47848=CARTESIAN_POINT('Ctrl Pts',(-5.4214186788809,14.638568921707,6.72133554077239));
#47849=CARTESIAN_POINT('Ctrl Pts',(-5.13532585476554,13.8656069146025,6.66900216498831));
#47850=CARTESIAN_POINT('Ctrl Pts',(-4.84923303065017,13.092644907498,6.61666878920422));
#47851=CARTESIAN_POINT('Ctrl Pts',(-4.97864193670987,12.1658951216425,6.56433541342014));
#47852=CARTESIAN_POINT('Ctrl Pts',(-5.46553146829354,11.5008704033029,6.51200203763605));
#47853=CARTESIAN_POINT('Ctrl Pts',(-5.95242099987721,10.8358456849633,6.45966866185197));
#47854=CARTESIAN_POINT('Ctrl Pts',(-6.79679115698486,10.4325460341398,6.40733528606789));
#47855=CARTESIAN_POINT('Ctrl Pts',(-7.62006453112491,10.471792520931,6.35500191028381));
#47856=CARTESIAN_POINT('Ctrl Pts',(-8.44333790526497,10.5110390077222,6.30266853449972));
#47857=CARTESIAN_POINT('Ctrl Pts',(-9.24551449643742,10.9928316321281,6.25033515871563));
#47858=CARTESIAN_POINT('Ctrl Pts',(-9.66693457878153,11.7011568743055,6.19800178293155));
#47859=CARTESIAN_POINT('Ctrl Pts',(-9.89621504923482,12.0865327772692,6.16952895611836));
#47860=CARTESIAN_POINT('Ctrl Pts',(-10.0127884887617,12.5389641820168,6.14105612930517));
#47861=CARTESIAN_POINT('Ctrl Pts',(-10.0137187170915,12.9909479514162,6.11258330249198));
#47862=CARTESIAN_POINT('Ctrl Pts',(-10.0170827477036,12.9925476830062,6.38741669750803));
#47863=CARTESIAN_POINT('Ctrl Pts',(-10.0116883182615,12.3724926793498,6.42660964589573));
#47864=CARTESIAN_POINT('Ctrl Pts',(-9.77974890631033,11.7488275963524,6.46580259428343));
#47865=CARTESIAN_POINT('Ctrl Pts',(-9.36410096710587,11.2924908434457,6.50499554267113));
#47866=CARTESIAN_POINT('Ctrl Pts',(-8.80909654179214,10.6831556503463,6.55732891845521));
#47867=CARTESIAN_POINT('Ctrl Pts',(-7.92654713908917,10.3721601963736,6.6096622942393));
#47868=CARTESIAN_POINT('Ctrl Pts',(-7.11214799700031,10.4989408139477,6.66199567002338));
#47869=CARTESIAN_POINT('Ctrl Pts',(-6.29774885491145,10.6257214315218,6.71432904580747));
#47870=CARTESIAN_POINT('Ctrl Pts',(-5.55149997343671,11.1902781206427,6.76666242159156));
#47871=CARTESIAN_POINT('Ctrl Pts',(-5.20798562845119,11.9394891669376,6.81899579737564));
#47872=CARTESIAN_POINT('Ctrl Pts',(-4.86447128346568,12.6887002132326,6.87132917315972));
#47873=CARTESIAN_POINT('Ctrl Pts',(-4.92369147496937,13.6225656167016,6.92366254894381));
#47874=CARTESIAN_POINT('Ctrl Pts',(-5.35909454078469,14.3223823516912,6.97599592472789));
#47875=CARTESIAN_POINT('Ctrl Pts',(-5.79449760660002,15.0221990866808,7.02832930051197));
#47876=CARTESIAN_POINT('Ctrl Pts',(-6.60608354672698,15.4879671531909,7.08066267629606));
#47877=CARTESIAN_POINT('Ctrl Pts',(-7.42997391459192,15.5108572005546,7.13299605208014));
#47878=CARTESIAN_POINT('Ctrl Pts',(-8.25386428245684,15.5337472479183,7.18532942786423));
#47879=CARTESIAN_POINT('Ctrl Pts',(-9.09005907805975,15.1137592761355,7.23766280364831));
#47880=CARTESIAN_POINT('Ctrl Pts',(-9.56364635237551,14.4391969089269,7.2899961794324));
#47881=CARTESIAN_POINT('Ctrl Pts',(-9.85751310519891,14.0206226287906,7.32246968545761));
#47882=CARTESIAN_POINT('Ctrl Pts',(-10.0117630617271,13.5040281493434,7.35494319148282));
#47883=CARTESIAN_POINT('Ctrl Pts',(-10.0145080012689,12.9889431840086,7.38741669750803));
#47884=CARTESIAN_POINT('Origin',(-7.5,12.9903810567666,7.5));
#47885=CARTESIAN_POINT('',(-10.0214370846894,12.9902333726245,8.38741669750803));
#47886=CARTESIAN_POINT('',(-10.0184390483887,12.992460268524,8.11258330249199));
#47887=CARTESIAN_POINT('',(-10.0175,12.9903810567666,7.5));
#47888=CARTESIAN_POINT('Ctrl Pts',(-10.0184390483887,12.992460268524,8.11258330249199));
#47889=CARTESIAN_POINT('Ctrl Pts',(-10.0198617859934,13.1535014782239,8.10238997204752));
#47890=CARTESIAN_POINT('Ctrl Pts',(-10.0057048345233,13.3142936934228,8.09219664160306));
#47891=CARTESIAN_POINT('Ctrl Pts',(-9.9750487925512,13.4718761813451,8.08200331115859));
#47892=CARTESIAN_POINT('Ctrl Pts',(-9.8176582151223,14.2809173090076,8.02966993537451));
#47893=CARTESIAN_POINT('Ctrl Pts',(-9.22537175290504,15.0053539438514,7.97733655959042));
#47894=CARTESIAN_POINT('Ctrl Pts',(-8.46374388225838,15.3203814452906,7.92500318380634));
#47895=CARTESIAN_POINT('Ctrl Pts',(-7.70211601161172,15.6354089467299,7.87266980802225));
#47896=CARTESIAN_POINT('Ctrl Pts',(-6.77114673253565,15.5410273147647,7.82033643223817));
#47897=CARTESIAN_POINT('Ctrl Pts',(-6.08824058698168,15.0795530074754,7.76800305645409));
#47898=CARTESIAN_POINT('Ctrl Pts',(-5.40533444142772,14.6180787001861,7.71566968067));
#47899=CARTESIAN_POINT('Ctrl Pts',(-4.97049142939586,13.7895117175727,7.66333630488591));
#47900=CARTESIAN_POINT('Ctrl Pts',(-4.97867550117357,12.9653440395039,7.61100292910182));
#47901=CARTESIAN_POINT('Ctrl Pts',(-4.98685957295128,12.1411763614351,7.55866955331774));
#47902=CARTESIAN_POINT('Ctrl Pts',(-5.43807072853852,11.3214079879109,7.50633617753367));
#47903=CARTESIAN_POINT('Ctrl Pts',(-6.13000628195668,10.8735860038557,7.45400280174958));
#47904=CARTESIAN_POINT('Ctrl Pts',(-6.82194183537485,10.4257640198005,7.4016694259655));
#47905=CARTESIAN_POINT('Ctrl Pts',(-7.75460178662392,10.3498884252143,7.3493360501814));
#47906=CARTESIAN_POINT('Ctrl Pts',(-8.50982357282137,10.6799784021981,7.29700267439732));
#47907=CARTESIAN_POINT('Ctrl Pts',(-9.2650453590188,11.0100683791819,7.24466929861323));
#47908=CARTESIAN_POINT('Ctrl Pts',(-9.84282898016461,11.7461239277358,7.19233592282916));
#47909=CARTESIAN_POINT('Ctrl Pts',(-9.98412237815762,12.5581310211375,7.14000254704507));
#47910=CARTESIAN_POINT('Ctrl Pts',(-10.0087985252324,12.6999437791798,7.13086279886071));
#47911=CARTESIAN_POINT('Ctrl Pts',(-10.020161379579,12.8440731186622,7.12172305067635));
#47912=CARTESIAN_POINT('Ctrl Pts',(-10.0189159587739,12.9883983308864,7.11258330249199));
#47913=CARTESIAN_POINT('Ctrl Pts',(-10.0145080012689,12.9889431840086,7.38741669750803));
#47914=CARTESIAN_POINT('Ctrl Pts',(-10.0161867279748,12.6739319154882,7.4072765672669));
#47915=CARTESIAN_POINT('Ctrl Pts',(-9.96119959962244,12.359485234924,7.42713643702578));
#47916=CARTESIAN_POINT('Ctrl Pts',(-9.84682730754632,12.0683695443894,7.44699630678465));
#47917=CARTESIAN_POINT('Ctrl Pts',(-9.54544123537271,11.3012413096949,7.49932968256874));
#47918=CARTESIAN_POINT('Ctrl Pts',(-8.83168933799688,10.6961216029404,7.55166305835282));
#47919=CARTESIAN_POINT('Ctrl Pts',(-8.02558570196195,10.5243187478344,7.60399643413691));
#47920=CARTESIAN_POINT('Ctrl Pts',(-7.21948206592701,10.3525158927284,7.65632980992099));
#47921=CARTESIAN_POINT('Ctrl Pts',(-6.32102669123297,10.6140298892709,7.70866318570508));
#47922=CARTESIAN_POINT('Ctrl Pts',(-5.73304635500187,11.1916096823396,7.76099656148916));
#47923=CARTESIAN_POINT('Ctrl Pts',(-5.14506601877077,11.7691894754082,7.81332993727325));
#47924=CARTESIAN_POINT('Ctrl Pts',(-4.8675607210026,12.6628350650029,7.86566331305733));
#47925=CARTESIAN_POINT('Ctrl Pts',(-5.02495129299175,13.4718761647033,7.91799668884141));
#47926=CARTESIAN_POINT('Ctrl Pts',(-5.18234186498089,14.2809172644038,7.9703300646255));
#47927=CARTESIAN_POINT('Ctrl Pts',(-5.77462830672734,15.0053538742101,8.02266344040958));
#47928=CARTESIAN_POINT('Ctrl Pts',(-6.53625615105054,15.3203813647611,8.07499681619367));
#47929=CARTESIAN_POINT('Ctrl Pts',(-7.29788399537374,15.6354088553122,8.12733019197775));
#47930=CARTESIAN_POINT('Ctrl Pts',(-8.22885324227368,15.5410272266082,8.17966356776184));
#47931=CARTESIAN_POINT('Ctrl Pts',(-8.91175936422494,15.0795529352688,8.23199694354592));
#47932=CARTESIAN_POINT('Ctrl Pts',(-9.58779130918474,14.6227238738573,8.28380352819996));
#47933=CARTESIAN_POINT('Ctrl Pts',(-10.0207290328118,13.8061553106607,8.33561011285399));
#47934=CARTESIAN_POINT('Ctrl Pts',(-10.0214370846894,12.9902333726245,8.38741669750803));
#47935=CARTESIAN_POINT('Origin',(-7.5,12.9903810567666,7.5));
#47936=CARTESIAN_POINT('',(-10.0148245050326,12.9920058624485,9.38741669750802));
#47937=CARTESIAN_POINT('',(-10.0138587145805,12.9895659971561,9.11258330249198));
#47938=CARTESIAN_POINT('',(-10.0175,12.9903810567666,7.5));
#47939=CARTESIAN_POINT('Ctrl Pts',(-10.0138587145805,12.9895659971561,9.11258330249198));
#47940=CARTESIAN_POINT('Ctrl Pts',(-10.0124665205819,13.458209000479,9.08305689341869));
#47941=CARTESIAN_POINT('Ctrl Pts',(-9.88655927300326,13.9275468726326,9.0535304843454));
#47942=CARTESIAN_POINT('Ctrl Pts',(-9.64090553321082,14.3223823977307,9.02400407527211));
#47943=CARTESIAN_POINT('Ctrl Pts',(-9.20550245234811,15.0221991569096,8.97167069948803));
#47944=CARTESIAN_POINT('Ctrl Pts',(-8.39391648416845,15.4879672395126,8.91933732370394));
#47945=CARTESIAN_POINT('Ctrl Pts',(-7.57002608782754,15.5108572876662,8.86700394791986));
#47946=CARTESIAN_POINT('Ctrl Pts',(-6.74613569148664,15.5337473358198,8.81467057213577));
#47947=CARTESIAN_POINT('Ctrl Pts',(-5.90994086698447,15.113759349524,8.76233719635169));
#47948=CARTESIAN_POINT('Ctrl Pts',(-5.43635357630086,14.4391969590017,8.71000382056761));
#47949=CARTESIAN_POINT('Ctrl Pts',(-4.96276628561725,13.7646345684795,8.65767044478352));
#47950=CARTESIAN_POINT('Ctrl Pts',(-4.85178652875219,12.8354977737306,8.60533706899943));
#47951=CARTESIAN_POINT('Ctrl Pts',(-5.15317261134217,12.0683695125223,8.55300369321535));
#47952=CARTESIAN_POINT('Ctrl Pts',(-5.45455869393216,11.3012412513139,8.50067031743126));
#47953=CARTESIAN_POINT('Ctrl Pts',(-6.16831061597719,10.696121523646,8.44833694164718));
#47954=CARTESIAN_POINT('Ctrl Pts',(-6.97441427987286,10.5243186626023,8.3960035658631));
#47955=CARTESIAN_POINT('Ctrl Pts',(-7.78051794376854,10.3525158015586,8.34367019007901));
#47956=CARTESIAN_POINT('Ctrl Pts',(-8.67897334951486,10.6140298071391,8.29133681429493));
#47957=CARTESIAN_POINT('Ctrl Pts',(-9.26695370606775,11.1916096201701,8.23900343851084));
#47958=CARTESIAN_POINT('Ctrl Pts',(-9.74040909687172,11.656690252629,8.19686339317122));
#47959=CARTESIAN_POINT('Ctrl Pts',(-10.0125573370586,12.3267029956413,8.15472334783161));
#47960=CARTESIAN_POINT('Ctrl Pts',(-10.0184390483887,12.992460268524,8.11258330249199));
#47961=CARTESIAN_POINT('Ctrl Pts',(-10.0214370846894,12.9902333726245,8.38741669750803));
#47962=CARTESIAN_POINT('Ctrl Pts',(-10.0214442844586,12.9819367353796,8.38794348863807));
#47963=CARTESIAN_POINT('Ctrl Pts',(-10.0214067930746,12.9736401649937,8.38847027976812));
#47964=CARTESIAN_POINT('Ctrl Pts',(-10.021324411684,12.9653440403702,8.38899707089817));
#47965=CARTESIAN_POINT('Ctrl Pts',(-10.0131403401893,12.1411763907856,8.44133044668226));
#47966=CARTESIAN_POINT('Ctrl Pts',(-9.56192920019726,11.3214080455913,8.49366382246634));
#47967=CARTESIAN_POINT('Ctrl Pts',(-8.86999367069368,10.873586077015,8.54599719825042));
#47968=CARTESIAN_POINT('Ctrl Pts',(-8.1780581411901,10.4257641084388,8.59833057403451));
#47969=CARTESIAN_POINT('Ctrl Pts',(-7.24539822217496,10.3498885164806,8.65066394981859));
#47970=CARTESIAN_POINT('Ctrl Pts',(-6.49017646207993,10.6799784820534,8.70299732560268));
#47971=CARTESIAN_POINT('Ctrl Pts',(-5.7349547019849,11.0100684476262,8.75533070138676));
#47972=CARTESIAN_POINT('Ctrl Pts',(-5.15717110080998,11.7461239707299,8.80766407717085));
#47973=CARTESIAN_POINT('Ctrl Pts',(-5.01587770769964,12.5581310360714,8.85999745295494));
#47974=CARTESIAN_POINT('Ctrl Pts',(-4.8745843145893,13.3701381014129,8.91233082873902));
#47975=CARTESIAN_POINT('Ctrl Pts',(-5.16978112954355,14.2580967089923,8.96466420452309));
#47976=CARTESIAN_POINT('Ctrl Pts',(-5.76911524447212,14.823886339783,9.01699758030718));
#47977=CARTESIAN_POINT('Ctrl Pts',(-6.36844935940068,15.3896759705738,9.06933095609126));
#47978=CARTESIAN_POINT('Ctrl Pts',(-7.27192077430355,15.633296624576,9.12166433187536));
#47979=CARTESIAN_POINT('Ctrl Pts',(-8.07445374677037,15.4455198481341,9.17399770765944));
#47980=CARTESIAN_POINT('Ctrl Pts',(-8.87698671923719,15.2577430716922,9.22633108344353));
#47981=CARTESIAN_POINT('Ctrl Pts',(-9.57858124926796,14.6385688648061,9.2786644592276));
#47982=CARTESIAN_POINT('Ctrl Pts',(-9.8646740635007,13.8656068843882,9.33099783501169));
#47983=CARTESIAN_POINT('Ctrl Pts',(-9.96748309569448,13.5878387295239,9.34980412251046));
#47984=CARTESIAN_POINT('Ctrl Pts',(-10.0166357361991,13.2902109767329,9.36861041000924));
#47985=CARTESIAN_POINT('Ctrl Pts',(-10.0148245050326,12.9920058624485,9.38741669750802));
#47986=CARTESIAN_POINT('Origin',(-7.5,12.9903810567666,7.5));
#47987=CARTESIAN_POINT('',(-10.0166112816083,12.988245230306,10.387416697508));
#47988=CARTESIAN_POINT('',(-10.0209918820407,12.9894441341194,10.112583302492));
#47989=CARTESIAN_POINT('',(-10.0175,12.9903810567666,7.5));
#47990=CARTESIAN_POINT('Ctrl Pts',(-10.0209918820407,12.9894441341194,10.112583302492));
#47991=CARTESIAN_POINT('Ctrl Pts',(-10.0172624812131,13.7593153446234,10.0637238147899));
#47992=CARTESIAN_POINT('Ctrl Pts',(-9.63824829706051,14.5323682430672,10.0148643270877));
#47993=CARTESIAN_POINT('Ctrl Pts',(-9.02557849846605,14.9979452399236,9.96600483938563));
#47994=CARTESIAN_POINT('Ctrl Pts',(-8.36934814670953,15.4966245564456,9.91367146360154));
#47995=CARTESIAN_POINT('Ctrl Pts',(-7.44505539412875,15.642550832678,9.86133808781746));
#47996=CARTESIAN_POINT('Ctrl Pts',(-6.66711117965626,15.3702971070154,9.80900471203338));
#47997=CARTESIAN_POINT('Ctrl Pts',(-5.88916696518377,15.0980433813528,9.75667133624929));
#47998=CARTESIAN_POINT('Ctrl Pts',(-5.25757128881956,14.4076096537953,9.70433796046521));
#47999=CARTESIAN_POINT('Ctrl Pts',(-5.05550317851592,13.608555308187,9.65200458468112));
#48000=CARTESIAN_POINT('Ctrl Pts',(-4.85343506821227,12.8095009625786,9.59967120889704));
#48001=CARTESIAN_POINT('Ctrl Pts',(-5.08089452396919,11.9018259989194,9.54733783311296));
#48002=CARTESIAN_POINT('Ctrl Pts',(-5.6358989684585,11.2924907847457,9.49500445732887));
#48003=CARTESIAN_POINT('Ctrl Pts',(-6.19090341294781,10.683155570572,9.44267108154479));
#48004=CARTESIAN_POINT('Ctrl Pts',(-7.0734528461695,10.3721601058839,9.3903377057607));
#48005=CARTESIAN_POINT('Ctrl Pts',(-7.88785201640932,10.4989407278476,9.33800432997662));
#48006=CARTESIAN_POINT('Ctrl Pts',(-8.70225118664915,10.6257213498112,9.28567095419253));
#48007=CARTESIAN_POINT('Ctrl Pts',(-9.44850009390711,11.1902780584266,9.23333757840845));
#48008=CARTESIAN_POINT('Ctrl Pts',(-9.79201445076321,11.9394891306117,9.18100420262436));
#48009=CARTESIAN_POINT('Ctrl Pts',(-9.9417185427335,12.2659964832652,9.15819723591357));
#48010=CARTESIAN_POINT('Ctrl Pts',(-10.014934081453,12.6275739462602,9.13539026920278));
#48011=CARTESIAN_POINT('Ctrl Pts',(-10.0138587145805,12.9895659971561,9.11258330249198));
#48012=CARTESIAN_POINT('Ctrl Pts',(-10.0148245050326,12.9920058624485,9.38741669750802));
#48013=CARTESIAN_POINT('Ctrl Pts',(-10.0115955154073,12.4603778526996,9.42094378579333));
#48014=CARTESIAN_POINT('Ctrl Pts',(-9.84639154112273,11.9269148544392,9.45447087407864));
#48015=CARTESIAN_POINT('Ctrl Pts',(-9.53446846140197,11.5008704547181,9.48799796236395));
#48016=CARTESIAN_POINT('Ctrl Pts',(-9.0475789466358,10.8358457594159,9.54033133814803));
#48017=CARTESIAN_POINT('Ctrl Pts',(-8.20320881866876,10.4325461227612,9.59266471393211));
#48018=CARTESIAN_POINT('Ctrl Pts',(-7.37993547300324,10.4717926080996,9.64499808971619));
#48019=CARTESIAN_POINT('Ctrl Pts',(-6.55666212733773,10.5110390934381,9.69733146550028));
#48020=CARTESIAN_POINT('Ctrl Pts',(-5.75448556397372,10.9928317007697,9.74966484128437));
#48021=CARTESIAN_POINT('Ctrl Pts',(-5.33306549615464,11.7011569186411,9.80199821706845));
#48022=CARTESIAN_POINT('Ctrl Pts',(-4.91164542833556,12.4094821365125,9.85433159285254));
#48023=CARTESIAN_POINT('Ctrl Pts',(-4.87098185606138,13.3443399649238,9.90666496863662));
#48024=CARTESIAN_POINT('Ctrl Pts',(-5.22930648076992,14.0865814044601,9.9589983444207));
#48025=CARTESIAN_POINT('Ctrl Pts',(-5.58763110547847,14.8288228439964,10.0113317202048));
#48026=CARTESIAN_POINT('Ctrl Pts',(-6.34494392716974,15.3784478946578,10.0636650959889));
#48027=CARTESIAN_POINT('Ctrl Pts',(-7.1617001217923,15.489031500081,10.115998471773));
#48028=CARTESIAN_POINT('Ctrl Pts',(-7.97845631641486,15.5996151055041,10.168331847557));
#48029=CARTESIAN_POINT('Ctrl Pts',(-8.8546558839687,15.2711572656891,10.2206652233411));
#48030=CARTESIAN_POINT('Ctrl Pts',(-9.39745052149691,14.6509197715574,10.2729985991252));
#48031=CARTESIAN_POINT('Ctrl Pts',(-9.79302682634298,14.1989048858303,10.3111379652528));
#48032=CARTESIAN_POINT('Ctrl Pts',(-10.0115264151771,13.5919211369207,10.3492773313804));
#48033=CARTESIAN_POINT('Ctrl Pts',(-10.0166112816083,12.988245230306,10.387416697508));
#48034=CARTESIAN_POINT('Origin',(-7.5,12.9903810567666,7.5));
#48035=CARTESIAN_POINT('',(-10.020507596494,12.9916292754481,11.387416697508));
#48036=CARTESIAN_POINT('',(-10.0159019782719,12.9923925656114,11.112583302492));
#48037=CARTESIAN_POINT('',(-10.0175,12.9903810567666,7.5));
#48038=CARTESIAN_POINT('',(-5.58653400333491,14.6263682601415,12.));
#48039=CARTESIAN_POINT('Ctrl Pts',(-10.020507596494,12.9916292754481,11.387416697508));
#48040=CARTESIAN_POINT('Ctrl Pts',(-10.0157033908479,12.2477735308672,11.4346110043198));
#48041=CARTESIAN_POINT('Ctrl Pts',(-9.66521700262529,11.5001788657538,11.4818053111315));
#48042=CARTESIAN_POINT('Ctrl Pts',(-9.08783233623607,11.0319150553912,11.5289996179432));
#48043=CARTESIAN_POINT('Ctrl Pts',(-8.44757526373259,10.5126611959891,11.5813329937273));
#48044=CARTESIAN_POINT('Ctrl Pts',(-7.52831480323821,10.3368839617759,11.6336663695114));
#48045=CARTESIAN_POINT('Ctrl Pts',(-6.74219715513642,10.5850674081367,11.6859997452955));
#48046=CARTESIAN_POINT('Ctrl Pts',(-5.95607950703463,10.8332508544976,11.7383331210796));
#48047=CARTESIAN_POINT('Ctrl Pts',(-5.30310467132541,11.5053949814325,11.7906664968637));
#48048=CARTESIAN_POINT('Ctrl Pts',(-5.07623184554712,12.2963777181293,11.8429998726477));
#48049=CARTESIAN_POINT('Ctrl Pts',(-4.84935901976883,13.0873604548261,11.8953332484318));
#48050=CARTESIAN_POINT('Ctrl Pts',(-5.04858820392146,13.9971818012847,11.9476666242159));
#48051=CARTESIAN_POINT('Ctrl Pts',(-5.58653400333491,14.6263682601415,12.));
#48052=CARTESIAN_POINT('',(-9.41699350863879,14.6286916542883,12.));
#48053=CARTESIAN_POINT('Origin',(-7.5,12.9903810567666,12.));
#48054=CARTESIAN_POINT('Ctrl Pts',(-9.41700728965905,14.6287007311509,12.));
#48055=CARTESIAN_POINT('Ctrl Pts',(-8.90328417076102,15.2258393704274,11.9500021225376));
#48056=CARTESIAN_POINT('Ctrl Pts',(-8.08591167026785,15.5661089832965,11.9000042450751));
#48057=CARTESIAN_POINT('Ctrl Pts',(-7.30082070927967,15.5037710574514,11.8500063676127));
#48058=CARTESIAN_POINT('Ctrl Pts',(-6.47905661905513,15.438521205569,11.7976729918286));
#48059=CARTESIAN_POINT('Ctrl Pts',(-5.6926603741346,14.9321721568753,11.7453396160445));
#48060=CARTESIAN_POINT('Ctrl Pts',(-5.29374195236929,14.2110639499398,11.6930062402604));
#48061=CARTESIAN_POINT('Ctrl Pts',(-4.89482353060398,13.4899557430043,11.6406728644763));
#48062=CARTESIAN_POINT('Ctrl Pts',(-4.88338293199389,12.554088377827,11.5883394886922));
#48063=CARTESIAN_POINT('Ctrl Pts',(-5.26479155556264,11.8234099202509,11.5360061129082));
#48064=CARTESIAN_POINT('Ctrl Pts',(-5.64620017913138,11.0927314626748,11.4836727371241));
#48065=CARTESIAN_POINT('Ctrl Pts',(-6.42045802487898,10.5672419126997,11.43133936134));
#48066=CARTESIAN_POINT('Ctrl Pts',(-7.24029926801916,10.482369652534,11.3790059855559));
#48067=CARTESIAN_POINT('Ctrl Pts',(-8.06014051115934,10.3974973923684,11.3266726097718));
#48068=CARTESIAN_POINT('Ctrl Pts',(-8.92556515169212,10.753242422012,11.2743392339877));
#48069=CARTESIAN_POINT('Ctrl Pts',(-9.44861906997071,11.3901953896836,11.2220058582037));
#48070=CARTESIAN_POINT('Ctrl Pts',(-9.81316588581269,11.8341251034117,11.1855316729664));
#48071=CARTESIAN_POINT('Ctrl Pts',(-10.0114057826858,12.4146518528183,11.1490574877292));
#48072=CARTESIAN_POINT('Ctrl Pts',(-10.0159019782719,12.9923925656114,11.112583302492));
#48073=CARTESIAN_POINT('Origin',(-7.5,12.9903810567666,14.2084234471775));
#48074=CARTESIAN_POINT('',(-10.5774088918681,12.99185618799,4.79157655282255));
#48075=CARTESIAN_POINT('',(-10.5686791348591,12.9902767031652,4.70842344717746));
#48076=CARTESIAN_POINT('',(-10.5735,12.9903810567666,14.2084234471775));
#48077=CARTESIAN_POINT('',(-6.70620071746715,10.0211581030209,4.));
#48078=CARTESIAN_POINT('Ctrl Pts',(-10.5686791348591,12.9902767031652,4.70842344717746));
#48079=CARTESIAN_POINT('Ctrl Pts',(-10.568341542465,13.509926201974,4.68161580125464));
#48080=CARTESIAN_POINT('Ctrl Pts',(-10.1982938594512,15.0443643081101,4.60247477954774));
#48081=CARTESIAN_POINT('Ctrl Pts',(-7.78634777823694,16.5973803971072,4.47100038205676));
#48082=CARTESIAN_POINT('Ctrl Pts',(-4.64704915358778,15.2208104036021,4.31400025470451));
#48083=CARTESIAN_POINT('Ctrl Pts',(-4.07060765975928,11.8373819589561,4.15700012735225));
#48084=CARTESIAN_POINT('Ctrl Pts',(-5.72985994157694,10.2821754194981,4.05233337578409));
#48085=CARTESIAN_POINT('Ctrl Pts',(-6.70620071746715,10.0211581030209,4.));
#48086=CARTESIAN_POINT('',(-8.29574161562937,10.0163810931058,4.00000000000001));
#48087=CARTESIAN_POINT('Origin',(-7.5,12.9903810567666,4.));
#48088=CARTESIAN_POINT('Ctrl Pts',(-10.5774088918681,12.99185618799,4.79157655282254));
#48089=CARTESIAN_POINT('Ctrl Pts',(-10.5779243576744,13.0789760377035,4.78704908248048));
#48090=CARTESIAN_POINT('Ctrl Pts',(-10.535392897551,14.1726059842126,4.73018823635432));
#48091=CARTESIAN_POINT('Ctrl Pts',(-9.2319528795399,16.1681374132995,4.62099401444409));
#48092=CARTESIAN_POINT('Ctrl Pts',(-5.80479653057489,16.1883357805992,4.46399388709183));
#48093=CARTESIAN_POINT('Ctrl Pts',(-3.89775210281319,13.3398493780975,4.30699375973959));
#48094=CARTESIAN_POINT('Ctrl Pts',(-5.2011833457958,10.227049143879,4.15232913070897));
#48095=CARTESIAN_POINT('Ctrl Pts',(-7.36594149062469,9.77083767708475,4.04999787746245));
#48096=CARTESIAN_POINT('Ctrl Pts',(-8.29574920379123,10.0163624306404,4.00000000000001));
#48097=CARTESIAN_POINT('Origin',(-7.5,12.9903810567666,14.2084234471775));
#48098=CARTESIAN_POINT('',(-10.5688836055535,12.9910731523796,5.79157655282255));
#48099=CARTESIAN_POINT('',(-10.5767201283484,12.9885005040359,5.70842344717746));
#48100=CARTESIAN_POINT('',(-10.5735,12.9903810567666,14.2084234471775));
#48101=CARTESIAN_POINT('Ctrl Pts',(-10.5767201283484,12.9885005040358,5.70842344717746));
#48102=CARTESIAN_POINT('Ctrl Pts',(-10.5702728094234,13.8768977505312,5.66228272262582));
#48103=CARTESIAN_POINT('Ctrl Pts',(-9.70223158388916,15.7839304785174,5.56380862229009));
#48104=CARTESIAN_POINT('Ctrl Pts',(-6.48106323809927,16.4631861795336,5.41300114617029));
#48105=CARTESIAN_POINT('Ctrl Pts',(-4.04127258839909,14.0562954080889,5.25600101881802));
#48106=CARTESIAN_POINT('Ctrl Pts',(-4.70303600953422,10.693474125437,5.09900089146578));
#48107=CARTESIAN_POINT('Ctrl Pts',(-7.87270732364685,9.390536089231,4.94200076411351));
#48108=CARTESIAN_POINT('Ctrl Pts',(-10.2242696810485,10.9865434678639,4.81180828268408));
#48109=CARTESIAN_POINT('Ctrl Pts',(-10.5690005839068,12.4954763477989,4.73394917703873));
#48110=CARTESIAN_POINT('Ctrl Pts',(-10.5686791348591,12.9902767031652,4.70842344717746));
#48111=CARTESIAN_POINT('Ctrl Pts',(-10.5688836055535,12.9910731523796,5.79157655282255));
#48112=CARTESIAN_POINT('Ctrl Pts',(-10.5698353122932,13.4534929538237,5.76771600385165));
#48113=CARTESIAN_POINT('Ctrl Pts',(-10.2562652325398,14.9289132187583,5.69152207909668));
#48114=CARTESIAN_POINT('Ctrl Pts',(-7.98558646537732,16.576874141135,5.56299477855761));
#48115=CARTESIAN_POINT('Ctrl Pts',(-4.77645105419042,15.3738768659897,5.40599465120536));
#48116=CARTESIAN_POINT('Ctrl Pts',(-4.00954823259222,12.0335573562934,5.24899452385311));
#48117=CARTESIAN_POINT('Ctrl Pts',(-6.37256675930357,9.55126737969704,5.09199439650085));
#48118=CARTESIAN_POINT('Ctrl Pts',(-9.64926869943611,10.135445743826,4.93952173949067));
#48119=CARTESIAN_POINT('Ctrl Pts',(-10.571966049015,12.0719510350338,4.83938245826456));
#48120=CARTESIAN_POINT('Ctrl Pts',(-10.5774088918681,12.99185618799,4.79157655282254));
#48121=CARTESIAN_POINT('Origin',(-7.5,12.9903810567666,14.2084234471775));
#48122=CARTESIAN_POINT('',(-10.5752286789639,12.9879604379016,6.79157655282255));
#48123=CARTESIAN_POINT('',(-10.5729905958558,12.9930261911251,6.70842344717746));
#48124=CARTESIAN_POINT('',(-10.5735,12.9903810567666,14.2084234471775));
#48125=CARTESIAN_POINT('Ctrl Pts',(-10.5729905958558,12.9930261911251,6.70842344717746));
#48126=CARTESIAN_POINT('Ctrl Pts',(-10.5751986555521,13.2468284658167,6.69528301978108));
#48127=CARTESIAN_POINT('Ctrl Pts',(-10.4312906141563,14.5089611116288,6.62980921660061));
#48128=CARTESIAN_POINT('Ctrl Pts',(-8.69550582596531,16.4064477577484,6.51200203763606));
#48129=CARTESIAN_POINT('Ctrl Pts',(-5.31022637025923,15.8719837317436,6.3550019102838));
#48130=CARTESIAN_POINT('Ctrl Pts',(-3.88853720662811,12.7535599895385,6.19800178293155));
#48131=CARTESIAN_POINT('Ctrl Pts',(-5.70528280371351,9.84749392134933,6.04100165557929));
#48132=CARTESIAN_POINT('Ctrl Pts',(-9.13136573648253,9.75968890749465,5.88400152822705));
#48133=CARTESIAN_POINT('Ctrl Pts',(-10.5176205520478,11.7432796147819,5.77314212542643));
#48134=CARTESIAN_POINT('Ctrl Pts',(-10.5775854376359,12.8692666957923,5.7146160984099));
#48135=CARTESIAN_POINT('Ctrl Pts',(-10.5767201283484,12.9885005040358,5.70842344717746));
#48136=CARTESIAN_POINT('Ctrl Pts',(-10.5752286789639,12.9879604379016,6.79157655282255));
#48137=CARTESIAN_POINT('Ctrl Pts',(-10.5680430414674,13.8206658595303,6.74838292522283));
#48138=CARTESIAN_POINT('Ctrl Pts',(-9.79183063316292,15.6740884921896,6.65285592183902));
#48139=CARTESIAN_POINT('Ctrl Pts',(-6.67544470099851,16.5144205342573,6.50499554267113));
#48140=CARTESIAN_POINT('Ctrl Pts',(-4.10581110106408,14.2466564935293,6.34799541531888));
#48141=CARTESIAN_POINT('Ctrl Pts',(-4.57977925134152,10.8523778836063,6.19099528796662));
#48142=CARTESIAN_POINT('Ctrl Pts',(-7.67233735803906,9.3752678814539,6.03399516061438));
#48143=CARTESIAN_POINT('Ctrl Pts',(-10.1638445777963,10.8716837770844,5.90085558223301));
#48144=CARTESIAN_POINT('Ctrl Pts',(-10.5677479325558,12.4392669496988,5.82004937963574));
#48145=CARTESIAN_POINT('Ctrl Pts',(-10.5688836055535,12.9910731523796,5.79157655282255));
#48146=CARTESIAN_POINT('Origin',(-7.5,12.9903810567666,14.2084234471775));
#48147=CARTESIAN_POINT('',(-10.5746464410021,12.992919470803,7.79157655282256));
#48148=CARTESIAN_POINT('',(-10.5698472063158,12.988625624027,7.70842344717746));
#48149=CARTESIAN_POINT('',(-10.5735,12.9903810567666,14.2084234471775));
#48150=CARTESIAN_POINT('Ctrl Pts',(-10.5698472063158,12.988625624027,7.70842344717746));
#48151=CARTESIAN_POINT('Ctrl Pts',(-10.5664960358364,13.6174691755491,7.67594994115225));
#48152=CARTESIAN_POINT('Ctrl Pts',(-10.0746935678837,15.2645519082853,7.59114305934296));
#48153=CARTESIAN_POINT('Ctrl Pts',(-7.39948646190492,16.6082039047423,7.45400280174958));
#48154=CARTESIAN_POINT('Ctrl Pts',(-4.42700258466931,14.902299453002,7.29700267439732));
#48155=CARTESIAN_POINT('Ctrl Pts',(-4.21010495775379,11.4819594519348,7.14000254704507));
#48156=CARTESIAN_POINT('Ctrl Pts',(-6.94328780249567,9.41423553851335,6.98300241969282));
#48157=CARTESIAN_POINT('Ctrl Pts',(-9.90513850811741,10.4579415361298,6.83914271973694));
#48158=CARTESIAN_POINT('Ctrl Pts',(-10.5664047849758,12.2360295461447,6.74761639556516));
#48159=CARTESIAN_POINT('Ctrl Pts',(-10.5729905958558,12.9930261911251,6.70842344717746));
#48160=CARTESIAN_POINT('Ctrl Pts',(-10.5746464410021,12.992919470803,7.79157655282255));
#48161=CARTESIAN_POINT('Ctrl Pts',(-10.5763833959288,13.1895272793482,7.78138322237809));
#48162=CARTESIAN_POINT('Ctrl Pts',(-10.4703645847954,14.393670666495,7.71885651614954));
#48163=CARTESIAN_POINT('Ctrl Pts',(-8.88333173423194,16.3348001890992,7.6039964341369));
#48164=CARTESIAN_POINT('Ctrl Pts',(-5.47359896850368,15.9891216041795,7.44699630678466));
#48165=CARTESIAN_POINT('Ctrl Pts',(-3.88095944817013,12.9544436048999,7.28999617943239));
#48166=CARTESIAN_POINT('Ctrl Pts',(-5.53354831017302,9.95199105749957,7.13299605208015));
#48167=CARTESIAN_POINT('Ctrl Pts',(-8.9494732676674,9.67409198306777,6.97599592472789));
#48168=CARTESIAN_POINT('Ctrl Pts',(-10.4834447329667,11.6282633493619,6.86218942497536));
#48169=CARTESIAN_POINT('Ctrl Pts',(-10.5767491559627,12.8117604221037,6.80071630100691));
#48170=CARTESIAN_POINT('Ctrl Pts',(-10.5752286789639,12.9879604379016,6.79157655282255));
#48171=CARTESIAN_POINT('Origin',(-7.5,12.9903810567666,14.2084234471775));
#48172=CARTESIAN_POINT('',(-10.5690545220509,12.9893859879631,8.79157655282255));
#48173=CARTESIAN_POINT('',(-10.5783066056774,12.9902007559877,8.70842344717746));
#48174=CARTESIAN_POINT('',(-10.5735,12.9903810567666,14.2084234471775));
#48175=CARTESIAN_POINT('Ctrl Pts',(-10.5783066056774,12.9902007559877,8.70842344717746));
#48176=CARTESIAN_POINT('Ctrl Pts',(-10.5774421776949,13.9863223355525,8.65661686252342));
#48177=CARTESIAN_POINT('Ctrl Pts',(-9.51496009867182,15.9902813747918,8.5524769020853));
#48178=CARTESIAN_POINT('Ctrl Pts',(-6.11666831357863,16.3348000735102,8.3960035658631));
#48179=CARTESIAN_POINT('Ctrl Pts',(-3.9473824601037,13.6815060275445,8.23900343851085));
#48180=CARTESIAN_POINT('Ctrl Pts',(-4.9637628366961,10.4084735910568,8.08200331115859));
#48181=CARTESIAN_POINT('Ctrl Pts',(-8.25441140963209,9.45066234771208,7.92500318380633));
#48182=CARTESIAN_POINT('Ctrl Pts',(-10.3278657153401,11.208539372,7.80047656247929));
#48183=CARTESIAN_POINT('Ctrl Pts',(-10.5718966865663,12.6040428499268,7.72828331693633));
#48184=CARTESIAN_POINT('Ctrl Pts',(-10.5698472063158,12.988625624027,7.70842344717746));
#48185=CARTESIAN_POINT('Ctrl Pts',(-10.5690545220509,12.9893859879631,8.79157655282255));
#48186=CARTESIAN_POINT('Ctrl Pts',(-10.5673548564085,13.5615306833804,8.76205014374926));
#48187=CARTESIAN_POINT('Ctrl Pts',(-10.1411931381796,15.1501114670399,8.6801903588919));
#48188=CARTESIAN_POINT('Ctrl Pts',(-7.60051354156566,16.6082040297755,8.54599719825042));
#48189=CARTESIAN_POINT('Ctrl Pts',(-4.53789809794217,15.0699719631857,8.38899707089818));
#48190=CARTESIAN_POINT('Ctrl Pts',(-4.1314278504052,11.6669507850401,8.23199694354592));
#48191=CARTESIAN_POINT('Ctrl Pts',(-6.74558856429446,9.45066222537301,8.07499681619367));
#48192=CARTESIAN_POINT('Ctrl Pts',(-9.82258984821385,10.3462870118539,7.92819001928587));
#48193=CARTESIAN_POINT('Ctrl Pts',(-10.5674657300694,12.1801270266301,7.83371659816217));
#48194=CARTESIAN_POINT('Ctrl Pts',(-10.5746464410021,12.992919470803,7.79157655282255));
#48195=CARTESIAN_POINT('Origin',(-7.5,12.9903810567666,14.2084234471775));
#48196=CARTESIAN_POINT('',(-10.5777630782332,12.9892372109846,9.79157655282255));
#48197=CARTESIAN_POINT('',(-10.5702336112086,12.9923647073181,9.70842344717745));
#48198=CARTESIAN_POINT('',(-10.5735,12.9903810567666,14.2084234471775));
#48199=CARTESIAN_POINT('Ctrl Pts',(-10.5702336112086,12.9923647073181,9.70842344717746));
#48200=CARTESIAN_POINT('Ctrl Pts',(-10.5724448600627,13.3564296204275,9.68961715967868));
#48201=CARTESIAN_POINT('Ctrl Pts',(-10.3454482739325,14.7309332712505,9.61847749639582));
#48202=CARTESIAN_POINT('Ctrl Pts',(-8.32455527051676,16.5144204123725,9.49500445732887));
#48203=CARTESIAN_POINT('Ctrl Pts',(-5.01553513899265,15.6221446466417,9.33800432997661));
#48204=CARTESIAN_POINT('Ctrl Pts',(-3.93435848267263,12.3699411347509,9.18100420262437));
#48205=CARTESIAN_POINT('Ctrl Pts',(-6.0505267824277,9.67409209769908,9.02400407527211));
#48206=CARTESIAN_POINT('Ctrl Pts',(-9.46645162186327,9.95199116250562,8.86700394791985));
#48207=CARTESIAN_POINT('Ctrl Pts',(-10.573722513556,11.9637004181345,8.76181040522164));
#48208=CARTESIAN_POINT('Ctrl Pts',(-10.5783153955445,12.9800717730395,8.70895023830751));
#48209=CARTESIAN_POINT('Ctrl Pts',(-10.5783066056774,12.9902007559877,8.70842344717746));
#48210=CARTESIAN_POINT('Ctrl Pts',(-10.5777630782332,12.9892372109846,9.79157655282255));
#48211=CARTESIAN_POINT('Ctrl Pts',(-10.5732100242337,13.9291375746327,9.74271706512043));
#48212=CARTESIAN_POINT('Ctrl Pts',(-9.61486878320428,15.8838097348119,9.64152420163422));
#48213=CARTESIAN_POINT('Ctrl Pts',(-6.30449413259093,16.4064478755407,9.48799796236394));
#48214=CARTESIAN_POINT('Ctrl Pts',(-3.99123576757957,13.8776914962184,9.3309978350117));
#48215=CARTESIAN_POINT('Ctrl Pts',(-4.82432014168349,10.5532756064786,9.17399770765943));
#48216=CARTESIAN_POINT('Ctrl Pts',(-8.05671221676616,9.41423541495656,9.0169975803072));
#48217=CARTESIAN_POINT('Ctrl Pts',(-10.2758759707643,11.0930905163184,8.88952386202821));
#48218=CARTESIAN_POINT('Ctrl Pts',(-10.5703673880222,12.5474465367502,8.81438351953334));
#48219=CARTESIAN_POINT('Ctrl Pts',(-10.5690545220509,12.9893859879631,8.79157655282255));
#48220=CARTESIAN_POINT('Origin',(-7.5,12.9903810567666,14.2084234471775));
#48221=CARTESIAN_POINT('',(-10.5715490487462,12.9928368154298,10.7915765528225));
#48222=CARTESIAN_POINT('',(-10.5724150045772,12.9877735244422,10.7084234471775));
#48223=CARTESIAN_POINT('',(-10.5735,12.9903810567666,14.2084234471775));
#48224=CARTESIAN_POINT('Ctrl Pts',(-10.5724150045772,12.9877735244422,10.7084234471775));
#48225=CARTESIAN_POINT('Ctrl Pts',(-10.5662071249442,13.7247736829249,10.6702840810499));
#48226=CARTESIAN_POINT('Ctrl Pts',(-9.93341852875246,15.4826369193415,10.5798113391382));
#48227=CARTESIAN_POINT('Ctrl Pts',(-7.01441355218445,16.5768740138536,10.4370052214424));
#48228=CARTESIAN_POINT('Ctrl Pts',(-4.24070833971001,14.56383815303,10.2800050940901));
#48229=CARTESIAN_POINT('Ctrl Pts',(-4.38964119697082,11.1398633340167,10.1230049667379));
#48230=CARTESIAN_POINT('Ctrl Pts',(-7.32766264781398,9.3752680069458,9.96600483938563));
#48231=CARTESIAN_POINT('Ctrl Pts',(-10.0497780511113,10.6754420854925,9.82781099953215));
#48232=CARTESIAN_POINT('Ctrl Pts',(-10.5662914862381,12.3433245134896,9.74195053546276));
#48233=CARTESIAN_POINT('Ctrl Pts',(-10.5702336112086,12.9923647073181,9.70842344717746));
#48234=CARTESIAN_POINT('Ctrl Pts',(-10.5715490487462,12.9928368154298,10.7915765528225));
#48235=CARTESIAN_POINT('Ctrl Pts',(-10.5739357845658,13.2995215285911,10.7757173622757));
#48236=CARTESIAN_POINT('Ctrl Pts',(-10.391916652594,14.6154630132259,10.7075247959447));
#48237=CARTESIAN_POINT('Ctrl Pts',(-8.5189368031419,16.4631863186891,10.5869988538297));
#48238=CARTESIAN_POINT('Ctrl Pts',(-5.16549655959477,15.7560380892136,10.4299987264775));
#48239=CARTESIAN_POINT('Ctrl Pts',(-3.90540705298465,12.5688686867556,10.2729985991252));
#48240=CARTESIAN_POINT('Ctrl Pts',(-5.86863420589283,9.75968879265402,10.115998471773));
#48241=CARTESIAN_POINT('Ctrl Pts',(-9.29471725902464,9.84749381445728,9.9589983444207));
#48242=CARTESIAN_POINT('Ctrl Pts',(-10.5460795409153,11.8491727898316,9.85085770477057));
#48243=CARTESIAN_POINT('Ctrl Pts',(-10.5780867983696,12.9224107085984,9.79505044090452));
#48244=CARTESIAN_POINT('Ctrl Pts',(-10.5777630782332,12.9892372109846,9.79157655282255));
#48245=CARTESIAN_POINT('Origin',(-7.5,12.9903810567666,14.2084234471775));
#48246=CARTESIAN_POINT('',(-10.5702206634037,12.9870745539208,11.7915765528226));
#48247=CARTESIAN_POINT('',(-10.5771718362758,12.9919049495641,11.7084234471775));
#48248=CARTESIAN_POINT('',(-10.5735,12.9903810567666,14.2084234471775));
#48249=CARTESIAN_POINT('',(-8.29379928253292,10.0211581030209,12.));
#48250=CARTESIAN_POINT('Ctrl Pts',(-8.29379928253292,10.0211581030209,12.));
#48251=CARTESIAN_POINT('Ctrl Pts',(-9.27014005842312,10.2821754194981,11.9476666242159));
#48252=CARTESIAN_POINT('Ctrl Pts',(-10.3714991025232,11.3144735509882,11.8781921418234));
#48253=CARTESIAN_POINT('Ctrl Pts',(-10.5724953140326,12.655363779409,11.808717659431));
#48254=CARTESIAN_POINT('Ctrl Pts',(-10.5702206634037,12.9870745539208,11.7915765528226));
#48255=CARTESIAN_POINT('',(-6.70425858890745,10.0163809826708,12.));
#48256=CARTESIAN_POINT('Origin',(-7.5,12.9903810567666,12.));
#48257=CARTESIAN_POINT('Ctrl Pts',(-6.70425100699972,10.0163623331919,12.));
#48258=CARTESIAN_POINT('Ctrl Pts',(-7.63405880919358,9.77083750064795,11.9500021225376));
#48259=CARTESIAN_POINT('Ctrl Pts',(-9.69010226711413,10.2041387247117,11.8528099382634));
#48260=CARTESIAN_POINT('Ctrl Pts',(-10.5713066024909,12.0837656721183,11.7556177539892));
#48261=CARTESIAN_POINT('Ctrl Pts',(-10.5771718362758,12.9919049495641,11.7084234471775));
#48262=CARTESIAN_POINT('Origin',(15.,0.,7.5));
#48263=CARTESIAN_POINT('',(12.4864520394788,-8.37379766882585E-5,4.38741669750802));
#48264=CARTESIAN_POINT('',(12.4839933051997,-0.00316412607611227,4.11258330249198));
#48265=CARTESIAN_POINT('',(12.4825,3.08304831685346E-16,7.5));
#48266=CARTESIAN_POINT('',(13.086534003335,1.63598720337497,4.));
#48267=CARTESIAN_POINT('Ctrl Pts',(12.4839933051997,-0.00316412607611227,
4.11258330249198));
#48268=CARTESIAN_POINT('Ctrl Pts',(12.4891843965477,0.589325119423629,4.07505553499466));
#48269=CARTESIAN_POINT('Ctrl Pts',(12.700778171916,1.18480356030443,4.03752776749733));
#48270=CARTESIAN_POINT('Ctrl Pts',(13.086534003335,1.63598720337497,4.));
#48271=CARTESIAN_POINT('',(12.4825,3.08304831685346E-16,4.));
#48272=CARTESIAN_POINT('Origin',(15.,0.,4.));
#48273=CARTESIAN_POINT('',(12.4825,-3.08304831685346E-16,3.));
#48274=CARTESIAN_POINT('',(12.4825,3.08304831685346E-16,7.5));
#48275=CARTESIAN_POINT('Origin',(15.,0.,3.));
#48276=CARTESIAN_POINT('',(16.9169900003259,1.63831767401966,4.));
#48277=CARTESIAN_POINT('Origin',(15.,0.,4.));
#48278=CARTESIAN_POINT('Ctrl Pts',(16.9170033607455,1.63832650944338,4.));
#48279=CARTESIAN_POINT('Ctrl Pts',(16.4032792982694,2.23546892087832,4.04999787746244));
#48280=CARTESIAN_POINT('Ctrl Pts',(15.5859097998096,2.57572249729409,4.09999575492489));
#48281=CARTESIAN_POINT('Ctrl Pts',(14.8008208232653,2.51338129467797,4.14999363238733));
#48282=CARTESIAN_POINT('Ctrl Pts',(13.9790588101819,2.44812801296032,4.20232700817141));
#48283=CARTESIAN_POINT('Ctrl Pts',(13.1926635275253,1.94178951401471,4.2546603839555));
#48284=CARTESIAN_POINT('Ctrl Pts',(12.7937453701095,1.22068434196769,4.30699375973958));
#48285=CARTESIAN_POINT('Ctrl Pts',(12.5894005030727,0.851299951304611,4.3338014056624));
#48286=CARTESIAN_POINT('Ctrl Pts',(12.4867287035022,0.425561301199251,4.36060905158521));
#48287=CARTESIAN_POINT('Ctrl Pts',(12.4864520394788,-8.37379766882585E-5,
4.38741669750802));
#48288=CARTESIAN_POINT('Origin',(15.,0.,7.5));
#48289=CARTESIAN_POINT('',(12.4798657694311,-0.00154038945686864,5.38741669750803));
#48290=CARTESIAN_POINT('',(12.4793021139561,0.00120904389216911,5.11258330249198));
#48291=CARTESIAN_POINT('',(12.4825,3.08304831685346E-16,7.5));
#48292=CARTESIAN_POINT('Ctrl Pts',(12.4793021139561,0.00120904389216911,
5.11258330249198));
#48293=CARTESIAN_POINT('Ctrl Pts',(12.478879906904,0.0725686704440801,5.10805583214991));
#48294=CARTESIAN_POINT('Ctrl Pts',(12.4816538040259,0.14389470397244,5.10352836180784));
#48295=CARTESIAN_POINT('Ctrl Pts',(12.4877315613661,0.214937734438189,5.09900089146578));
#48296=CARTESIAN_POINT('Ctrl Pts',(12.5579848230722,1.0361295544392,5.04666751568169));
#48297=CARTESIAN_POINT('Ctrl Pts',(13.0696742764471,1.81950869898314,4.99433413989761));
#48298=CARTESIAN_POINT('Ctrl Pts',(13.7933805800141,2.21395750784665,4.94200076411352));
#48299=CARTESIAN_POINT('Ctrl Pts',(14.5170868835811,2.60840631671017,4.88966738832944));
#48300=CARTESIAN_POINT('Ctrl Pts',(15.4528100373402,2.61392478989326,4.83733401254535));
#48301=CARTESIAN_POINT('Ctrl Pts',(16.1810158838377,2.22781637405164,4.78500063676127));
#48302=CARTESIAN_POINT('Ctrl Pts',(16.9092217303351,1.84170795821001,4.73266726097718));
#48303=CARTESIAN_POINT('Ctrl Pts',(17.4299102695709,1.06397265334366,4.6803338851931));
#48304=CARTESIAN_POINT('Ctrl Pts',(17.5096246317311,0.243745210316159,4.62800050940901));
#48305=CARTESIAN_POINT('Ctrl Pts',(17.5893389938914,-0.576482232711353,
4.57566713362493));
#48306=CARTESIAN_POINT('Ctrl Pts',(17.2280791789763,-1.43920181390003,4.52333375784085));
#48307=CARTESIAN_POINT('Ctrl Pts',(16.5878264117224,-1.95845762325597,4.47100038205676));
#48308=CARTESIAN_POINT('Ctrl Pts',(15.9475736444685,-2.47771343261192,4.41866700627268));
#48309=CARTESIAN_POINT('Ctrl Pts',(15.0283279248759,-2.65350547013512,4.36633363048859));
#48310=CARTESIAN_POINT('Ctrl Pts',(14.2422049662735,-2.40531717421469,4.3140002547045));
#48311=CARTESIAN_POINT('Ctrl Pts',(13.4560820076711,-2.15712887829427,4.26166687892042));
#48312=CARTESIAN_POINT('Ctrl Pts',(12.8030818100589,-1.48496024893023,4.20933350313634));
#48313=CARTESIAN_POINT('Ctrl Pts',(12.5762083591215,-0.69397784322712,4.15700012735226));
#48314=CARTESIAN_POINT('Ctrl Pts',(12.5120237084102,-0.470201419766977,
4.1421945190655));
#48315=CARTESIAN_POINT('Ctrl Pts',(12.4819452946144,-0.236915405941376,
4.12738891077874));
#48316=CARTESIAN_POINT('Ctrl Pts',(12.4839933051997,-0.00316412607611227,
4.11258330249198));
#48317=CARTESIAN_POINT('Ctrl Pts',(12.4864520394788,-8.37379766882585E-5,
4.38741669750802));
#48318=CARTESIAN_POINT('Ctrl Pts',(12.4861886052651,-0.405374837317443,
4.41294242736929));
#48319=CARTESIAN_POINT('Ctrl Pts',(12.5787615741259,-0.810581064443052,
4.43846815723057));
#48320=CARTESIAN_POINT('Ctrl Pts',(12.7647943027407,-1.16697133984538,4.46399388709184));
#48321=CARTESIAN_POINT('Ctrl Pts',(13.146202424963,-1.897650004463,4.51632726287592));
#48322=CARTESIAN_POINT('Ctrl Pts',(13.9204597015827,-2.42313548854983,4.56866063866001));
#48323=CARTESIAN_POINT('Ctrl Pts',(14.7402998673034,-2.50800691661078,4.62099401444409));
#48324=CARTESIAN_POINT('Ctrl Pts',(15.560140033024,-2.59287834467174,4.67332739022818));
#48325=CARTESIAN_POINT('Ctrl Pts',(16.4255630878457,-2.23713571670682,4.72566076601226));
#48326=CARTESIAN_POINT('Ctrl Pts',(16.9486162247073,-1.60018404184685,4.77799414179635));
#48327=CARTESIAN_POINT('Ctrl Pts',(17.471669361569,-0.963232366986897,4.83032751758043));
#48328=CARTESIAN_POINT('Ctrl Pts',(17.6523525804706,-0.0450716452319087,
4.88266089336451));
#48329=CARTESIAN_POINT('Ctrl Pts',(17.4096229743894,0.742588180844264,4.9349942691486));
#48330=CARTESIAN_POINT('Ctrl Pts',(17.1668933683082,1.53024800692044,4.98732764493268));
#48331=CARTESIAN_POINT('Ctrl Pts',(16.5007509372442,2.1874069373178,5.03966102071677));
#48332=CARTESIAN_POINT('Ctrl Pts',(15.7098806230762,2.41944933284425,5.09199439650085));
#48333=CARTESIAN_POINT('Ctrl Pts',(14.9190103089082,2.6514917283707,5.14432777228493));
#48334=CARTESIAN_POINT('Ctrl Pts',(14.0034121116361,2.45841758902623,5.19666114806902));
#48335=CARTESIAN_POINT('Ctrl Pts',(13.3735902615222,1.92677994818613,5.2489945238531));
#48336=CARTESIAN_POINT('Ctrl Pts',(12.8182957469354,1.45805142494902,5.29513524840474));
#48337=CARTESIAN_POINT('Ctrl Pts',(12.4851467735748,0.72614376520494,5.34127597295639));
#48338=CARTESIAN_POINT('Ctrl Pts',(12.4798657694311,-0.00154038945686864,
5.38741669750803));
#48339=CARTESIAN_POINT('Origin',(15.,0.,7.5));
#48340=CARTESIAN_POINT('',(12.482920633805,0.00216662177004473,6.38741669750803));
#48341=CARTESIAN_POINT('',(12.4862854318642,0.000566909999415368,6.11258330249198));
#48342=CARTESIAN_POINT('',(12.4825,3.08304831685346E-16,7.5));
#48343=CARTESIAN_POINT('Ctrl Pts',(12.4862854318642,0.000566909999415368,
6.11258330249198));
#48344=CARTESIAN_POINT('Ctrl Pts',(12.4855058897774,0.379333771915191,6.08872275352109));
#48345=CARTESIAN_POINT('Ctrl Pts',(12.5659381445238,0.757786273313489,6.06486220455019));
#48346=CARTESIAN_POINT('Ctrl Pts',(12.7293101493446,1.09619859491376,6.04100165557929));
#48347=CARTESIAN_POINT('Ctrl Pts',(13.08763419844,1.83843881821599,5.98866827979521));
#48348=CARTESIAN_POINT('Ctrl Pts',(13.8449458114837,2.38806291012985,5.93633490401113));
#48349=CARTESIAN_POINT('Ctrl Pts',(14.6617006772638,2.49864636478707,5.88400152822704));
#48350=CARTESIAN_POINT('Ctrl Pts',(15.4784555430439,2.60922981944428,5.83166815244296));
#48351=CARTESIAN_POINT('Ctrl Pts',(16.3546536615603,2.28077263684485,5.77933477665887));
#48352=CARTESIAN_POINT('Ctrl Pts',(16.8974474362482,1.66053609593171,5.72700140087479));
#48353=CARTESIAN_POINT('Ctrl Pts',(17.4402412109362,1.04029955501857,5.6746680250907));
#48354=CARTESIAN_POINT('Ctrl Pts',(17.6496306417956,0.128283655791723,5.62233464930662));
#48355=CARTESIAN_POINT('Ctrl Pts',(17.4317349092204,-0.66659696383412,5.57000127352254));
#48356=CARTESIAN_POINT('Ctrl Pts',(17.2138391766452,-1.46147758345996,5.51766789773845));
#48357=CARTESIAN_POINT('Ctrl Pts',(16.5686582806354,-2.13922292348481,5.46533452195437));
#48358=CARTESIAN_POINT('Ctrl Pts',(15.7854622951236,-2.39597806232545,5.41300114617028));
#48359=CARTESIAN_POINT('Ctrl Pts',(15.0022663096119,-2.65273320116609,5.3606677703862));
#48360=CARTESIAN_POINT('Ctrl Pts',(14.0810552345983,-2.48849813882253,5.30833439460211));
#48361=CARTESIAN_POINT('Ctrl Pts',(13.4348582321103,-1.9768783599217,5.25600101881803));
#48362=CARTESIAN_POINT('Ctrl Pts',(12.8445650905918,-1.50951988350108,5.20819511337601));
#48363=CARTESIAN_POINT('Ctrl Pts',(12.4837602304949,-0.752282707918894,
5.160389207934));
#48364=CARTESIAN_POINT('Ctrl Pts',(12.4793021139561,0.00120904389216911,
5.11258330249198));
#48365=CARTESIAN_POINT('Ctrl Pts',(12.4798657694311,-0.00154038945686864,
5.38741669750803));
#48366=CARTESIAN_POINT('Ctrl Pts',(12.4791569938941,-0.0992045293459824,
5.39360934874047));
#48367=CARTESIAN_POINT('Ctrl Pts',(12.4843540819724,-0.196792591522919,
5.39980199997291));
#48368=CARTESIAN_POINT('Ctrl Pts',(12.4957126236098,-0.293658114991017,
5.40599465120536));
#48369=CARTESIAN_POINT('Ctrl Pts',(12.5917023387672,-1.11225739499233,5.45832802698944));
#48370=CARTESIAN_POINT('Ctrl Pts',(13.1277272720379,-1.87925481265923,5.51066140277353));
#48371=CARTESIAN_POINT('Ctrl Pts',(13.8634558058795,-2.25076673554666,5.56299477855761));
#48372=CARTESIAN_POINT('Ctrl Pts',(14.5991843397211,-2.62227865843409,5.61532815434169));
#48373=CARTESIAN_POINT('Ctrl Pts',(15.5346164741336,-2.59830508654206,5.66766153012578));
#48374=CARTESIAN_POINT('Ctrl Pts',(16.2503478880118,-2.18959297269902,5.71999490590987));
#48375=CARTESIAN_POINT('Ctrl Pts',(16.96607930189,-1.78088085885597,5.77232828169395));
#48376=CARTESIAN_POINT('Ctrl Pts',(17.4621099952338,-0.98743020306191,5.82466165747803));
#48377=CARTESIAN_POINT('Ctrl Pts',(17.5160416303984,-0.16498929182795,5.87699503326212));
#48378=CARTESIAN_POINT('Ctrl Pts',(17.5699732655631,0.657451619406004,5.9293284090462));
#48379=CARTESIAN_POINT('Ctrl Pts',(17.1818058425485,1.50888278607985,5.98166178483029));
#48380=CARTESIAN_POINT('Ctrl Pts',(16.5255763936941,2.00756141147231,6.03399516061437));
#48381=CARTESIAN_POINT('Ctrl Pts',(15.8693469448397,2.50624003686478,6.08632853639846));
#48382=CARTESIAN_POINT('Ctrl Pts',(14.9450554701454,2.65216612097585,6.13866191218254));
#48383=CARTESIAN_POINT('Ctrl Pts',(14.1671123287709,2.37991277262463,6.19099528796662));
#48384=CARTESIAN_POINT('Ctrl Pts',(13.3891691873965,2.10765942427341,6.24332866375071));
#48385=CARTESIAN_POINT('Ctrl Pts',(12.7575743793418,1.41722664345988,6.2956620395348));
#48386=CARTESIAN_POINT('Ctrl Pts',(12.5555065470498,0.618173398042358,6.34799541531888));
#48387=CARTESIAN_POINT('Ctrl Pts',(12.5047691803197,0.417538506829285,6.36113584271526));
#48388=CARTESIAN_POINT('Ctrl Pts',(12.4811120172555,0.210055467607507,6.37427627011165));
#48389=CARTESIAN_POINT('Ctrl Pts',(12.482920633805,0.00216662177004473,
6.38741669750803));
#48390=CARTESIAN_POINT('Origin',(15.,0.,7.5));
#48391=CARTESIAN_POINT('',(12.4854953774899,-0.00143787083715985,7.38741669750803));
#48392=CARTESIAN_POINT('',(12.4810882026093,-0.00198272270578489,7.11258330249199));
#48393=CARTESIAN_POINT('',(12.4825,3.08304831685346E-16,7.5));
#48394=CARTESIAN_POINT('Ctrl Pts',(12.4810882026093,-0.00198272270578489,
7.11258330249199));
#48395=CARTESIAN_POINT('Ctrl Pts',(12.4869739395021,0.680084118616307,7.06938967489226));
#48396=CARTESIAN_POINT('Ctrl Pts',(12.7744552727444,1.36652561897882,7.02619604729254));
#48397=CARTESIAN_POINT('Ctrl Pts',(13.269118044078,1.83350231786092,6.98300241969281));
#48398=CARTESIAN_POINT('Ctrl Pts',(13.8684511896637,2.39929103307328,6.93066904390873));
#48399=CARTESIAN_POINT('Ctrl Pts',(14.7719211435091,2.64291129119537,6.87833566812465));
#48400=CARTESIAN_POINT('Ctrl Pts',(15.5744528177492,2.45513481925728,6.82600229234056));
#48401=CARTESIAN_POINT('Ctrl Pts',(16.3769844919893,2.26735834731918,6.77366891655648));
#48402=CARTESIAN_POINT('Ctrl Pts',(17.0785778866242,1.64818514532091,6.72133554077239));
#48403=CARTESIAN_POINT('Ctrl Pts',(17.3646702383797,0.875224413728682,6.66900216498831));
#48404=CARTESIAN_POINT('Ctrl Pts',(17.6507625901351,0.102263682136454,6.61666878920422));
#48405=CARTESIAN_POINT('Ctrl Pts',(17.5213538990113,-0.82448457904973,6.56433541342014));
#48406=CARTESIAN_POINT('Ctrl Pts',(17.0344651712476,-1.48950819606356,6.51200203763606));
#48407=CARTESIAN_POINT('Ctrl Pts',(16.547576443484,-2.15453181307739,6.45966866185197));
#48408=CARTESIAN_POINT('Ctrl Pts',(15.7032076790805,-2.55783078591888,6.40733528606789));
#48409=CARTESIAN_POINT('Ctrl Pts',(14.8799356660918,-2.51858436884117,6.3550019102838));
#48410=CARTESIAN_POINT('Ctrl Pts',(14.0566636531032,-2.47933795176346,6.30266853449972));
#48411=CARTESIAN_POINT('Ctrl Pts',(13.2544883915292,-1.99754614476656,6.25033515871564));
#48412=CARTESIAN_POINT('Ctrl Pts',(12.8330690033158,-1.28922206392281,6.19800178293155));
#48413=CARTESIAN_POINT('Ctrl Pts',(12.6037889105156,-0.903846792801687,
6.16952895611836));
#48414=CARTESIAN_POINT('Ctrl Pts',(12.4872156605381,-0.451416121701059,
6.14105612930517));
#48415=CARTESIAN_POINT('Ctrl Pts',(12.4862854318642,0.000566909999415368,
6.11258330249198));
#48416=CARTESIAN_POINT('Ctrl Pts',(12.482920633805,0.00216662177004473,
6.38741669750803));
#48417=CARTESIAN_POINT('Ctrl Pts',(12.488315056143,-0.617887548426095,6.42660964589573));
#48418=CARTESIAN_POINT('Ctrl Pts',(12.7202541571503,-1.24155179185567,6.46580259428343));
#48419=CARTESIAN_POINT('Ctrl Pts',(13.1359015380453,-1.69788793113621,6.50499554267113));
#48420=CARTESIAN_POINT('Ctrl Pts',(13.6909052178623,-2.30722230487577,6.55732891845522));
#48421=CARTESIAN_POINT('Ctrl Pts',(14.5734534340258,-2.61821734233337,6.6096622942393));
#48422=CARTESIAN_POINT('Ctrl Pts',(15.3878514816524,-2.49143689543374,6.66199567002338));
#48423=CARTESIAN_POINT('Ctrl Pts',(16.2022495292791,-2.36465644853411,6.71432904580747));
#48424=CARTESIAN_POINT('Ctrl Pts',(16.9484974083689,-1.80010051727723,6.76666242159155));
#48425=CARTESIAN_POINT('Ctrl Pts',(17.2920112918525,-1.05089047753226,6.81899579737564));
#48426=CARTESIAN_POINT('Ctrl Pts',(17.635525175336,-0.301680437787271,6.87132917315973));
#48427=CARTESIAN_POINT('Ctrl Pts',(17.5763050632133,0.632183710445827,6.92366254894381));
#48428=CARTESIAN_POINT('Ctrl Pts',(17.1409025824082,1.33199950499447,6.97599592472789));
#48429=CARTESIAN_POINT('Ctrl Pts',(16.7055001016032,2.03181529954311,7.02832930051198));
#48430=CARTESIAN_POINT('Ctrl Pts',(15.8939152521159,2.49758274040729,7.08066267629606));
#48431=CARTESIAN_POINT('Ctrl Pts',(15.0700259913432,2.52047275706227,7.13299605208015));
#48432=CARTESIAN_POINT('Ctrl Pts',(14.2461367305706,2.54336277371724,7.18532942786423));
#48433=CARTESIAN_POINT('Ctrl Pts',(13.4099430585124,2.12337536616301,7.23766280364831));
#48434=CARTESIAN_POINT('Ctrl Pts',(12.9363564205467,1.44881390534349,7.2899961794324));
#48435=CARTESIAN_POINT('Ctrl Pts',(12.6424900625863,1.03024018763275,7.32246968545761));
#48436=CARTESIAN_POINT('Ctrl Pts',(12.4882403133338,0.513646402355209,7.35494319148282));
#48437=CARTESIAN_POINT('Ctrl Pts',(12.4854953774899,-0.00143787083715985,
7.38741669750803));
#48438=CARTESIAN_POINT('Origin',(15.,0.,7.5));
#48439=CARTESIAN_POINT('',(12.4785663033905,-0.000147683907944251,8.38741669750803));
#48440=CARTESIAN_POINT('',(12.4815651121962,0.00207920831391662,8.11258330249198));
#48441=CARTESIAN_POINT('',(12.4825,3.08304831685346E-16,7.5));
#48442=CARTESIAN_POINT('Ctrl Pts',(12.4815651121962,0.00207920831391661,
8.11258330249198));
#48443=CARTESIAN_POINT('Ctrl Pts',(12.4801423769425,0.163120151964822,8.10238997204752));
#48444=CARTESIAN_POINT('Ctrl Pts',(12.4942993050251,0.323912101526709,8.09219664160305));
#48445=CARTESIAN_POINT('Ctrl Pts',(12.524955296352,0.48149432911561,8.08200331115859));
#48446=CARTESIAN_POINT('Ctrl Pts',(12.6823456137647,1.29053412020584,8.0296699353745));
#48447=CARTESIAN_POINT('Ctrl Pts',(13.27463109749,2.01496955827445,7.97733655959042));
#48448=CARTESIAN_POINT('Ctrl Pts',(14.036257709891,2.32999653926404,7.92500318380634));
#48449=CARTESIAN_POINT('Ctrl Pts',(14.797884322292,2.64502352025364,7.87266980802225));
#48450=CARTESIAN_POINT('Ctrl Pts',(15.7288520633688,2.55064204416424,7.82033643223817));
#48451=CARTESIAN_POINT('Ctrl Pts',(16.4117570807264,2.08916849927148,7.76800305645408));
#48452=CARTESIAN_POINT('Ctrl Pts',(17.0946620980841,1.62769495437873,7.71566968067));
#48453=CARTESIAN_POINT('Ctrl Pts',(17.5295043917226,0.799129340682624,7.66333630488591));
#48454=CARTESIAN_POINT('Ctrl Pts',(17.5213203334702,-0.0250369758568184,
7.61100292910183));
#48455=CARTESIAN_POINT('Ctrl Pts',(17.5131362752179,-0.849203292396252,
7.55866955331774));
#48456=CARTESIAN_POINT('Ctrl Pts',(17.0619258650746,-1.66897031177902,7.50633617753366));
#48457=CARTESIAN_POINT('Ctrl Pts',(16.3699914547578,-2.11679155594354,7.45400280174958));
#48458=CARTESIAN_POINT('Ctrl Pts',(15.678057044441,-2.56461280010805,7.4016694259655));
#48459=CARTESIAN_POINT('Ctrl Pts',(14.7453986339507,-2.6404882690543,7.34933605018141));
#48460=CARTESIAN_POINT('Ctrl Pts',(13.9901780954356,-2.31039883752012,7.29700267439732));
#48461=CARTESIAN_POINT('Ctrl Pts',(13.2349575569204,-1.98030940598595,7.24466929861324));
#48462=CARTESIAN_POINT('Ctrl Pts',(12.6571748903804,-1.24425507397135,7.19233592282916));
#48463=CARTESIAN_POINT('Ctrl Pts',(12.5158817257734,-0.43224932181273,7.14000254704507));
#48464=CARTESIAN_POINT('Ctrl Pts',(12.4912056194582,-0.29043679801142,7.13086279886071));
#48465=CARTESIAN_POINT('Ctrl Pts',(12.4798427838735,-0.146307696573625,
7.12172305067635));
#48466=CARTESIAN_POINT('Ctrl Pts',(12.4810882026093,-0.00198272270578489,
7.11258330249199));
#48467=CARTESIAN_POINT('Ctrl Pts',(12.4854953774899,-0.00143787083715985,
7.38741669750803));
#48468=CARTESIAN_POINT('Ctrl Pts',(12.4838166530455,-0.316448716062932,
7.4072765672669));
#48469=CARTESIAN_POINT('Ctrl Pts',(12.5388037075173,-0.630894974090679,
7.42713643702578));
#48470=CARTESIAN_POINT('Ctrl Pts',(12.6531758459131,-0.922010273445696,
7.44699630678465));
#48471=CARTESIAN_POINT('Ctrl Pts',(12.9545615131189,-1.68913747733048,7.49932968256874));
#48472=CARTESIAN_POINT('Ctrl Pts',(13.6683124514037,-2.29425637101525,7.55166305835282));
#48473=CARTESIAN_POINT('Ctrl Pts',(14.474415004267,-2.46605899527454,7.6039964341369));
#48474=CARTESIAN_POINT('Ctrl Pts',(15.2805175571303,-2.63786161953383,7.65632980992099));
#48475=CARTESIAN_POINT('Ctrl Pts',(16.1789717245721,-2.37634797436764,7.70866318570507));
#48476=CARTESIAN_POINT('Ctrl Pts',(16.766951270731,-1.79876895739606,7.76099656148916));
#48477=CARTESIAN_POINT('Ctrl Pts',(17.35493081689,-1.22118994042448,7.81332993727324));
#48478=CARTESIAN_POINT('Ctrl Pts',(17.6324357417662,-0.327545551647488,
7.86566331305733));
#48479=CARTESIAN_POINT('Ctrl Pts',(17.4750453812635,0.48149446094025,7.91799668884141));
#48480=CARTESIAN_POINT('Ctrl Pts',(17.3176550207607,1.290534473528,7.97033006462549));
#48481=CARTESIAN_POINT('Ctrl Pts',(16.7253693748791,2.01497010992651,8.02266344040958));
#48482=CARTESIAN_POINT('Ctrl Pts',(15.9637425539609,2.32999717716545,8.07499681619367));
#48483=CARTESIAN_POINT('Ctrl Pts',(15.2021157330427,2.64502424440439,8.12733019197775));
#48484=CARTESIAN_POINT('Ctrl Pts',(14.271147737088,2.55064274248376,8.17966356776183));
#48485=CARTESIAN_POINT('Ctrl Pts',(13.5882425327649,2.08916907124602,8.23199694354592));
#48486=CARTESIAN_POINT('Ctrl Pts',(12.9122114961964,1.63234062369425,8.28380352819995));
#48487=CARTESIAN_POINT('Ctrl Pts',(12.4792743543203,0.815773157793952,8.33561011285399));
#48488=CARTESIAN_POINT('Ctrl Pts',(12.4785663033905,-0.000147683907944251,
8.38741669750803));
#48489=CARTESIAN_POINT('Origin',(15.,0.,7.5));
#48490=CARTESIAN_POINT('',(12.4851788739807,0.00162480267774629,9.38741669750802));
#48491=CARTESIAN_POINT('',(12.486145438329,-0.000815058042068406,9.11258330249198));
#48492=CARTESIAN_POINT('',(12.4825,3.08304831685346E-16,7.5));
#48493=CARTESIAN_POINT('Ctrl Pts',(12.486145438329,-0.000815058042068406,
9.11258330249198));
#48494=CARTESIAN_POINT('Ctrl Pts',(12.4875376300823,0.467827170949961,9.08305689341869));
#48495=CARTESIAN_POINT('Ctrl Pts',(12.6134446697461,0.937164267550756,9.0535304843454));
#48496=CARTESIAN_POINT('Ctrl Pts',(12.8590980037376,1.33199914029708,9.02400407527211));
#48497=CARTESIAN_POINT('Ctrl Pts',(13.2945003653482,2.03181474323085,8.97167069948803));
#48498=CARTESIAN_POINT('Ctrl Pts',(14.1060849926179,2.49758205662421,8.91933732370394));
#48499=CARTESIAN_POINT('Ctrl Pts',(14.9299740278219,2.52047206702312,8.86700394791986));
#48500=CARTESIAN_POINT('Ctrl Pts',(15.753863063026,2.54336207742203,8.81467057213577));
#48501=CARTESIAN_POINT('Ctrl Pts',(16.5900565061644,2.12337478482649,8.76233719635169));
#48502=CARTESIAN_POINT('Ctrl Pts',(17.063643014475,1.44881350868189,8.7100038205676));
#48503=CARTESIAN_POINT('Ctrl Pts',(17.5372295227856,0.774252232537298,8.65767044478352));
#48504=CARTESIAN_POINT('Ctrl Pts',(17.6482090962684,-0.154883027156347,
8.60533706899943));
#48505=CARTESIAN_POINT('Ctrl Pts',(17.3468235115742,-0.922010021015011,
8.55300369321535));
#48506=CARTESIAN_POINT('Ctrl Pts',(17.0454379268799,-1.68913701487367,8.50067031743127));
#48507=CARTESIAN_POINT('Ctrl Pts',(16.3316871840086,-2.29425574289735,8.44833694164718));
#48508=CARTESIAN_POINT('Ctrl Pts',(15.5255848518399,-2.46605832012208,8.3960035658631));
#48509=CARTESIAN_POINT('Ctrl Pts',(14.7194825196712,-2.6378608973468,8.34367019007902));
#48510=CARTESIAN_POINT('Ctrl Pts',(13.8210285982051,-2.37634732377256,8.29133681429493));
#48511=CARTESIAN_POINT('Ctrl Pts',(13.2330492130222,-1.79876846492951,8.23900343851085));
#48512=CARTESIAN_POINT('Ctrl Pts',(12.7595946043877,-1.33368860080475,8.19686339317123));
#48513=CARTESIAN_POINT('Ctrl Pts',(12.4874468138073,-0.663676964701131,
8.1547233478316));
#48514=CARTESIAN_POINT('Ctrl Pts',(12.4815651121962,0.00207920831391661,
8.11258330249198));
#48515=CARTESIAN_POINT('Ctrl Pts',(12.4785663033905,-0.000147683907944251,
8.38741669750803));
#48516=CARTESIAN_POINT('Ctrl Pts',(12.478559103631,-0.0084443100048087,
8.38794348863808));
#48517=CARTESIAN_POINT('Ctrl Pts',(12.4785965949646,-0.016740869242818,
8.38847027976812));
#48518=CARTESIAN_POINT('Ctrl Pts',(12.4786789762444,-0.0250369827190495,
8.38899707089817));
#48519=CARTESIAN_POINT('Ctrl Pts',(12.4868630367383,-0.84920352489154,8.44133044668226));
#48520=CARTESIAN_POINT('Ctrl Pts',(12.9380735704173,-1.66897076868167,8.49366382246634));
#48521=CARTESIAN_POINT('Ctrl Pts',(13.6300081701693,-2.11679213546203,8.54599719825043));
#48522=CARTESIAN_POINT('Ctrl Pts',(14.3219427699214,-2.5646135022424,8.59833057403451));
#48523=CARTESIAN_POINT('Ctrl Pts',(15.2546014357464,-2.64048899201301,8.65066394981859));
#48524=CARTESIAN_POINT('Ctrl Pts',(16.0098221810285,-2.31039947008532,8.70299732560268));
#48525=CARTESIAN_POINT('Ctrl Pts',(16.7650429263106,-1.98030994815763,8.75533070138676));
#48526=CARTESIAN_POINT('Ctrl Pts',(17.3428257510498,-1.24425541453165,8.80766407717086));
#48527=CARTESIAN_POINT('Ctrl Pts',(17.4841189543331,-0.432249440103775,
8.85999745295494));
#48528=CARTESIAN_POINT('Ctrl Pts',(17.6254121576165,0.379756534324098,8.91233082873902));
#48529=CARTESIAN_POINT('Ctrl Pts',(17.3302157394439,1.26771394955386,8.9646642045231));
#48530=CARTESIAN_POINT('Ctrl Pts',(16.7308824297867,1.83350281974262,9.01699758030718));
#48531=CARTESIAN_POINT('Ctrl Pts',(16.1315491201295,2.39929168993138,9.06933095609127));
#48532=CARTESIAN_POINT('Ctrl Pts',(15.2280789189876,2.64291201507916,9.12166433187536));
#48533=CARTESIAN_POINT('Ctrl Pts',(14.4255470250055,2.45513549159302,9.17399770765945));
#48534=CARTESIAN_POINT('Ctrl Pts',(13.6230151310234,2.26735896810689,9.22633108344353));
#48535=CARTESIAN_POINT('Ctrl Pts',(12.9214215442012,1.64818559598687,9.2786644592276));
#48536=CARTESIAN_POINT('Ctrl Pts',(12.6353291141696,0.875224653029136,9.33099783501169));
#48537=CARTESIAN_POINT('Ctrl Pts',(12.5325202200407,0.597456870981902,9.34980412251047));
#48538=CARTESIAN_POINT('Ctrl Pts',(12.4833676454127,0.29982951718309,9.36861041000924));
#48539=CARTESIAN_POINT('Ctrl Pts',(12.4851788739807,0.00162480267774629,
9.38741669750802));
#48540=CARTESIAN_POINT('Origin',(15.,0.,7.5));
#48541=CARTESIAN_POINT('',(12.4833920687165,-0.00213593309729046,10.387416697508));
#48542=CARTESIAN_POINT('',(12.4790122776664,-0.000936909191352325,10.112583302492));
#48543=CARTESIAN_POINT('',(12.4825,3.08304831685346E-16,7.5));
#48544=CARTESIAN_POINT('Ctrl Pts',(12.4790122776664,-0.000936909191352325,
10.112583302492));
#48545=CARTESIAN_POINT('Ctrl Pts',(12.4827416706421,0.768933033990792,10.0637238147899));
#48546=CARTESIAN_POINT('Ctrl Pts',(12.8617552362247,1.54198463745441,10.0148643270877));
#48547=CARTESIAN_POINT('Ctrl Pts',(13.4744240244193,2.00756086084053,9.96600483938563));
#48548=CARTESIAN_POINT('Ctrl Pts',(14.1306532939369,2.50623934889895,9.91367146360154));
#48549=CARTESIAN_POINT('Ctrl Pts',(15.0549445147503,2.65216539497217,9.86133808781746));
#48550=CARTESIAN_POINT('Ctrl Pts',(15.8328874429565,2.37991212159725,9.80900471203338));
#48551=CARTESIAN_POINT('Ctrl Pts',(16.6108303711627,2.10765884822232,9.75667133624929));
#48552=CARTESIAN_POINT('Ctrl Pts',(17.2424250067619,1.41722625539925,9.70433796046521));
#48553=CARTESIAN_POINT('Ctrl Pts',(17.4444927838351,0.618173228507267,9.65200458468112));
#48554=CARTESIAN_POINT('Ctrl Pts',(17.6465605609084,-0.18087979838472,9.59967120889704));
#48555=CARTESIAN_POINT('Ctrl Pts',(17.4191014794558,-1.08855325934562,9.54733783311295));
#48556=CARTESIAN_POINT('Ctrl Pts',(16.8640979515296,-1.69788746613335,9.49500445732887));
#48557=CARTESIAN_POINT('Ctrl Pts',(16.3090944236034,-2.30722167292107,9.44267108154478));
#48558=CARTESIAN_POINT('Ctrl Pts',(15.4265464492036,-2.61821662553562,9.3903377057607));
#48559=CARTESIAN_POINT('Ctrl Pts',(14.6121486245737,-2.49143621341537,9.33800432997662));
#48560=CARTESIAN_POINT('Ctrl Pts',(13.7977507999438,-2.36465580129513,9.28567095419253));
#48561=CARTESIAN_POINT('Ctrl Pts',(13.0515031250838,-1.80010002444009,9.23333757840845));
#48562=CARTESIAN_POINT('Ctrl Pts',(12.7079893356296,-1.05089018977548,9.18100420262436));
#48563=CARTESIAN_POINT('Ctrl Pts',(12.5582854909339,-0.724383376435316,
9.15819723591357));
#48564=CARTESIAN_POINT('Ctrl Pts',(12.4850700731909,-0.362806510824638,
9.13539026920278));
#48565=CARTESIAN_POINT('Ctrl Pts',(12.486145438329,-0.000815058042068406,
9.11258330249198));
#48566=CARTESIAN_POINT('Ctrl Pts',(12.4851788739807,0.00162480267774629,
9.38741669750802));
#48567=CARTESIAN_POINT('Ctrl Pts',(12.4884078589736,-0.530002494361348,
9.42094378579333));
#48568=CARTESIAN_POINT('Ctrl Pts',(12.6536116109961,-1.06346477741145,9.45447087407864));
#48569=CARTESIAN_POINT('Ctrl Pts',(12.9655342718635,-1.48950860327335,9.48799796236395));
#48570=CARTESIAN_POINT('Ctrl Pts',(13.4524231328298,-2.15453240282264,9.54033133814804));
#48571=CARTESIAN_POINT('Ctrl Pts',(14.2967921280032,-2.55783148812579,9.59266471393212));
#48572=CARTESIAN_POINT('Ctrl Pts',(15.1200643665754,-2.51858505945467,9.6449980897162));
#48573=CARTESIAN_POINT('Ctrl Pts',(15.9433366051476,-2.47933863078355,9.69733146550028));
#48574=CARTESIAN_POINT('Ctrl Pts',(16.7455120871185,-1.99754668813814,9.74966484128436));
#48575=CARTESIAN_POINT('Ctrl Pts',(17.1669315903404,-1.28922241490791,9.80199821706845));
#48576=CARTESIAN_POINT('Ctrl Pts',(17.5883510935622,-0.580898141677671,
9.85433159285254));
#48577=CARTESIAN_POINT('Ctrl Pts',(17.6290146180349,0.353958462137397,9.90666496863663));
#48578=CARTESIAN_POINT('Ctrl Pts',(17.2706904715522,1.09619889141998,9.95899834442071));
#48579=CARTESIAN_POINT('Ctrl Pts',(16.9123663250695,1.83843932070257,10.0113317202048));
#48580=CARTESIAN_POINT('Ctrl Pts',(16.1550545076315,2.38806357545267,10.0636650959889));
#48581=CARTESIAN_POINT('Ctrl Pts',(15.3382994168527,2.49864705542611,10.115998471773));
#48582=CARTESIAN_POINT('Ctrl Pts',(14.5215443260739,2.60923053539955,10.168331847557));
#48583=CARTESIAN_POINT('Ctrl Pts',(13.6453459619542,2.28077324059635,10.2206652233411));
#48584=CARTESIAN_POINT('Ctrl Pts',(13.1025520413601,1.66053653868267,10.2729985991252));
#48585=CARTESIAN_POINT('Ctrl Pts',(12.7069762589991,1.20852223030592,10.3111379652528));
#48586=CARTESIAN_POINT('Ctrl Pts',(12.4884769342622,0.601539190041919,10.3492773313804));
#48587=CARTESIAN_POINT('Ctrl Pts',(12.4833920687165,-0.00213593309729046,
10.387416697508));
#48588=CARTESIAN_POINT('Origin',(15.,0.,7.5));
#48589=CARTESIAN_POINT('',(12.4794948718273,0.00124609658704006,11.387416697508));
#48590=CARTESIAN_POINT('',(12.4841021658346,0.00201143405015815,11.112583302492));
#48591=CARTESIAN_POINT('',(12.4825,3.08304831685346E-16,7.5));
#48592=CARTESIAN_POINT('',(16.9134659966651,1.63598720337492,12.));
#48593=CARTESIAN_POINT('Ctrl Pts',(12.4794948718273,0.00124609658704006,
11.387416697508));
#48594=CARTESIAN_POINT('Ctrl Pts',(12.4843009282632,-0.742606326482963,
11.4346110043198));
#48595=CARTESIAN_POINT('Ctrl Pts',(12.8347911135691,-1.49019380442116,11.4818053111315));
#48596=CARTESIAN_POINT('Ctrl Pts',(13.4121725655462,-1.95845906653105,11.5289996179432));
#48597=CARTESIAN_POINT('Ctrl Pts',(14.0524260736147,-2.47771453576351,11.5813329937273));
#48598=CARTESIAN_POINT('Ctrl Pts',(14.971674348053,-2.65350400257885,11.6336663695114));
#48599=CARTESIAN_POINT('Ctrl Pts',(15.7577964008607,-2.4053165320775,11.6859997452955));
#48600=CARTESIAN_POINT('Ctrl Pts',(16.5439184536685,-2.15712906157615,11.7383331210796));
#48601=CARTESIAN_POINT('Ctrl Pts',(17.1969142848456,-1.4849646537581,11.7906664968637));
#48602=CARTESIAN_POINT('Ctrl Pts',(17.4237876204482,-0.693982202234524,
11.8429998726477));
#48603=CARTESIAN_POINT('Ctrl Pts',(17.6506609560507,0.0970002492890512,
11.8953332484318));
#48604=CARTESIAN_POINT('Ctrl Pts',(17.4514117960785,1.00680074451815,11.9476666242159));
#48605=CARTESIAN_POINT('Ctrl Pts',(16.9134659966651,1.63598720337493,12.));
#48606=CARTESIAN_POINT('',(13.0830107080184,1.63831915944298,12.));
#48607=CARTESIAN_POINT('Origin',(15.,0.,12.));
#48608=CARTESIAN_POINT('Ctrl Pts',(13.0829974340784,1.63832794503776,12.));
#48609=CARTESIAN_POINT('Ctrl Pts',(13.5967216860793,2.23547110522819,11.9500021225376));
#48610=CARTESIAN_POINT('Ctrl Pts',(14.4140905740858,2.57572139725963,11.9000042450751));
#48611=CARTESIAN_POINT('Ctrl Pts',(15.1991791514308,2.51337952595466,11.8500063676127));
#48612=CARTESIAN_POINT('Ctrl Pts',(16.0209407466675,2.44812554431239,11.7976729918286));
#48613=CARTESIAN_POINT('Ctrl Pts',(16.8073358429282,1.94178921121356,11.7453396160445));
#48614=CARTESIAN_POINT('Ctrl Pts',(17.2062539503585,1.22068465472099,11.6930062402604));
#48615=CARTESIAN_POINT('Ctrl Pts',(17.6051720577887,0.499580098228415,11.6406728644763));
#48616=CARTESIAN_POINT('Ctrl Pts',(17.6166131763885,-0.436292681657898,
11.5883394886922));
#48617=CARTESIAN_POINT('Ctrl Pts',(17.2352051529428,-1.16697139580525,11.5360061129082));
#48618=CARTESIAN_POINT('Ctrl Pts',(16.853797129497,-1.8976501099526,11.4836727371241));
#48619=CARTESIAN_POINT('Ctrl Pts',(16.0795399640059,-2.42313475836099,11.43133936134));
#48620=CARTESIAN_POINT('Ctrl Pts',(15.259700012361,-2.508006015706,11.3790059855559));
#48621=CARTESIAN_POINT('Ctrl Pts',(14.439860060716,-2.59287727305101,11.3266726097718));
#48622=CARTESIAN_POINT('Ctrl Pts',(13.5744373229174,-2.23713513933264,11.2743392339877));
#48623=CARTESIAN_POINT('Ctrl Pts',(13.0513843414681,-1.60018372469102,11.2220058582037));
#48624=CARTESIAN_POINT('Ctrl Pts',(12.6868381785572,-1.15625509336019,11.1855316729664));
#48625=CARTESIAN_POINT('Ctrl Pts',(12.488598465426,-0.575728774038117,11.1490574877292));
#48626=CARTESIAN_POINT('Ctrl Pts',(12.4841021658346,0.00201143405015815,
11.112583302492));
#48627=CARTESIAN_POINT('Origin',(15.,0.,14.2084234471775));
#48628=CARTESIAN_POINT('',(11.9225958479619,0.00147606609843115,4.79157655282255));
#48629=CARTESIAN_POINT('',(11.9313248632922,-0.000102231845577353,4.70842344717745));
#48630=CARTESIAN_POINT('',(11.9265,6.70613782525944E-14,14.2084234471775));
#48631=CARTESIAN_POINT('',(15.7937992825329,-2.9692229537457,4.));
#48632=CARTESIAN_POINT('Ctrl Pts',(11.9313248632922,-0.000102231845577234,
4.70842344717745));
#48633=CARTESIAN_POINT('Ctrl Pts',(11.9316626296779,0.519548226111607,4.68161580125464));
#48634=CARTESIAN_POINT('Ctrl Pts',(12.3017104806267,2.0539878015009,4.60247477954774));
#48635=CARTESIAN_POINT('Ctrl Pts',(14.713653685934,3.60697232347283,4.47100038205677));
#48636=CARTESIAN_POINT('Ctrl Pts',(17.8529409071999,2.23046453345384,4.3140002547045));
#48637=CARTESIAN_POINT('Ctrl Pts',(18.4294036968932,-1.15306868324745,4.15700012735226));
#48638=CARTESIAN_POINT('Ctrl Pts',(16.7701400584231,-2.7082056372685,4.05233337578409));
#48639=CARTESIAN_POINT('Ctrl Pts',(15.7937992825329,-2.9692229537457,4.));
#48640=CARTESIAN_POINT('',(14.2042685477155,-2.9740056618826,4.));
#48641=CARTESIAN_POINT('Origin',(15.,0.,4.));
#48642=CARTESIAN_POINT('Ctrl Pts',(11.9225958479619,0.00147606609843164,
4.79157655282255));
#48643=CARTESIAN_POINT('Ctrl Pts',(11.9220803947843,0.0885957531718082,
4.78704908248048));
#48644=CARTESIAN_POINT('Ctrl Pts',(11.9646120017673,1.18222348786824,4.73018823635433));
#48645=CARTESIAN_POINT('Ctrl Pts',(13.2680522040149,3.17774609218688,4.62099401444409));
#48646=CARTESIAN_POINT('Ctrl Pts',(16.6951963308219,3.19795784272698,4.46399388709183));
#48647=CARTESIAN_POINT('Ctrl Pts',(18.6022504225887,0.349454018091392,4.30699375973959));
#48648=CARTESIAN_POINT('Ctrl Pts',(17.2987966073653,-2.76330605967289,4.15232913070897));
#48649=CARTESIAN_POINT('Ctrl Pts',(15.1340732479013,-3.21955219912907,4.04999787746244));
#48650=CARTESIAN_POINT('Ctrl Pts',(14.2042612683071,-2.97402368063355,4.));
#48651=CARTESIAN_POINT('Origin',(15.,0.,14.2084234471775));
#48652=CARTESIAN_POINT('',(11.9311214597158,0.000692114352876805,5.79157655282255));
#48653=CARTESIAN_POINT('',(11.9232839890155,-0.001880590663607,5.70842344717745));
#48654=CARTESIAN_POINT('',(11.9265,6.70613782525944E-14,14.2084234471775));
#48655=CARTESIAN_POINT('Ctrl Pts',(11.9232839890155,-0.00188059066360697,
5.70842344717745));
#48656=CARTESIAN_POINT('Ctrl Pts',(11.9297313241637,0.88651553618964,5.66228272262581));
#48657=CARTESIAN_POINT('Ctrl Pts',(12.7977715060129,2.79354605065376,5.56380862229009));
#48658=CARTESIAN_POINT('Ctrl Pts',(16.0189351514379,3.47279968000896,5.41300114617029));
#48659=CARTESIAN_POINT('Ctrl Pts',(18.4587231497003,1.06591431050395,5.25600101881802));
#48660=CARTESIAN_POINT('Ctrl Pts',(17.7969596462713,-2.29690631906584,5.09900089146578));
#48661=CARTESIAN_POINT('Ctrl Pts',(14.6272939950368,-3.59983577334609,4.94200076411352));
#48662=CARTESIAN_POINT('Ctrl Pts',(12.2757333222409,-2.00384044231271,4.81180828268409));
#48663=CARTESIAN_POINT('Ctrl Pts',(11.9310032485729,-0.494903500494573,
4.73394917703873));
#48664=CARTESIAN_POINT('Ctrl Pts',(11.9313248632922,-0.000102231845577234,
4.70842344717745));
#48665=CARTESIAN_POINT('Ctrl Pts',(11.9311214597158,0.000692114352877186,
5.79157655282255));
#48666=CARTESIAN_POINT('Ctrl Pts',(11.930169752624,0.463111161065124,5.76771600385165));
#48667=CARTESIAN_POINT('Ctrl Pts',(12.2437393113606,1.9385290048203,5.69152207909668));
#48668=CARTESIAN_POINT('Ctrl Pts',(14.5144143770745,3.58648699137295,5.56299477855761));
#48669=CARTESIAN_POINT('Ctrl Pts',(17.7235443678513,2.3834921742297,5.40599465120536));
#48670=CARTESIAN_POINT('Ctrl Pts',(18.4904461542425,-0.956822661448993,
5.2489945238531));
#48671=CARTESIAN_POINT('Ctrl Pts',(16.1274310791049,-3.43910703392132,5.09199439650085));
#48672=CARTESIAN_POINT('Ctrl Pts',(12.8507354093227,-2.85493220992714,4.93952173949066));
#48673=CARTESIAN_POINT('Ctrl Pts',(11.9280385574681,-0.918427369528735,
4.83938245826456));
#48674=CARTESIAN_POINT('Ctrl Pts',(11.9225958479619,0.00147606609843164,
4.79157655282255));
#48675=CARTESIAN_POINT('Origin',(15.,0.,14.2084234471775));
#48676=CARTESIAN_POINT('',(11.9247764014775,-0.00242061498952145,6.79157655282255));
#48677=CARTESIAN_POINT('',(11.9270135324726,0.00264512890178066,6.70842344717746));
#48678=CARTESIAN_POINT('',(11.9265,6.70613782525944E-14,14.2084234471775));
#48679=CARTESIAN_POINT('Ctrl Pts',(11.9270135324726,0.00264512890178106,
6.70842344717746));
#48680=CARTESIAN_POINT('Ctrl Pts',(11.9248054756842,0.256447062439599,6.69528301978107));
#48681=CARTESIAN_POINT('Ctrl Pts',(12.0687133238052,1.518578012587,6.62980921660061));
#48682=CARTESIAN_POINT('Ctrl Pts',(13.8044957855091,3.41606212207931,6.51200203763605));
#48683=CARTESIAN_POINT('Ctrl Pts',(17.1897706782275,2.88159878204111,6.35500191028381));
#48684=CARTESIAN_POINT('Ctrl Pts',(18.6114579568395,-0.236820710438023,
6.19800178293155));
#48685=CARTESIAN_POINT('Ctrl Pts',(16.7947147560542,-3.14288298322814,6.04100165557929));
#48686=CARTESIAN_POINT('Ctrl Pts',(13.3686365056666,-3.23068767821543,5.88400152822705));
#48687=CARTESIAN_POINT('Ctrl Pts',(11.9823834565481,-1.24709989542488,5.77314212542643));
#48688=CARTESIAN_POINT('Ctrl Pts',(11.9224186775506,-0.121114248637474,
5.7146160984099));
#48689=CARTESIAN_POINT('Ctrl Pts',(11.9232839890155,-0.00188059066360697,
5.70842344717745));
#48690=CARTESIAN_POINT('Ctrl Pts',(11.9247764014775,-0.00242061498952133,
6.79157655282255));
#48691=CARTESIAN_POINT('Ctrl Pts',(11.9319620270346,0.830283431407061,6.74838292522283));
#48692=CARTESIAN_POINT('Ctrl Pts',(12.7081731527432,2.68370300380156,6.65285592183902));
#48693=CARTESIAN_POINT('Ctrl Pts',(15.824553937525,3.52403365117268,6.50499554267113));
#48694=CARTESIAN_POINT('Ctrl Pts',(18.3941832901488,1.25627336953411,6.34799541531888));
#48695=CARTESIAN_POINT('Ctrl Pts',(17.9202159270872,-2.13799965619268,6.19099528796662));
#48696=CARTESIAN_POINT('Ctrl Pts',(14.8276629212552,-3.61510717519363,6.03399516061437));
#48697=CARTESIAN_POINT('Ctrl Pts',(12.3361598311427,-2.11869381838128,5.90085558223301));
#48698=CARTESIAN_POINT('Ctrl Pts',(11.9322571331336,-0.551113187705301,
5.82004937963574));
#48699=CARTESIAN_POINT('Ctrl Pts',(11.9311214597158,0.000692114352877186,
5.79157655282255));
#48700=CARTESIAN_POINT('Origin',(15.,0.,14.2084234471775));
#48701=CARTESIAN_POINT('',(11.9253586384648,0.00253840983232584,7.79157655282255));
#48702=CARTESIAN_POINT('',(11.9301569186554,-0.00175543039446494,7.70842344717746));
#48703=CARTESIAN_POINT('',(11.9265,6.70613782525944E-14,14.2084234471775));
#48704=CARTESIAN_POINT('Ctrl Pts',(11.9301569186554,-0.00175543039446478,
7.70842344717746));
#48705=CARTESIAN_POINT('Ctrl Pts',(11.9335080846202,0.627087276122613,7.67594994115225));
#48706=CARTESIAN_POINT('Ctrl Pts',(12.425309891706,2.27416779560488,7.59114305934296));
#48707=CARTESIAN_POINT('Ctrl Pts',(15.1005134031695,3.61781798694653,7.45400280174957));
#48708=CARTESIAN_POINT('Ctrl Pts',(18.0729932858696,1.91191582667314,7.29700267439733));
#48709=CARTESIAN_POINT('Ctrl Pts',(18.2898906220475,-1.50841957701434,7.14000254704506));
#48710=CARTESIAN_POINT('Ctrl Pts',(15.5567114486024,-3.57614071471203,6.98300241969282));
#48711=CARTESIAN_POINT('Ctrl Pts',(12.5948647250275,-2.532436114927,6.83914271973694));
#48712=CARTESIAN_POINT('Ctrl Pts',(11.9335993346794,-0.754350498545223,
6.74761639556516));
#48713=CARTESIAN_POINT('Ctrl Pts',(11.9270135324726,0.00264512890178106,
6.70842344717746));
#48714=CARTESIAN_POINT('Ctrl Pts',(11.9253586384648,0.00253840983232619,
7.79157655282255));
#48715=CARTESIAN_POINT('Ctrl Pts',(11.9236216864083,0.199145893570575,7.78138322237808));
#48716=CARTESIAN_POINT('Ctrl Pts',(12.0296403223963,1.40328729141077,7.71885651614953));
#48717=CARTESIAN_POINT('Ctrl Pts',(13.6166705510885,3.34441360725337,7.60399643413689));
#48718=CARTESIAN_POINT('Ctrl Pts',(17.0263976837988,2.99873559323853,7.44699630678466));
#48719=CARTESIAN_POINT('Ctrl Pts',(18.6190345729722,-0.0359373922966709,
7.2899961794324));
#48720=CARTESIAN_POINT('Ctrl Pts',(16.9664484412042,-3.03838498006983,7.13299605208014));
#48721=CARTESIAN_POINT('Ctrl Pts',(13.5505291268344,-3.3162835943375,6.97599592472789));
#48722=CARTESIAN_POINT('Ctrl Pts',(12.0165601959407,-1.36211545786235,6.86218942497536));
#48723=CARTESIAN_POINT('Ctrl Pts',(11.923255927005,-0.178620339789062,6.80071630100691));
#48724=CARTESIAN_POINT('Ctrl Pts',(11.9247764014775,-0.00242061498952133,
6.79157655282255));
#48725=CARTESIAN_POINT('Origin',(15.,0.,14.2084234471775));
#48726=CARTESIAN_POINT('',(11.9309505480454,-0.000995066888654084,8.79157655282255));
#48727=CARTESIAN_POINT('',(11.9216975306736,-0.000180300492997754,8.70842344717746));
#48728=CARTESIAN_POINT('',(11.9265,6.70613782525944E-14,14.2084234471775));
#48729=CARTESIAN_POINT('Ctrl Pts',(11.9216975306736,-0.000180300492997622,
8.70842344717746));
#48730=CARTESIAN_POINT('Ctrl Pts',(11.9225619574989,0.995939940607609,8.65661686252342));
#48731=CARTESIAN_POINT('Ctrl Pts',(12.9850426088341,2.99989628694768,8.5524769020853));
#48732=CARTESIAN_POINT('Ctrl Pts',(16.383329827636,3.34441452287188,8.39600356586309));
#48733=CARTESIAN_POINT('Ctrl Pts',(18.5526127662067,0.691124042072478,8.23900343851084));
#48734=CARTESIAN_POINT('Ctrl Pts',(17.5362337553543,-2.58190399634584,8.08200331115859));
#48735=CARTESIAN_POINT('Ctrl Pts',(14.2455896040548,-3.53971395275292,7.92500318380633));
#48736=CARTESIAN_POINT('Ctrl Pts',(12.1721380845128,-1.78183929043833,7.8004765624793));
#48737=CARTESIAN_POINT('Ctrl Pts',(11.928107441166,-0.386337687713779,7.72828331693634));
#48738=CARTESIAN_POINT('Ctrl Pts',(11.9301569186554,-0.00175543039446478,
7.70842344717746));
#48739=CARTESIAN_POINT('Ctrl Pts',(11.9309505480454,-0.000995066888653875,
8.79157655282255));
#48740=CARTESIAN_POINT('Ctrl Pts',(11.9326502109465,0.571148683183627,8.76205014374926));
#48741=CARTESIAN_POINT('Ctrl Pts',(12.3588112254404,2.15972684180816,8.68019035889189));
#48742=CARTESIAN_POINT('Ctrl Pts',(14.8994866243195,3.61781699652394,8.54599719825042));
#48743=CARTESIAN_POINT('Ctrl Pts',(17.9620970086125,2.07958747065415,8.38899707089818));
#48744=CARTESIAN_POINT('Ctrl Pts',(18.3685665845007,-1.32342808525659,8.23199694354591));
#48745=CARTESIAN_POINT('Ctrl Pts',(15.7544101894084,-3.53971298366467,8.07499681619367));
#48746=CARTESIAN_POINT('Ctrl Pts',(12.6774139888043,-2.64408967670503,7.92819001928588));
#48747=CARTESIAN_POINT('Ctrl Pts',(11.932539337532,-0.810252691562618,7.83371659816217));
#48748=CARTESIAN_POINT('Ctrl Pts',(11.9253586384648,0.00253840983232619,
7.79157655282255));
#48749=CARTESIAN_POINT('Origin',(15.,0.,14.2084234471775));
#48750=CARTESIAN_POINT('',(11.9222420001619,-0.00114382935434674,9.79157655282255));
#48751=CARTESIAN_POINT('',(11.9297705140734,0.00198364688382296,9.70842344717746));
#48752=CARTESIAN_POINT('',(11.9265,6.70613782525944E-14,14.2084234471775));
#48753=CARTESIAN_POINT('Ctrl Pts',(11.9297705140734,0.00198364688382347,
9.70842344717746));
#48754=CARTESIAN_POINT('Ctrl Pts',(11.9275592683916,0.36604807192143,9.68961715967868));
#48755=CARTESIAN_POINT('Ctrl Pts',(12.1545555502906,1.7405498801195,9.61847749639582));
#48756=CARTESIAN_POINT('Ctrl Pts',(14.1754458368614,3.52403461675767,9.49500445732887));
#48757=CARTESIAN_POINT('Ctrl Pts',(17.4844615229107,2.63176005547664,9.33800432997661));
#48758=CARTESIAN_POINT('Ctrl Pts',(18.565636725993,-0.620439089359897,9.18100420262437));
#48759=CARTESIAN_POINT('Ctrl Pts',(16.4494712699821,-3.31628450238807,9.0240040752721));
#48760=CARTESIAN_POINT('Ctrl Pts',(13.033551020433,-3.03838581184986,8.86700394791986));
#48761=CARTESIAN_POINT('Ctrl Pts',(11.9262816166307,-1.02667925906391,8.76181040522164));
#48762=CARTESIAN_POINT('Ctrl Pts',(11.9216887408183,-0.0103092698311159,
8.70895023830751));
#48763=CARTESIAN_POINT('Ctrl Pts',(11.9216975306736,-0.000180300492997622,
8.70842344717746));
#48764=CARTESIAN_POINT('Ctrl Pts',(11.9222420001619,-0.00114382935434687,
9.79157655282255));
#48765=CARTESIAN_POINT('Ctrl Pts',(11.9267950445754,0.938754987078744,9.74271706512043));
#48766=CARTESIAN_POINT('Ctrl Pts',(12.8851347215443,2.89342387288723,9.64152420163423));
#48767=CARTESIAN_POINT('Ctrl Pts',(16.1955038860992,3.41606118929613,9.48799796236394));
#48768=CARTESIAN_POINT('Ctrl Pts',(18.5087584392439,0.887308966009096,9.3309978350117));
#48769=CARTESIAN_POINT('Ctrl Pts',(17.6756754360527,-2.43710142000481,9.17399770765943));
#48770=CARTESIAN_POINT('Ctrl Pts',(14.4432887039958,-3.57613973602564,9.0169975803072));
#48771=CARTESIAN_POINT('Ctrl Pts',(12.2241286148511,-1.89728740549368,8.88952386202822));
#48772=CARTESIAN_POINT('Ctrl Pts',(11.9296376841916,-0.442933787892533,
8.81438351953334));
#48773=CARTESIAN_POINT('Ctrl Pts',(11.9309505480454,-0.000995066888653875,
8.79157655282255));
#48774=CARTESIAN_POINT('Origin',(15.,0.,14.2084234471775));
#48775=CARTESIAN_POINT('',(11.9284560106028,0.00245566734982605,10.7915765528225));
#48776=CARTESIAN_POINT('',(11.9275890856804,-0.00260766251225693,10.7084234471775));
#48777=CARTESIAN_POINT('',(11.9265,6.70613782525944E-14,14.2084234471775));
#48778=CARTESIAN_POINT('Ctrl Pts',(11.9275890856804,-0.00260766251225678,
10.7084234471775));
#48779=CARTESIAN_POINT('Ctrl Pts',(11.9337969642323,0.734391539461283,10.6702840810499));
#48780=CARTESIAN_POINT('Ctrl Pts',(12.5665847955819,2.49225272359552,10.5798113391382));
#48781=CARTESIAN_POINT('Ctrl Pts',(15.4855857629831,3.58648800243424,10.4370052214424));
#48782=CARTESIAN_POINT('Ctrl Pts',(18.2592872973176,1.57345505668517,10.2800050940901));
#48783=CARTESIAN_POINT('Ctrl Pts',(18.1103546151327,-1.85051527716861,10.1230049667379));
#48784=CARTESIAN_POINT('Ctrl Pts',(15.1723371249586,-3.61510816978504,9.96600483938563));
#48785=CARTESIAN_POINT('Ctrl Pts',(12.4502253736084,-2.31493586870828,9.82781099953215));
#48786=CARTESIAN_POINT('Ctrl Pts',(11.9337126333884,-0.647055676830039,
9.74195053546276));
#48787=CARTESIAN_POINT('Ctrl Pts',(11.9297705140734,0.00198364688382347,
9.70842344717746));
#48788=CARTESIAN_POINT('Ctrl Pts',(11.9284560106028,0.0024556673498264,
10.7915765528226));
#48789=CARTESIAN_POINT('Ctrl Pts',(11.9260692195737,0.309140112596412,10.7757173622757));
#48790=CARTESIAN_POINT('Ctrl Pts',(12.1080878285752,1.62508037117336,10.7075247959448));
#48791=CARTESIAN_POINT('Ctrl Pts',(13.9810651784412,3.47279856287599,10.5869988538297));
#48792=CARTESIAN_POINT('Ctrl Pts',(17.3344994031312,2.76565299665532,10.4299987264775));
#48793=CARTESIAN_POINT('Ctrl Pts',(18.5945871152999,-0.421511967551375,
10.2729985991252));
#48794=CARTESIAN_POINT('Ctrl Pts',(16.6313630370479,-3.23068676566348,10.115998471773));
#48795=CARTESIAN_POINT('Ctrl Pts',(13.205285741413,-3.14288213812672,9.9589983444207));
#48796=CARTESIAN_POINT('Ctrl Pts',(11.9539254885605,-1.14120637601563,9.85085770477057));
#48797=CARTESIAN_POINT('Ctrl Pts',(11.921918280707,-0.0679702217342443,
9.79505044090452));
#48798=CARTESIAN_POINT('Ctrl Pts',(11.9222420001619,-0.00114382935434687,
9.79157655282255));
#48799=CARTESIAN_POINT('Origin',(15.,0.,14.2084234471775));
#48800=CARTESIAN_POINT('',(11.9297760945785,-0.00333806817183438,11.7915765528226));
#48801=CARTESIAN_POINT('',(11.9228311771842,0.00152130202986591,11.7084234471775));
#48802=CARTESIAN_POINT('',(11.9265,6.70613782525944E-14,14.2084234471775));
#48803=CARTESIAN_POINT('',(14.2062007174671,-2.96922295374568,12.));
#48804=CARTESIAN_POINT('Ctrl Pts',(14.2062007174671,-2.96922295374568,12.));
#48805=CARTESIAN_POINT('Ctrl Pts',(13.2298599415769,-2.70820563726846,11.9476666242159));
#48806=CARTESIAN_POINT('Ctrl Pts',(12.1284916041782,-1.6759644246982,11.8781921418234));
#48807=CARTESIAN_POINT('Ctrl Pts',(11.9274999800733,-0.33505537898738,11.8087176594309));
#48808=CARTESIAN_POINT('Ctrl Pts',(11.9297760945785,-0.00333806817183434,
11.7915765528225));
#48809=CARTESIAN_POINT('',(15.7957331921886,-2.97400465723624,12.));
#48810=CARTESIAN_POINT('Origin',(15.,0.,12.));
#48811=CARTESIAN_POINT('Ctrl Pts',(15.7957405241459,-2.97402278592475,12.));
#48812=CARTESIAN_POINT('Ctrl Pts',(14.8659292530302,-3.21955068215558,11.9500021225376));
#48813=CARTESIAN_POINT('Ctrl Pts',(12.809912552641,-2.78622279751186,11.8528099382634));
#48814=CARTESIAN_POINT('Ctrl Pts',(11.9286986705132,-0.906613920335824,
11.7556177539892));
#48815=CARTESIAN_POINT('Ctrl Pts',(11.9228311771842,0.00152130202986659,
11.7084234471775));
#48816=CARTESIAN_POINT('Origin',(15.,1.36827403442078E-16,4.));
#48817=CARTESIAN_POINT('Ctrl Pts',(13.086534003335,1.63598720337497,4.));
#48818=CARTESIAN_POINT('Ctrl Pts',(13.0243671614557,1.57756563722365,4.));
#48819=CARTESIAN_POINT('Ctrl Pts',(12.9655713261624,1.51589246301216,4.));
#48820=CARTESIAN_POINT('Ctrl Pts',(12.9101605215997,1.45134356594541,4.));
#48821=CARTESIAN_POINT('Ctrl Pts',(12.8533994594265,1.38522173305508,4.));
#48822=CARTESIAN_POINT('Ctrl Pts',(12.8001899401135,1.31608182626898,4.));
#48823=CARTESIAN_POINT('Ctrl Pts',(12.7505758639603,1.24428161564212,4.));
#48824=CARTESIAN_POINT('Ctrl Pts',(12.737567030614,1.22545556774005,4.));
#48825=CARTESIAN_POINT('Ctrl Pts',(12.7248055528518,1.20644640781821,4.));
#48826=CARTESIAN_POINT('Ctrl Pts',(12.7122926030956,1.18726014528907,4.));
#48827=CARTESIAN_POINT('Ctrl Pts',(12.7022174307361,1.17181175736453,4.));
#48828=CARTESIAN_POINT('Ctrl Pts',(12.6923030248513,1.15624777849328,4.));
#48829=CARTESIAN_POINT('Ctrl Pts',(12.6825586157748,1.14058556199816,4.));
#48830=CARTESIAN_POINT('Ctrl Pts',(12.6350797654636,1.06427267050556,4.));
#48831=CARTESIAN_POINT('Ctrl Pts',(12.5915831545383,0.985554475328281,4.00000000000001));
#48832=CARTESIAN_POINT('Ctrl Pts',(12.5521056896097,0.904822546167765,4.00000000000001));
#48833=CARTESIAN_POINT('Ctrl Pts',(12.5205631790518,0.840317701884819,4.));
#48834=CARTESIAN_POINT('Ctrl Pts',(12.4915870127793,0.774526199173173,4.));
#48835=CARTESIAN_POINT('Ctrl Pts',(12.4652125787776,0.707630559635218,4.));
#48836=CARTESIAN_POINT('Ctrl Pts',(12.4565302425272,0.685608838292681,4.));
#48837=CARTESIAN_POINT('Ctrl Pts',(12.4481299823828,0.663467358107674,4.));
#48838=CARTESIAN_POINT('Ctrl Pts',(12.4400134491405,0.641212348322469,4.));
#48839=CARTESIAN_POINT('Ctrl Pts',(12.4326491678695,0.6210199648435,4.));
#48840=CARTESIAN_POINT('Ctrl Pts',(12.4255170259942,0.600729502784082,4.));
#48841=CARTESIAN_POINT('Ctrl Pts',(12.41862769741,0.580374130450127,4.));
#48842=CARTESIAN_POINT('Ctrl Pts',(12.3890480800735,0.492977497088245,4.));
#48843=CARTESIAN_POINT('Ctrl Pts',(12.363907391977,0.404299179172776,4.00000000000001));
#48844=CARTESIAN_POINT('Ctrl Pts',(12.3432403919349,0.314735964380019,4.00000000000001));
#48845=CARTESIAN_POINT('Ctrl Pts',(12.322257026321,0.223801736977766,4.00000000000001));
#48846=CARTESIAN_POINT('Ctrl Pts',(12.3058848583804,0.131954509394712,4.));
#48847=CARTESIAN_POINT('Ctrl Pts',(12.2942020415478,0.039576420273935,4.));
#48848=CARTESIAN_POINT('Ctrl Pts',(12.2826102453471,-0.0520819526881022,
4.));
#48849=CARTESIAN_POINT('Ctrl Pts',(12.2756346673422,-0.14426387445687,4.));
#48850=CARTESIAN_POINT('Ctrl Pts',(12.2733985971608,-0.236615283315844,
4.));
#48851=CARTESIAN_POINT('Ctrl Pts',(12.2723186623648,-0.28121741642928,4.));
#48852=CARTESIAN_POINT('Ctrl Pts',(12.2723449592516,-0.325859284098739,
4.));
#48853=CARTESIAN_POINT('Ctrl Pts',(12.2734957210626,-0.370501641907857,
4.));
#48854=CARTESIAN_POINT('Ctrl Pts',(12.2738658684163,-0.384861043177254,
4.));
#48855=CARTESIAN_POINT('Ctrl Pts',(12.2743523774935,-0.399220495972395,
4.));
#48856=CARTESIAN_POINT('Ctrl Pts',(12.2749559214615,-0.413578694513598,
4.));
#48857=CARTESIAN_POINT('Ctrl Pts',(12.2755868612803,-0.428588635239398,
4.));
#48858=CARTESIAN_POINT('Ctrl Pts',(12.2763453773817,-0.443588732674977,
4.));
#48859=CARTESIAN_POINT('Ctrl Pts',(12.2772314223084,-0.458571999977678,
4.));
#48860=CARTESIAN_POINT('Ctrl Pts',(12.2828802428556,-0.554095133908471,
4.));
#48861=CARTESIAN_POINT('Ctrl Pts',(12.2937114584574,-0.649002595692518,
4.));
#48862=CARTESIAN_POINT('Ctrl Pts',(12.3097976800713,-0.742900147453328,
4.));
#48863=CARTESIAN_POINT('Ctrl Pts',(12.3112861449746,-0.75158852771142,4.));
#48864=CARTESIAN_POINT('Ctrl Pts',(12.3128196370525,-0.760268274419424,
4.));
#48865=CARTESIAN_POINT('Ctrl Pts',(12.3143982352413,-0.768939082485976,
4.));
#48866=CARTESIAN_POINT('Ctrl Pts',(12.3307867311623,-0.858956607935255,
4.));
#48867=CARTESIAN_POINT('Ctrl Pts',(12.3520323002905,-0.948010485772638,
4.));
#48868=CARTESIAN_POINT('Ctrl Pts',(12.3778326203319,-1.03586583972401,4.));
#48869=CARTESIAN_POINT('Ctrl Pts',(12.4042241967268,-1.12573454219727,4.));
#48870=CARTESIAN_POINT('Ctrl Pts',(12.435381875245,-1.21434985801567,4.));
#48871=CARTESIAN_POINT('Ctrl Pts',(12.4710363747919,-1.30145748669412,4.));
#48872=CARTESIAN_POINT('Ctrl Pts',(12.4909273060557,-1.35005308827618,4.));
#48873=CARTESIAN_POINT('Ctrl Pts',(12.5122187298043,-1.39817934130794,4.));
#48874=CARTESIAN_POINT('Ctrl Pts',(12.534870586159,-1.44579043537726,4.));
#48875=CARTESIAN_POINT('Ctrl Pts',(12.5412077066689,-1.45911019319316,4.));
#48876=CARTESIAN_POINT('Ctrl Pts',(12.5476516035311,-1.47239000998161,4.));
#48877=CARTESIAN_POINT('Ctrl Pts',(12.5541943737652,-1.48561501829369,4.));
#48878=CARTESIAN_POINT('Ctrl Pts',(12.5969523561364,-1.57204242626194,4.));
#48879=CARTESIAN_POINT('Ctrl Pts',(12.6439961654632,-1.65627338500264,4.));
#48880=CARTESIAN_POINT('Ctrl Pts',(12.6949857265575,-1.73805452373085,4.));
#48881=CARTESIAN_POINT('Ctrl Pts',(12.7469808269627,-1.82144842687817,4.));
#48882=CARTESIAN_POINT('Ctrl Pts',(12.8030791489228,-1.90229571208266,4.));
#48883=CARTESIAN_POINT('Ctrl Pts',(12.8629750013787,-1.98032077373009,4.));
#48884=CARTESIAN_POINT('Ctrl Pts',(12.9233424571313,-2.05896018302908,4.));
#48885=CARTESIAN_POINT('Ctrl Pts',(12.9875679362272,-2.13473359370643,4.));
#48886=CARTESIAN_POINT('Ctrl Pts',(13.0553877098439,-2.20733955177719,4.));
#48887=CARTESIAN_POINT('Ctrl Pts',(13.0913230991629,-2.24581097730712,4.));
#48888=CARTESIAN_POINT('Ctrl Pts',(13.1282683996108,-2.28339271539353,4.));
#48889=CARTESIAN_POINT('Ctrl Pts',(13.1661892287502,-2.32003649064048,4.));
#48890=CARTESIAN_POINT('Ctrl Pts',(13.1814900570711,-2.33482203533466,4.));
#48891=CARTESIAN_POINT('Ctrl Pts',(13.196949744001,-2.34945484110134,4.));
#48892=CARTESIAN_POINT('Ctrl Pts',(13.2125661689314,-2.36393160001069,4.));
#48893=CARTESIAN_POINT('Ctrl Pts',(13.2232570858249,-2.37384230794012,4.));
#48894=CARTESIAN_POINT('Ctrl Pts',(13.2340146157559,-2.3836735202466,4.));
#48895=CARTESIAN_POINT('Ctrl Pts',(13.2448364129784,-2.39342320679516,4.));
#48896=CARTESIAN_POINT('Ctrl Pts',(13.320625051765,-2.46170349859172,4.));
#48897=CARTESIAN_POINT('Ctrl Pts',(13.3995829817648,-2.52600647852482,4.));
#48898=CARTESIAN_POINT('Ctrl Pts',(13.4813873531473,-2.58604589859231,4.));
#48899=CARTESIAN_POINT('Ctrl Pts',(13.5632614554873,-2.64613649693043,4.));
#48900=CARTESIAN_POINT('Ctrl Pts',(13.6479874247046,-2.70195710712452,4.));
#48901=CARTESIAN_POINT('Ctrl Pts',(13.7352864859208,-2.75319451696124,4.));
#48902=CARTESIAN_POINT('Ctrl Pts',(13.8208945029142,-2.80343942212848,4.));
#48903=CARTESIAN_POINT('Ctrl Pts',(13.9089775477651,-2.84927765377448,4.));
#48904=CARTESIAN_POINT('Ctrl Pts',(13.9993066119595,-2.89037749094858,4.));
#48905=CARTESIAN_POINT('Ctrl Pts',(14.025515470362,-2.90230255429857,4.));
#48906=CARTESIAN_POINT('Ctrl Pts',(14.0519135997525,-2.91382843622988,4.));
#48907=CARTESIAN_POINT('Ctrl Pts',(14.0784958352494,-2.92494631785187,4.));
#48908=CARTESIAN_POINT('Ctrl Pts',(14.1199798960696,-2.94229681034347,4.));
#48909=CARTESIAN_POINT('Ctrl Pts',(14.1619123028466,-2.95865373590191,4.));
#48910=CARTESIAN_POINT('Ctrl Pts',(14.204261268307,-2.97402368063354,4.));
#48911=CARTESIAN_POINT('Ctrl Pts',(15.7937992825329,-2.9692229537457,4.));
#48912=CARTESIAN_POINT('Ctrl Pts',(15.8886556608518,-2.93452406683594,4.));
#48913=CARTESIAN_POINT('Ctrl Pts',(15.9814715788842,-2.89484190048077,4.));
#48914=CARTESIAN_POINT('Ctrl Pts',(16.0720047548823,-2.85049467748599,4.));
#48915=CARTESIAN_POINT('Ctrl Pts',(16.1637866430073,-2.80553577910774,4.));
#48916=CARTESIAN_POINT('Ctrl Pts',(16.2532230529932,-2.75578154813471,4.));
#48917=CARTESIAN_POINT('Ctrl Pts',(16.3400275203182,-2.70152291880737,4.));
#48918=CARTESIAN_POINT('Ctrl Pts',(16.3646888442304,-2.686107932988,4.));
#48919=CARTESIAN_POINT('Ctrl Pts',(16.389137491053,-2.67032916740001,4.));
#48920=CARTESIAN_POINT('Ctrl Pts',(16.4133662837328,-2.65419282892726,4.));
#48921=CARTESIAN_POINT('Ctrl Pts',(16.4325631402962,-2.64140775212984,4.));
#48922=CARTESIAN_POINT('Ctrl Pts',(16.4516239542716,-2.62839666993241,4.));
#48923=CARTESIAN_POINT('Ctrl Pts',(16.4705261961219,-2.61517619923621,4.));
#48924=CARTESIAN_POINT('Ctrl Pts',(16.5532306656362,-2.55733163115156,4.));
#48925=CARTESIAN_POINT('Ctrl Pts',(16.6329816584356,-2.49543011909309,4.));
#48926=CARTESIAN_POINT('Ctrl Pts',(16.7095117106738,-2.42976651841151,4.));
#48927=CARTESIAN_POINT('Ctrl Pts',(16.7679773228431,-2.37960239988795,4.));
#48928=CARTESIAN_POINT('Ctrl Pts',(16.8245624524955,-2.32724171199687,4.));
#48929=CARTESIAN_POINT('Ctrl Pts',(16.8791308185435,-2.27280449707864,4.));
#48930=CARTESIAN_POINT('Ctrl Pts',(16.9076285190194,-2.2443752887693,4.));
#48931=CARTESIAN_POINT('Ctrl Pts',(16.9355759205114,-2.21537960309138,4.));
#48932=CARTESIAN_POINT('Ctrl Pts',(16.9629517841853,-2.18583377975445,4.));
#48933=CARTESIAN_POINT('Ctrl Pts',(16.9740993314633,-2.17380261732463,4.));
#48934=CARTESIAN_POINT('Ctrl Pts',(16.9851523150081,-2.16167987026619,4.));
#48935=CARTESIAN_POINT('Ctrl Pts',(16.9960991984116,-2.14947815004889,4.));
#48936=CARTESIAN_POINT('Ctrl Pts',(17.061864093391,-2.07617465177648,4.));
#48937=CARTESIAN_POINT('Ctrl Pts',(17.1238952962526,-1.9999250033291,4.));
#48938=CARTESIAN_POINT('Ctrl Pts',(17.1819478816723,-1.92100525783345,4.));
#48939=CARTESIAN_POINT('Ctrl Pts',(17.2389325987962,-1.84353722880334,4.));
#48940=CARTESIAN_POINT('Ctrl Pts',(17.2920840747574,-1.76349564200828,4.));
#48941=CARTESIAN_POINT('Ctrl Pts',(17.3411263889919,-1.681119910375,4.));
#48942=CARTESIAN_POINT('Ctrl Pts',(17.3892346863819,-1.6003130345782,4.));
#48943=CARTESIAN_POINT('Ctrl Pts',(17.4333891346359,-1.51725940586905,4.));
#48944=CARTESIAN_POINT('Ctrl Pts',(17.473281665729,-1.43217460910322,4.));
#48945=CARTESIAN_POINT('Ctrl Pts',(17.4935758753293,-1.38889009814213,4.));
#48946=CARTESIAN_POINT('Ctrl Pts',(17.5127663147042,-1.34507981852401,4.));
#48947=CARTESIAN_POINT('Ctrl Pts',(17.5308071984732,-1.30077191375233,4.));
#48948=CARTESIAN_POINT('Ctrl Pts',(17.5396600651807,-1.27902952130341,4.));
#48949=CARTESIAN_POINT('Ctrl Pts',(17.548236065603,-1.25716730274661,4.));
#48950=CARTESIAN_POINT('Ctrl Pts',(17.5565294575664,-1.23518860043795,4.));
#48951=CARTESIAN_POINT('Ctrl Pts',(17.5612619499656,-1.22264680305532,4.));
#48952=CARTESIAN_POINT('Ctrl Pts',(17.5659011120686,-1.21007041067208,4.));
#48953=CARTESIAN_POINT('Ctrl Pts',(17.5704433141742,-1.19746790314509,4.));
#48954=CARTESIAN_POINT('Ctrl Pts',(17.601949668132,-1.11005236027246,4.));
#48955=CARTESIAN_POINT('Ctrl Pts',(17.6288373085193,-1.02126995392761,4.));
#48956=CARTESIAN_POINT('Ctrl Pts',(17.6508530784154,-0.931342019285625,
4.));
#48957=CARTESIAN_POINT('Ctrl Pts',(17.6541059208438,-0.918055116184408,
4.));
#48958=CARTESIAN_POINT('Ctrl Pts',(17.6572523179739,-0.90474318860678,4.));
#48959=CARTESIAN_POINT('Ctrl Pts',(17.6602913566075,-0.891406935242469,
4.));
#48960=CARTESIAN_POINT('Ctrl Pts',(17.6812030503878,-0.79963987330047,4.));
#48961=CARTESIAN_POINT('Ctrl Pts',(17.6970357825963,-0.706720788882977,
4.));
#48962=CARTESIAN_POINT('Ctrl Pts',(17.7078979433461,-0.613041608366267,
4.));
#48963=CARTESIAN_POINT('Ctrl Pts',(17.71918010274,-0.515740208504458,4.));
#48964=CARTESIAN_POINT('Ctrl Pts',(17.7250998267343,-0.417617597139405,
4.));
#48965=CARTESIAN_POINT('Ctrl Pts',(17.7257219253175,-0.319126306900475,
4.));
#48966=CARTESIAN_POINT('Ctrl Pts',(17.7259028938113,-0.290475188042702,
4.));
#48967=CARTESIAN_POINT('Ctrl Pts',(17.7256352115795,-0.261793020088843,
4.));
#48968=CARTESIAN_POINT('Ctrl Pts',(17.7249196338,-0.233091376404626,4.));
#48969=CARTESIAN_POINT('Ctrl Pts',(17.7245239501318,-0.217220604586536,
4.));
#48970=CARTESIAN_POINT('Ctrl Pts',(17.7239913108662,-0.201343881980789,
4.));
#48971=CARTESIAN_POINT('Ctrl Pts',(17.7233217966467,-0.185463198608965,
4.));
#48972=CARTESIAN_POINT('Ctrl Pts',(17.7227411089474,-0.171689454568016,
4.));
#48973=CARTESIAN_POINT('Ctrl Pts',(17.7220574547657,-0.157914135821034,
4.));
#48974=CARTESIAN_POINT('Ctrl Pts',(17.7212718008001,-0.144150654953,4.));
#48975=CARTESIAN_POINT('Ctrl Pts',(17.7159690064325,-0.0512536391956395,
4.));
#48976=CARTESIAN_POINT('Ctrl Pts',(17.7060179260155,0.0412556969053557,
4.));
#48977=CARTESIAN_POINT('Ctrl Pts',(17.691537290537,0.133004324856137,4.));
#48978=CARTESIAN_POINT('Ctrl Pts',(17.6770974224585,0.224494652470098,4.));
#48979=CARTESIAN_POINT('Ctrl Pts',(17.6581530629752,0.315229493843254,4.));
#48980=CARTESIAN_POINT('Ctrl Pts',(17.6347733990709,0.404821867293602,4.));
#48981=CARTESIAN_POINT('Ctrl Pts',(17.6117974920603,0.492867018399034,4.));
#48982=CARTESIAN_POINT('Ctrl Pts',(17.5845376887683,0.579809603493695,4.));
#48983=CARTESIAN_POINT('Ctrl Pts',(17.5530192634714,0.665253146715262,4.));
#48984=CARTESIAN_POINT('Ctrl Pts',(17.5376266260196,0.706981166786664,4.));
#48985=CARTESIAN_POINT('Ctrl Pts',(17.521217712657,0.748351139728866,4.));
#48986=CARTESIAN_POINT('Ctrl Pts',(17.5037923624592,0.789313445373718,4.));
#48987=CARTESIAN_POINT('Ctrl Pts',(17.4980299458858,0.802859334911291,4.));
#48988=CARTESIAN_POINT('Ctrl Pts',(17.4921563593103,0.816360622497498,4.));
#48989=CARTESIAN_POINT('Ctrl Pts',(17.4861715515314,0.829815450098292,4.));
#48990=CARTESIAN_POINT('Ctrl Pts',(17.4804842577731,0.842601417477522,4.));
#48991=CARTESIAN_POINT('Ctrl Pts',(17.4746999465266,0.855337690933622,4.));
#48992=CARTESIAN_POINT('Ctrl Pts',(17.4688205030047,0.868019526422757,4.));
#48993=CARTESIAN_POINT('Ctrl Pts',(17.4313685751689,0.948802543693164,4.));
#48994=CARTESIAN_POINT('Ctrl Pts',(17.3900398049897,1.02742425086957,4.));
#48995=CARTESIAN_POINT('Ctrl Pts',(17.3448999527151,1.10353609749938,4.));
#48996=CARTESIAN_POINT('Ctrl Pts',(17.3005164856713,1.17837257715787,4.));
#48997=CARTESIAN_POINT('Ctrl Pts',(17.2524481398624,1.25078327494736,4.));
#48998=CARTESIAN_POINT('Ctrl Pts',(17.2007210868077,1.32040265351989,4.));
#48999=CARTESIAN_POINT('Ctrl Pts',(17.1505256542607,1.38796062589101,4.));
#49000=CARTESIAN_POINT('Ctrl Pts',(17.0968845380256,1.45289058144554,4.));
#49001=CARTESIAN_POINT('Ctrl Pts',(17.0397936511852,1.5148180351349,4.));
#49002=CARTESIAN_POINT('Ctrl Pts',(17.0255930287153,1.53022169128796,4.));
#49003=CARTESIAN_POINT('Ctrl Pts',(17.0111788466503,1.54543936332989,4.));
#49004=CARTESIAN_POINT('Ctrl Pts',(16.9965508084827,1.56046483491105,4.));
#49005=CARTESIAN_POINT('Ctrl Pts',(16.9706944922369,1.58702364891564,4.));
#49006=CARTESIAN_POINT('Ctrl Pts',(16.9441700096348,1.61298203696882,4.));
#49007=CARTESIAN_POINT('Ctrl Pts',(16.9170033607454,1.6383265094434,4.));
#49008=CARTESIAN_POINT('Origin',(15.,0.,14.2084234471775));
#49009=CARTESIAN_POINT('Ctrl Pts',(11.9228311771842,0.0015213020298664,
11.7084234471775));
#49010=CARTESIAN_POINT('Ctrl Pts',(11.9221922557771,0.100409703179003,11.7032843782051));
#49011=CARTESIAN_POINT('Ctrl Pts',(11.9710108327432,1.20571704782255,11.6458119334487));
#49012=CARTESIAN_POINT('Ctrl Pts',(13.3048024582519,3.19795728077006,11.5360061129082));
#49013=CARTESIAN_POINT('Ctrl Pts',(16.7319486542021,3.17774782202826,11.3790059855559));
#49014=CARTESIAN_POINT('Ctrl Pts',(18.606042966971,0.308570934784431,11.2220058582037));
#49015=CARTESIAN_POINT('Ctrl Pts',(17.246562375271,-2.83758641060089,11.0650057308514));
#49016=CARTESIAN_POINT('Ctrl Pts',(13.8725685599584,-3.4391081414099,10.9080056034992));
#49017=CARTESIAN_POINT('Ctrl Pts',(12.0835901505745,-1.55983373126709,10.7891448422745));
#49018=CARTESIAN_POINT('Ctrl Pts',(11.9252787513183,-0.276890505982443,
10.7226174568339));
#49019=CARTESIAN_POINT('Ctrl Pts',(11.9275890856804,-0.00260766251225678,
10.7084234471775));
#49020=CARTESIAN_POINT('Ctrl Pts',(11.9297760945785,-0.00333806817183434,
11.7915765528225));
#49021=CARTESIAN_POINT('Ctrl Pts',(11.9344491671038,0.677708095250012,11.7563842836469));
#49022=CARTESIAN_POINT('Ctrl Pts',(12.4898049314569,2.38075616290146,11.6688586386871));
#49023=CARTESIAN_POINT('Ctrl Pts',(15.2863460006058,3.60696666543133,11.5289996179432));
#49024=CARTESIAN_POINT('Ctrl Pts',(18.1665668486981,1.75247841941832,11.371999490591));
#49025=CARTESIAN_POINT('Ctrl Pts',(18.2084706556688,-1.6752137223659,11.2149993632387));
#49026=CARTESIAN_POINT('Ctrl Pts',(15.3727057323674,-3.59983386165072,11.0579992358865));
#49027=CARTESIAN_POINT('Ctrl Pts',(12.5232213208654,-2.42851998200457,10.9168582990811));
#49028=CARTESIAN_POINT('Ctrl Pts',(11.9339453360424,-0.702880789277512,
10.8280507380598));
#49029=CARTESIAN_POINT('Ctrl Pts',(11.9284560106028,0.0024556673498264,
10.7915765528226));
#49030=CARTESIAN_POINT('Ctrl Pts',(16.9134659966651,1.63598720337493,12.));
#49031=CARTESIAN_POINT('Ctrl Pts',(17.4514117960785,1.00680074451815,11.9476666242159));
#49032=CARTESIAN_POINT('Ctrl Pts',(17.8499101160228,-0.812800245940048,
11.8429998726477));
#49033=CARTESIAN_POINT('Ctrl Pts',(15.8909226224913,-2.8292934693942,11.6859997452955));
#49034=CARTESIAN_POINT('Ctrl Pts',(13.1331777991764,-2.30192506894816,11.5289996179432));
#49035=CARTESIAN_POINT('Ctrl Pts',(12.0494015740803,0.286239346000545,11.371999490591));
#49036=CARTESIAN_POINT('Ctrl Pts',(13.6114658170324,2.61944280277814,11.2149993632387));
#49037=CARTESIAN_POINT('Ctrl Pts',(16.4186369731426,2.60288926043798,11.0579992358865));
#49038=CARTESIAN_POINT('Ctrl Pts',(17.9537052771594,0.252750066152531,10.9009991085342));
#49039=CARTESIAN_POINT('Ctrl Pts',(16.8401564274426,-2.32426347443882,10.743998981182));
#49040=CARTESIAN_POINT('Ctrl Pts',(14.0765223197317,-2.81696917065216,10.5869988538297));
#49041=CARTESIAN_POINT('Ctrl Pts',(12.1409791666289,-0.783732381279285,
10.4299987264775));
#49042=CARTESIAN_POINT('Ctrl Pts',(12.7691475978345,1.95231594579313,10.2729985991252));
#49043=CARTESIAN_POINT('Ctrl Pts',(15.3977426901935,2.93768783020276,10.1159984717729));
#49044=CARTESIAN_POINT('Ctrl Pts',(17.6696781425075,1.28881506595247,9.95899834442072));
#49045=CARTESIAN_POINT('Ctrl Pts',(17.5476875690895,-1.51575474549275,9.80199821706844));
#49046=CARTESIAN_POINT('Ctrl Pts',(15.1411611231766,-2.96113057342894,9.6449980897162));
#49047=CARTESIAN_POINT('Ctrl Pts',(12.6080541376564,-1.75123331751949,9.48799796236395));
#49048=CARTESIAN_POINT('Ctrl Pts',(12.2198279573789,1.02901222386683,9.33099783501168));
#49049=CARTESIAN_POINT('Ctrl Pts',(14.3246087178457,2.88653234022692,9.17399770765945));
#49050=CARTESIAN_POINT('Ctrl Pts',(17.0350193212714,2.15567136478361,9.01699758030717));
#49051=CARTESIAN_POINT('Ctrl Pts',(17.920608575789,-0.508200880905659,8.85999745295495));
#49052=CARTESIAN_POINT('Ctrl Pts',(16.1872601015714,-2.71636448178362,8.70299732560267));
#49053=CARTESIAN_POINT('Ctrl Pts',(13.3892841040964,-2.48873801247178,8.54599719825043));
#49054=CARTESIAN_POINT('Ctrl Pts',(12.0356525030592,-0.0294362811014349,
8.38899707089817));
#49055=CARTESIAN_POINT('Ctrl Pts',(13.3401797411332,2.45626124056312,8.23199694354592));
#49056=CARTESIAN_POINT('Ctrl Pts',(16.1330837289975,2.73940574632503,8.07499681619367));
#49057=CARTESIAN_POINT('Ctrl Pts',(17.9099406666424,0.566098837129481,7.91799668884141));
#49058=CARTESIAN_POINT('Ctrl Pts',(17.0774258920138,-2.11483432920145,7.76099656148916));
#49059=CARTESIAN_POINT('Ctrl Pts',(14.3820633896886,-2.89937526470001,7.6039964341369));
#49060=CARTESIAN_POINT('Ctrl Pts',(12.240810574834,-1.08401858364571,7.44699630678465));
#49061=CARTESIAN_POINT('Ctrl Pts',(12.5737493864543,1.70338795860876,7.28999617943239));
#49062=CARTESIAN_POINT('Ctrl Pts',(15.0823304026287,2.96335018127148,7.13299605208015));
#49063=CARTESIAN_POINT('Ctrl Pts',(17.5170849510905,1.56604785867891,6.97599592472789));
#49064=CARTESIAN_POINT('Ctrl Pts',(17.6947452874587,-1.23554458602037,6.81899579737564));
#49065=CARTESIAN_POINT('Ctrl Pts',(15.4560016501892,-2.92921237979097,6.66199567002338));
#49066=CARTESIAN_POINT('Ctrl Pts',(12.8083570016989,-1.99622726741817,6.50499554267113));
#49067=CARTESIAN_POINT('Ctrl Pts',(12.1259795712872,0.726793862646375,6.34799541531888));
#49068=CARTESIAN_POINT('Ctrl Pts',(14.0207639954511,2.79809220508692,6.19099528796662));
#49069=CARTESIAN_POINT('Ctrl Pts',(16.793638419534,2.3603139527537,6.03399516061437));
#49070=CARTESIAN_POINT('Ctrl Pts',(17.9581406885776,-0.193979547267846,
5.87699503326211));
#49071=CARTESIAN_POINT('Ctrl Pts',(16.4700486085461,-2.57433151465002,5.71999490590987));
#49072=CARTESIAN_POINT('Ctrl Pts',(13.6637522053085,-2.64625223032612,5.56299477855761));
#49073=CARTESIAN_POINT('Ctrl Pts',(12.0556774054966,-0.345259977325435,
5.40599465120536));
#49074=CARTESIAN_POINT('Ctrl Pts',(13.0878139143641,2.26534344968177,5.2489945238531));
#49075=CARTESIAN_POINT('Ctrl Pts',(15.8346085061802,2.84456586771516,5.09199439650085));
#49076=CARTESIAN_POINT('Ctrl Pts',(17.8330357993722,0.87308907652308,4.9349942691486));
#49077=CARTESIAN_POINT('Ctrl Pts',(17.2909861426673,-1.8813930887419,4.77799414179634));
#49078=CARTESIAN_POINT('Ctrl Pts',(14.6947169782024,-2.94862097263666,4.62099401444409));
#49079=CARTESIAN_POINT('Ctrl Pts',(12.3719451483433,-1.37216452037615,4.46399388709184));
#49080=CARTESIAN_POINT('Ctrl Pts',(12.4062682448688,1.4354510150691,4.30699375973958));
#49081=CARTESIAN_POINT('Ctrl Pts',(14.7654540928384,2.95446651190592,4.14999363238733));
#49082=CARTESIAN_POINT('Ctrl Pts',(17.3368403233694,1.82697070537499,3.99299350503508));
#49083=CARTESIAN_POINT('Ctrl Pts',(17.8090202723047,-0.94447711406392,3.83599337768282));
#49084=CARTESIAN_POINT('Ctrl Pts',(16.4499195044998,-2.21828784507026,3.73132662611465));
#49085=CARTESIAN_POINT('Ctrl Pts',(15.6501999979751,-2.43208680203507,3.67899325033057));
#49086=CARTESIAN_POINT('Ctrl Pts',(17.0543315503421,1.75642532122682,12.1070022498898));
#49087=CARTESIAN_POINT('Ctrl Pts',(17.6318798475343,1.08091940905997,12.0546688741057));
#49088=CARTESIAN_POINT('Ctrl Pts',(18.0597148196982,-0.872636980364766,
11.9500021225376));
#49089=CARTESIAN_POINT('Ctrl Pts',(15.9565105706019,-3.03758041662798,11.7930019951853));
#49090=CARTESIAN_POINT('Ctrl Pts',(12.9957460688013,-2.47138820543743,11.6360018678331));
#49091=CARTESIAN_POINT('Ctrl Pts',(11.8321843976736,0.307311716258913,11.4790017404808));
#49092=CARTESIAN_POINT('Ctrl Pts',(13.5092446974389,2.81228096210878,11.3220016131285));
#49093=CARTESIAN_POINT('Ctrl Pts',(16.5230742001624,2.79450878096808,11.1650014857763));
#49094=CARTESIAN_POINT('Ctrl Pts',(18.1711511737633,0.271357022363162,11.008001358424));
#49095=CARTESIAN_POINT('Ctrl Pts',(16.9756250767187,-2.49537111982618,10.8510012310718));
#49096=CARTESIAN_POINT('Ctrl Pts',(14.0085377331406,-3.02434882757141,10.6940011037195));
#49097=CARTESIAN_POINT('Ctrl Pts',(11.9305037500974,-0.841429197431721,
10.5370009763673));
#49098=CARTESIAN_POINT('Ctrl Pts',(12.604916689446,2.09604155530799,10.380000849015));
#49099=CARTESIAN_POINT('Ctrl Pts',(15.4270237144567,3.15395455427992,10.2230007216628));
#49100=CARTESIAN_POINT('Ctrl Pts',(17.8662145274442,1.38369506286337,10.0660005943105));
#49101=CARTESIAN_POINT('Ctrl Pts',(17.7352432511039,-1.62734158938471,9.90900046695827));
#49102=CARTESIAN_POINT('Ctrl Pts',(15.1515531237706,-3.17912310554764,9.752000339606));
#49103=CARTESIAN_POINT('Ctrl Pts',(12.4319638497434,-1.88015562464175,9.59500021225376));
#49104=CARTESIAN_POINT('Ctrl Pts',(12.0151572316991,1.10476605325709,9.4380000849015));
#49105=CARTESIAN_POINT('Ctrl Pts',(14.2748877575176,3.09903309907051,9.28099995754925));
#49106=CARTESIAN_POINT('Ctrl Pts',(17.1848333884845,2.31436759501462,9.123999830197));
#49107=CARTESIAN_POINT('Ctrl Pts',(18.1356179591903,-0.54561361705707,8.96699970284474));
#49108=CARTESIAN_POINT('Ctrl Pts',(16.274663824375,-2.9163378219851,8.80999957549249));
#49109=CARTESIAN_POINT('Ctrl Pts',(13.2707064095419,-2.67195394559781,8.65299944814023));
#49110=CARTESIAN_POINT('Ctrl Pts',(11.817423147442,-0.0316033214579261,
8.49599932078798));
#49111=CARTESIAN_POINT('Ctrl Pts',(13.2179870812285,2.63708629845826,8.33899919343572));
#49112=CARTESIAN_POINT('Ctrl Pts',(16.2164990952103,2.94107533850731,8.18199906608348));
#49113=CARTESIAN_POINT('Ctrl Pts',(18.1241646998305,0.607773905443812,8.02499893873121));
#49114=CARTESIAN_POINT('Ctrl Pts',(17.2303618464606,-2.27052421824958,7.86799881137898));
#49115=CARTESIAN_POINT('Ctrl Pts',(14.3365721278107,-3.11282149405098,7.71099868402671));
#49116=CARTESIAN_POINT('Ctrl Pts',(12.0376845476387,-1.16382187163074,7.55399855667447));
#49117=CARTESIAN_POINT('Ctrl Pts',(12.3951336511175,1.8287879857503,7.39699842932221));
#49118=CARTESIAN_POINT('Ctrl Pts',(15.088391402809,3.1815061164965,7.23999830196995));
#49119=CARTESIAN_POINT('Ctrl Pts',(17.7023877293502,1.68133718134365,7.0829981746177));
#49120=CARTESIAN_POINT('Ctrl Pts',(17.893127065655,-1.3265029163517,6.92599804726544));
#49121=CARTESIAN_POINT('Ctrl Pts',(15.4895715829936,-3.14485515809799,6.7689979199132));
#49122=CARTESIAN_POINT('Ctrl Pts',(12.6470126114897,-2.1431855409282,6.61199779256094));
#49123=CARTESIAN_POINT('Ctrl Pts',(11.9143999144365,0.780298978519449,6.45499766520869));
#49124=CARTESIAN_POINT('Ctrl Pts',(13.9486745921371,3.00408217741771,6.29799753785644));
#49125=CARTESIAN_POINT('Ctrl Pts',(16.9256825057651,2.53407556251617,6.14099741050418));
#49126=CARTESIAN_POINT('Ctrl Pts',(18.1759131113316,-0.208259934991238,
5.98399728315193));
#49127=CARTESIAN_POINT('Ctrl Pts',(16.5782706577155,-2.76384867084273,5.82699715579967));
#49128=CARTESIAN_POINT('Ctrl Pts',(13.5653803054279,-2.84106404628923,5.66999702844742));
#49129=CARTESIAN_POINT('Ctrl Pts',(11.8389222432929,-0.370677328850485,
5.51299690109516));
#49130=CARTESIAN_POINT('Ctrl Pts',(12.9470425851866,2.43211352025748,5.35599677374291));
#49131=CARTESIAN_POINT('Ctrl Pts',(15.8960507212661,3.05397713847976,5.19899664639066));
#49132=CARTESIAN_POINT('Ctrl Pts',(18.0415982494816,0.937364154516702,5.04199651903841));
#49133=CARTESIAN_POINT('Ctrl Pts',(17.459643977202,-2.01989749884988,4.88499639168616));
#49134=CARTESIAN_POINT('Ctrl Pts',(14.6722426504805,-3.16569257287314,4.7279962643339));
#49135=CARTESIAN_POINT('Ctrl Pts',(12.1784729871356,-1.4731805380298,4.57099613698165));
#49136=CARTESIAN_POINT('Ctrl Pts',(12.215322881631,1.54112605834992,4.41399600962939));
#49137=CARTESIAN_POINT('Ctrl Pts',(14.7481872905369,3.17196844909489,4.25699588227714));
#49138=CARTESIAN_POINT('Ctrl Pts',(17.5088738513129,1.96146864806794,4.09999575492489));
#49139=CARTESIAN_POINT('Ctrl Pts',(18.0158147471675,-1.0140076371251,3.94299562757263));
#49140=CARTESIAN_POINT('Ctrl Pts',(16.5566596891409,-2.38159377580301,3.83832887600446));
#49141=CARTESIAN_POINT('Ctrl Pts',(15.698066426161,-2.61113218593862,3.78599550022038));
#49142=CARTESIAN_POINT('Ctrl Pts',(17.1951971040191,1.87686343907872,12.2140044997796));
#49143=CARTESIAN_POINT('Ctrl Pts',(17.8123478989901,1.15503807360179,12.1616711239955));
#49144=CARTESIAN_POINT('Ctrl Pts',(18.2695195233736,-0.932473714789483,
12.0570043724274));
#49145=CARTESIAN_POINT('Ctrl Pts',(16.0220985187125,-3.24586736386177,11.9000042450751));
#49146=CARTESIAN_POINT('Ctrl Pts',(12.8583143384262,-2.6408513419267,11.7430041177229));
#49147=CARTESIAN_POINT('Ctrl Pts',(11.6149672212669,0.328384086517278,11.5860039903706));
#49148=CARTESIAN_POINT('Ctrl Pts',(13.4070235778454,3.00511912143942,11.4290038630183));
#49149=CARTESIAN_POINT('Ctrl Pts',(16.6275114271823,2.98612830149817,11.2720037356661));
#49150=CARTESIAN_POINT('Ctrl Pts',(18.3885970703671,0.289963978573797,11.1150036083139));
#49151=CARTESIAN_POINT('Ctrl Pts',(17.1110937259949,-2.66647876521353,10.9580034809616));
#49152=CARTESIAN_POINT('Ctrl Pts',(13.9405531465495,-3.23172848449065,10.8010033536093));
#49153=CARTESIAN_POINT('Ctrl Pts',(11.7200283335659,-0.899126013584159,
10.6440032262571));
#49154=CARTESIAN_POINT('Ctrl Pts',(12.4406857810575,2.23976716482285,10.4870030989048));
#49155=CARTESIAN_POINT('Ctrl Pts',(15.4563047387199,3.37022127835708,10.3300029715526));
#49156=CARTESIAN_POINT('Ctrl Pts',(18.0627509123809,1.47857505977427,10.1730028442003));
#49157=CARTESIAN_POINT('Ctrl Pts',(17.9227989331183,-1.73892843327666,10.0160027168481));
#49158=CARTESIAN_POINT('Ctrl Pts',(15.1619451243646,-3.39711563766634,9.85900258949583));
#49159=CARTESIAN_POINT('Ctrl Pts',(12.2558735618304,-2.00907793176401,9.70200246214356));
#49160=CARTESIAN_POINT('Ctrl Pts',(11.8104865060192,1.18051988264736,9.54500233479131));
#49161=CARTESIAN_POINT('Ctrl Pts',(14.2251667971895,3.31153385791409,9.38800220743906));
#49162=CARTESIAN_POINT('Ctrl Pts',(17.3346474556976,2.47306382524563,9.2310020800868));
#49163=CARTESIAN_POINT('Ctrl Pts',(18.3506273425917,-0.583026353208485,
9.07400195273456));
#49164=CARTESIAN_POINT('Ctrl Pts',(16.3620675471785,-3.11631116218659,8.91700182538229));
#49165=CARTESIAN_POINT('Ctrl Pts',(13.1521287149875,-2.85516987872383,8.76000169803006));
#49166=CARTESIAN_POINT('Ctrl Pts',(11.5991937918248,-0.0337703618144171,
8.60300157067778));
#49167=CARTESIAN_POINT('Ctrl Pts',(13.0957944213239,2.81791135635341,8.44600144332555));
#49168=CARTESIAN_POINT('Ctrl Pts',(16.2999144614232,3.1427449306896,8.28900131597327));
#49169=CARTESIAN_POINT('Ctrl Pts',(18.3383887330186,0.649448973758145,8.13200118862104));
#49170=CARTESIAN_POINT('Ctrl Pts',(17.3832978009075,-2.42621410729771,7.97500106126878));
#49171=CARTESIAN_POINT('Ctrl Pts',(14.2910808659327,-3.32626772340195,7.81800093391653));
#49172=CARTESIAN_POINT('Ctrl Pts',(11.8345585204434,-1.24362515961579,7.66100080656427));
#49173=CARTESIAN_POINT('Ctrl Pts',(12.2165179157807,1.95418801289184,7.50400067921202));
#49174=CARTESIAN_POINT('Ctrl Pts',(15.0944524029892,3.39966205172151,7.34700055185976));
#49175=CARTESIAN_POINT('Ctrl Pts',(17.8876905076099,1.7966265040084,7.19000042450751));
#49176=CARTESIAN_POINT('Ctrl Pts',(18.0915088438512,-1.41746124668302,7.03300029715526));
#49177=CARTESIAN_POINT('Ctrl Pts',(15.523141515798,-3.36049793640501,6.87600016980301));
#49178=CARTESIAN_POINT('Ctrl Pts',(12.4856682212804,-2.29014381443823,6.71900004245075));
#49179=CARTESIAN_POINT('Ctrl Pts',(11.7028202575859,0.833804094392522,6.5619999150985));
#49180=CARTESIAN_POINT('Ctrl Pts',(13.8765851888231,3.21007214974851,6.40499978774624));
#49181=CARTESIAN_POINT('Ctrl Pts',(17.0577265919963,2.70783717227864,6.247999660394));
#49182=CARTESIAN_POINT('Ctrl Pts',(18.3936855340856,-0.22254032271463,6.09099953304174));
#49183=CARTESIAN_POINT('Ctrl Pts',(16.6864927068848,-2.95336582703543,5.93399940568949));
#49184=CARTESIAN_POINT('Ctrl Pts',(13.4670084055473,-3.03587586225233,5.77699927833723));
#49185=CARTESIAN_POINT('Ctrl Pts',(11.6221670810891,-0.396094680375534,
5.61999915098498));
#49186=CARTESIAN_POINT('Ctrl Pts',(12.806271256009,2.59888359083319,5.46299902363272));
#49187=CARTESIAN_POINT('Ctrl Pts',(15.957492936352,3.26338840924436,5.30599889628048));
#49188=CARTESIAN_POINT('Ctrl Pts',(18.250160699591,1.00163923251032,5.14899876892821));
#49189=CARTESIAN_POINT('Ctrl Pts',(17.6283018117366,-2.15840190895786,4.99199864157597));
#49190=CARTESIAN_POINT('Ctrl Pts',(14.6497683227587,-3.38276417310961,4.8349985142237));
#49191=CARTESIAN_POINT('Ctrl Pts',(11.9850008259279,-1.57419655568344,4.67799838687146));
#49192=CARTESIAN_POINT('Ctrl Pts',(12.0243775183933,1.64680110163074,4.5209982595192));
#49193=CARTESIAN_POINT('Ctrl Pts',(14.7309204882355,3.38947038628386,4.36399813216696));
#49194=CARTESIAN_POINT('Ctrl Pts',(17.6809073792564,2.09596659076089,4.20699800481469));
#49195=CARTESIAN_POINT('Ctrl Pts',(18.2226092220303,-1.08353816018628,4.04999787746244));
#49196=CARTESIAN_POINT('Ctrl Pts',(16.663399873782,-2.54489970653575,3.94533112589427));
#49197=CARTESIAN_POINT('Ctrl Pts',(15.7459328543469,-2.79017756984216,3.89299775011019));
#49198=CARTESIAN_POINT('Ctrl Pts',(17.3360626576962,1.99730155693062,12.3210067496694));
#49199=CARTESIAN_POINT('Ctrl Pts',(17.9928159504458,1.22915673814361,12.2686733738853));
#49200=CARTESIAN_POINT('Ctrl Pts',(18.4793242270491,-0.9923104492142,12.1640066223172));
#49201=CARTESIAN_POINT('Ctrl Pts',(16.087686466823,-3.45415431109555,12.0070064949649));
#49202=CARTESIAN_POINT('Ctrl Pts',(12.7208826080511,-2.81031447841596,11.8500063676127));
#49203=CARTESIAN_POINT('Ctrl Pts',(11.3977500448602,0.349456456775644,11.6930062402604));
#49204=CARTESIAN_POINT('Ctrl Pts',(13.3048024582519,3.19795728077006,11.5360061129082));
#49205=CARTESIAN_POINT('Ctrl Pts',(16.7319486542021,3.17774782202826,11.3790059855559));
#49206=CARTESIAN_POINT('Ctrl Pts',(18.606042966971,0.308570934784431,11.2220058582037));
#49207=CARTESIAN_POINT('Ctrl Pts',(17.246562375271,-2.83758641060089,11.0650057308514));
#49208=CARTESIAN_POINT('Ctrl Pts',(13.8725685599584,-3.4391081414099,10.9080056034992));
#49209=CARTESIAN_POINT('Ctrl Pts',(11.5095529170344,-0.956822829736598,
10.7510054761469));
#49210=CARTESIAN_POINT('Ctrl Pts',(12.276454872669,2.38349277433771,10.5940053487947));
#49211=CARTESIAN_POINT('Ctrl Pts',(15.4855857629831,3.58648800243424,10.4370052214424));
#49212=CARTESIAN_POINT('Ctrl Pts',(18.2592872973176,1.57345505668517,10.2800050940901));
#49213=CARTESIAN_POINT('Ctrl Pts',(18.1103546151327,-1.85051527716861,10.1230049667379));
#49214=CARTESIAN_POINT('Ctrl Pts',(15.1723371249586,-3.61510816978504,9.96600483938563));
#49215=CARTESIAN_POINT('Ctrl Pts',(12.0797832739173,-2.13800023888626,9.80900471203338));
#49216=CARTESIAN_POINT('Ctrl Pts',(11.6058157803393,1.25627371203762,9.65200458468112));
#49217=CARTESIAN_POINT('Ctrl Pts',(14.1754458368614,3.52403461675767,9.49500445732887));
#49218=CARTESIAN_POINT('Ctrl Pts',(17.4844615229107,2.63176005547664,9.33800432997661));
#49219=CARTESIAN_POINT('Ctrl Pts',(18.565636725993,-0.620439089359897,9.18100420262437));
#49220=CARTESIAN_POINT('Ctrl Pts',(16.4494712699821,-3.31628450238807,9.0240040752721));
#49221=CARTESIAN_POINT('Ctrl Pts',(13.033551020433,-3.03838581184986,8.86700394791986));
#49222=CARTESIAN_POINT('Ctrl Pts',(11.3809644362075,-0.0359374021709085,
8.7100038205676));
#49223=CARTESIAN_POINT('Ctrl Pts',(12.9736017614192,2.99873641424856,8.55300369321535));
#49224=CARTESIAN_POINT('Ctrl Pts',(16.383329827636,3.34441452287188,8.39600356586309));
#49225=CARTESIAN_POINT('Ctrl Pts',(18.5526127662067,0.691124042072478,8.23900343851084));
#49226=CARTESIAN_POINT('Ctrl Pts',(17.5362337553543,-2.58190399634584,8.08200331115859));
#49227=CARTESIAN_POINT('Ctrl Pts',(14.2455896040548,-3.53971395275292,7.92500318380633));
#49228=CARTESIAN_POINT('Ctrl Pts',(11.6314324932481,-1.32342844760082,7.76800305645409));
#49229=CARTESIAN_POINT('Ctrl Pts',(12.0379021804438,2.07958804003338,7.61100292910183));
#49230=CARTESIAN_POINT('Ctrl Pts',(15.1005134031695,3.61781798694653,7.45400280174957));
#49231=CARTESIAN_POINT('Ctrl Pts',(18.0729932858696,1.91191582667314,7.29700267439733));
#49232=CARTESIAN_POINT('Ctrl Pts',(18.2898906220475,-1.50841957701434,7.14000254704506));
#49233=CARTESIAN_POINT('Ctrl Pts',(15.5567114486024,-3.57614071471203,6.98300241969282));
#49234=CARTESIAN_POINT('Ctrl Pts',(12.3243238310711,-2.43710208794826,6.82600229234056));
#49235=CARTESIAN_POINT('Ctrl Pts',(11.4912406007353,0.887309210265594,6.66900216498831));
#49236=CARTESIAN_POINT('Ctrl Pts',(13.8044957855091,3.41606212207931,6.51200203763605));
#49237=CARTESIAN_POINT('Ctrl Pts',(17.1897706782275,2.88159878204111,6.35500191028381));
#49238=CARTESIAN_POINT('Ctrl Pts',(18.6114579568395,-0.236820710438023,
6.19800178293155));
#49239=CARTESIAN_POINT('Ctrl Pts',(16.7947147560542,-3.14288298322814,6.04100165557929));
#49240=CARTESIAN_POINT('Ctrl Pts',(13.3686365056666,-3.23068767821543,5.88400152822705));
#49241=CARTESIAN_POINT('Ctrl Pts',(11.4054119188853,-0.421512031900586,
5.72700140087479));
#49242=CARTESIAN_POINT('Ctrl Pts',(12.6654999268314,2.7656536614089,5.57000127352253));
#49243=CARTESIAN_POINT('Ctrl Pts',(16.0189351514379,3.47279968000896,5.41300114617029));
#49244=CARTESIAN_POINT('Ctrl Pts',(18.4587231497003,1.06591431050395,5.25600101881802));
#49245=CARTESIAN_POINT('Ctrl Pts',(17.7969596462713,-2.29690631906584,5.09900089146578));
#49246=CARTESIAN_POINT('Ctrl Pts',(14.6272939950368,-3.59983577334609,4.94200076411352));
#49247=CARTESIAN_POINT('Ctrl Pts',(11.7915286647202,-1.67521257333708,4.78500063676127));
#49248=CARTESIAN_POINT('Ctrl Pts',(11.8334321551556,1.75247614491157,4.62800050940901));
#49249=CARTESIAN_POINT('Ctrl Pts',(14.713653685934,3.60697232347283,4.47100038205677));
#49250=CARTESIAN_POINT('Ctrl Pts',(17.8529409071999,2.23046453345384,4.3140002547045));
#49251=CARTESIAN_POINT('Ctrl Pts',(18.4294036968932,-1.15306868324745,4.15700012735226));
#49252=CARTESIAN_POINT('Ctrl Pts',(16.7701400584231,-2.7082056372685,4.05233337578409));
#49253=CARTESIAN_POINT('Ctrl Pts',(15.7937992825329,-2.9692229537457,4.));
#49254=CARTESIAN_POINT('Ctrl Pts',(16.9134659966651,1.63598720337493,12.));
#49255=CARTESIAN_POINT('Ctrl Pts',(16.9751046175812,1.57806203522303,12.));
#49256=CARTESIAN_POINT('Ctrl Pts',(17.0333781400082,1.51698823254714,12.));
#49257=CARTESIAN_POINT('Ctrl Pts',(17.0882869575319,1.45315007481724,12.));
#49258=CARTESIAN_POINT('Ctrl Pts',(17.144646063235,1.38762578124011,12.));
#49259=CARTESIAN_POINT('Ctrl Pts',(17.1974608152615,1.31918874417436,12.));
#49260=CARTESIAN_POINT('Ctrl Pts',(17.246706209466,1.24820595309377,12.));
#49261=CARTESIAN_POINT('Ctrl Pts',(17.2968789923958,1.17588641486748,12.));
#49262=CARTESIAN_POINT('Ctrl Pts',(17.3433471915708,1.10092373974675,12.));
#49263=CARTESIAN_POINT('Ctrl Pts',(17.3860513180704,1.02366428011772,12.));
#49264=CARTESIAN_POINT('Ctrl Pts',(17.4053930048836,0.988671683523578,12.));
#49265=CARTESIAN_POINT('Ctrl Pts',(17.4239620441889,0.953207420756028,12.));
#49266=CARTESIAN_POINT('Ctrl Pts',(17.4417503295423,0.917301461090561,12.));
#49267=CARTESIAN_POINT('Ctrl Pts',(17.4518550628932,0.896904883178727,12.));
#49268=CARTESIAN_POINT('Ctrl Pts',(17.4617078263978,0.876365752925188,12.));
#49269=CARTESIAN_POINT('Ctrl Pts',(17.4713068826732,0.855689404786285,12.));
#49270=CARTESIAN_POINT('Ctrl Pts',(17.4795241183999,0.837989495363037,12.));
#49271=CARTESIAN_POINT('Ctrl Pts',(17.4875575606575,0.820183889043797,12.));
#49272=CARTESIAN_POINT('Ctrl Pts',(17.4953933345483,0.802305631697034,12.));
#49273=CARTESIAN_POINT('Ctrl Pts',(17.5320009593848,0.718780947752926,12.));
#49274=CARTESIAN_POINT('Ctrl Pts',(17.5643466650844,0.633572893252199,12.));
#49275=CARTESIAN_POINT('Ctrl Pts',(17.5924032599934,0.547079296293481,12.));
#49276=CARTESIAN_POINT('Ctrl Pts',(17.6209190605514,0.45917004827483,12.));
#49277=CARTESIAN_POINT('Ctrl Pts',(17.6450046970528,0.369932078122487,12.));
#49278=CARTESIAN_POINT('Ctrl Pts',(17.6645925974806,0.27974597155399,12.));
#49279=CARTESIAN_POINT('Ctrl Pts',(17.6832979692358,0.193623180766213,12.));
#49280=CARTESIAN_POINT('Ctrl Pts',(17.6979018128389,0.106634841931331,12.));
#49281=CARTESIAN_POINT('Ctrl Pts',(17.7083066964275,0.0190916104279826,
12.));
#49282=CARTESIAN_POINT('Ctrl Pts',(17.7128967523775,-0.0195275944118574,
12.));
#49283=CARTESIAN_POINT('Ctrl Pts',(17.7166691326112,-0.0582549851430788,
12.));
#49284=CARTESIAN_POINT('Ctrl Pts',(17.7196128778618,-0.0970645844891166,
12.));
#49285=CARTESIAN_POINT('Ctrl Pts',(17.720985220376,-0.115157204130783,12.));
#49286=CARTESIAN_POINT('Ctrl Pts',(17.7221774501012,-0.13326769426837,12.));
#49287=CARTESIAN_POINT('Ctrl Pts',(17.7231883308136,-0.151393437782305,
12.));
#49288=CARTESIAN_POINT('Ctrl Pts',(17.724162595519,-0.168862632662539,12.));
#49289=CARTESIAN_POINT('Ctrl Pts',(17.7249684090533,-0.186348823197974,
12.));
#49290=CARTESIAN_POINT('Ctrl Pts',(17.7256040109254,-0.203825085573831,
12.));
#49291=CARTESIAN_POINT('Ctrl Pts',(17.7290683171088,-0.299078303780242,
12.));
#49292=CARTESIAN_POINT('Ctrl Pts',(17.7274898676139,-0.394183686637061,
12.));
#49293=CARTESIAN_POINT('Ctrl Pts',(17.7208064378308,-0.488742644592356,
12.));
#49294=CARTESIAN_POINT('Ctrl Pts',(17.71415791669,-0.582807705707687,12.));
#49295=CARTESIAN_POINT('Ctrl Pts',(17.7024579548962,-0.676332990245415,
12.));
#49296=CARTESIAN_POINT('Ctrl Pts',(17.6855973100545,-0.768943912339204,
12.));
#49297=CARTESIAN_POINT('Ctrl Pts',(17.6690987547922,-0.859565975160523,
12.));
#49298=CARTESIAN_POINT('Ctrl Pts',(17.6476591367551,-0.949313458601225,
12.));
#49299=CARTESIAN_POINT('Ctrl Pts',(17.6215530748909,-1.03794459575461,12.));
#49300=CARTESIAN_POINT('Ctrl Pts',(17.6062284518588,-1.08997231149527,12.));
#49301=CARTESIAN_POINT('Ctrl Pts',(17.5892948213721,-1.14161533429799,12.));
#49302=CARTESIAN_POINT('Ctrl Pts',(17.5707996132467,-1.19282361176805,12.));
#49303=CARTESIAN_POINT('Ctrl Pts',(17.5660385338913,-1.20600576527691,12.));
#49304=CARTESIAN_POINT('Ctrl Pts',(17.5611731178881,-1.21916127939291,12.));
#49305=CARTESIAN_POINT('Ctrl Pts',(17.5562068240413,-1.23228215182306,12.));
#49306=CARTESIAN_POINT('Ctrl Pts',(17.5231582789659,-1.31959590274395,12.));
#49307=CARTESIAN_POINT('Ctrl Pts',(17.4857269461903,-1.40516846103908,12.));
#49308=CARTESIAN_POINT('Ctrl Pts',(17.4442438276358,-1.48876399852657,12.));
#49309=CARTESIAN_POINT('Ctrl Pts',(17.4011939593262,-1.57551680317371,12.));
#49310=CARTESIAN_POINT('Ctrl Pts',(17.3537803586004,-1.6601411473433,12.));
#49311=CARTESIAN_POINT('Ctrl Pts',(17.302316868041,-1.74237153203792,12.));
#49312=CARTESIAN_POINT('Ctrl Pts',(17.2502282381553,-1.82560078887907,12.));
#49313=CARTESIAN_POINT('Ctrl Pts',(17.1939903374979,-1.90637839472423,12.));
#49314=CARTESIAN_POINT('Ctrl Pts',(17.133876364298,-1.98441530832993,12.));
#49315=CARTESIAN_POINT('Ctrl Pts',(17.0944014617075,-2.03565962639887,12.));
#49316=CARTESIAN_POINT('Ctrl Pts',(17.0532540884055,-2.08572182092047,12.));
#49317=CARTESIAN_POINT('Ctrl Pts',(17.0105008848643,-2.13451422415292,12.));
#49318=CARTESIAN_POINT('Ctrl Pts',(16.9990423392555,-2.14759137233113,12.));
#49319=CARTESIAN_POINT('Ctrl Pts',(16.9874683992165,-2.16057727630897,12.));
#49320=CARTESIAN_POINT('Ctrl Pts',(16.9757802548447,-2.17347017426791,12.));
#49321=CARTESIAN_POINT('Ctrl Pts',(16.9646250327531,-2.18577521906894,12.));
#49322=CARTESIAN_POINT('Ctrl Pts',(16.953371454143,-2.19798925370335,12.));
#49323=CARTESIAN_POINT('Ctrl Pts',(16.942023959817,-2.2101077517839,12.));
#49324=CARTESIAN_POINT('Ctrl Pts',(16.8702005619852,-2.28681117932109,12.));
#49325=CARTESIAN_POINT('Ctrl Pts',(16.7945813632066,-2.35973107336475,12.));
#49326=CARTESIAN_POINT('Ctrl Pts',(16.7155099454751,-2.42853427108366,12.));
#49327=CARTESIAN_POINT('Ctrl Pts',(16.6562063821765,-2.48013666937285,12.));
#49328=CARTESIAN_POINT('Ctrl Pts',(16.5949596324728,-2.52942316838901,12.));
#49329=CARTESIAN_POINT('Ctrl Pts',(16.5318955908763,-2.57624166180053,12.));
#49330=CARTESIAN_POINT('Ctrl Pts',(16.509253132243,-2.59305133294597,12.));
#49331=CARTESIAN_POINT('Ctrl Pts',(16.4863762692883,-2.60954274193113,12.));
#49332=CARTESIAN_POINT('Ctrl Pts',(16.4632703841368,-2.62570843265804,12.));
#49333=CARTESIAN_POINT('Ctrl Pts',(16.4439550552025,-2.63922211680365,12.));
#49334=CARTESIAN_POINT('Ctrl Pts',(16.4244771453842,-2.65250971655999,12.));
#49335=CARTESIAN_POINT('Ctrl Pts',(16.4048604457735,-2.66555338685653,12.));
#49336=CARTESIAN_POINT('Ctrl Pts',(16.3198883986288,-2.72205358257614,12.));
#49337=CARTESIAN_POINT('Ctrl Pts',(16.2322397460524,-2.7740341002851,12.));
#49338=CARTESIAN_POINT('Ctrl Pts',(16.1422018474634,-2.82118285115376,12.));
#49339=CARTESIAN_POINT('Ctrl Pts',(16.0701250286698,-2.85892620174232,12.));
#49340=CARTESIAN_POINT('Ctrl Pts',(15.9965161480314,-2.89357290485328,12.));
#49341=CARTESIAN_POINT('Ctrl Pts',(15.9215058272316,-2.92494553699154,12.));
#49342=CARTESIAN_POINT('Ctrl Pts',(15.8800022019638,-2.94230418782848,12.));
#49343=CARTESIAN_POINT('Ctrl Pts',(15.8380692864041,-2.95866019100725,12.));
#49344=CARTESIAN_POINT('Ctrl Pts',(15.795740524146,-2.97402278592473,12.));
#49345=CARTESIAN_POINT('Ctrl Pts',(12.4833920687165,-0.00213593309729046,
10.387416697508));
#49346=CARTESIAN_POINT('Ctrl Pts',(12.4814996767346,-0.226800666605093,
10.4016107071645));
#49347=CARTESIAN_POINT('Ctrl Pts',(12.5091661046464,-0.451007239373056,
10.415804716821));
#49348=CARTESIAN_POINT('Ctrl Pts',(12.5682644306803,-0.666597124996037,
10.4299987264775));
#49349=CARTESIAN_POINT('Ctrl Pts',(12.7861602176632,-1.46147797773692,10.4823321022615));
#49350=CARTESIAN_POINT('Ctrl Pts',(13.4313412686974,-2.13922357419454,10.5346654780456));
#49351=CARTESIAN_POINT('Ctrl Pts',(14.2145374788331,-2.39597875638779,10.5869988538297));
#49352=CARTESIAN_POINT('Ctrl Pts',(14.9977336889687,-2.65273393858105,10.6393322296138));
#49353=CARTESIAN_POINT('Ctrl Pts',(15.9189450582056,-2.48849870650994,10.6916656053979));
#49354=CARTESIAN_POINT('Ctrl Pts',(16.5651422177769,-1.97687883370916,10.743998981182));
#49355=CARTESIAN_POINT('Ctrl Pts',(17.2113393773482,-1.46525896090837,10.7963323569661));
#49356=CARTESIAN_POINT('Ctrl Pts',(17.5825223272538,-0.60625444737792,10.8486657327501));
#49357=CARTESIAN_POINT('Ctrl Pts',(17.5122690848705,0.214937675101548,10.9009991085342));
#49358=CARTESIAN_POINT('Ctrl Pts',(17.4420158424871,1.03612979758102,10.9533324843183));
#49359=CARTESIAN_POINT('Ctrl Pts',(16.9303264078149,1.8195095290095,11.0056658601024));
#49360=CARTESIAN_POINT('Ctrl Pts',(16.206619831127,2.2139583184471,11.0579992358865));
#49361=CARTESIAN_POINT('Ctrl Pts',(15.4829132544392,2.60840710788471,11.1103326116706));
#49362=CARTESIAN_POINT('Ctrl Pts',(14.5471895357358,2.61392495533142,11.1626659874547));
#49363=CARTESIAN_POINT('Ctrl Pts',(13.8189836358921,2.22781663625852,11.2149993632387));
#49364=CARTESIAN_POINT('Ctrl Pts',(13.0907777360484,1.84170831718561,11.2673327390228));
#49365=CARTESIAN_POINT('Ctrl Pts',(12.5700896550643,1.06397383159308,11.3196661148069));
#49366=CARTESIAN_POINT('Ctrl Pts',(12.4903749854216,0.243745852972027,11.371999490591));
#49367=CARTESIAN_POINT('Ctrl Pts',(12.4825471092477,0.163200539545801,11.3771385595633));
#49368=CARTESIAN_POINT('Ctrl Pts',(12.4789715321031,0.0822454620963692,
11.3822776285357));
#49369=CARTESIAN_POINT('Ctrl Pts',(12.4794948718273,0.00124609658704006,
11.387416697508));
#49370=CARTESIAN_POINT('Ctrl Pts',(14.2062007174671,-2.96922295374568,12.));
#49371=CARTESIAN_POINT('Ctrl Pts',(13.2298599415769,-2.70820563726846,11.9476666242159));
#49372=CARTESIAN_POINT('Ctrl Pts',(11.5705939465555,-1.15308308242658,11.8429998726477));
#49373=CARTESIAN_POINT('Ctrl Pts',(12.1470611574329,2.23047193499529,11.6859997452955));
#49374=CARTESIAN_POINT('Ctrl Pts',(15.2863460006058,3.60696666543133,11.5289996179432));
#49375=CARTESIAN_POINT('Ctrl Pts',(18.1665668486981,1.75247841941832,11.371999490591));
#49376=CARTESIAN_POINT('Ctrl Pts',(18.2084706556688,-1.6752137223659,11.2149993632387));
#49377=CARTESIAN_POINT('Ctrl Pts',(15.3727057323674,-3.59983386165072,11.0579992358865));
#49378=CARTESIAN_POINT('Ctrl Pts',(12.2030412422492,-2.29690621757914,10.9009991085342));
#49379=CARTESIAN_POINT('Ctrl Pts',(11.5412777161188,1.06591431606771,10.743998981182));
#49380=CARTESIAN_POINT('Ctrl Pts',(13.9810651784412,3.47279856287599,10.5869988538297));
#49381=CARTESIAN_POINT('Ctrl Pts',(17.3344994031312,2.76565299665532,10.4299987264775));
#49382=CARTESIAN_POINT('Ctrl Pts',(18.5945871152999,-0.421511967551375,
10.2729985991252));
#49383=CARTESIAN_POINT('Ctrl Pts',(16.6313630370479,-3.23068676566348,10.115998471773));
#49384=CARTESIAN_POINT('Ctrl Pts',(13.205285741413,-3.14288213812672,9.9589983444207));
#49385=CARTESIAN_POINT('Ctrl Pts',(11.388543028433,-0.236820637232293,9.80199821706845));
#49386=CARTESIAN_POINT('Ctrl Pts',(12.8102299232355,2.88159798857394,9.6449980897162));
#49387=CARTESIAN_POINT('Ctrl Pts',(16.1955038860992,3.41606118929613,9.48799796236394));
#49388=CARTESIAN_POINT('Ctrl Pts',(18.5087584392439,0.887308966009096,9.3309978350117));
#49389=CARTESIAN_POINT('Ctrl Pts',(17.6756754360527,-2.43710142000481,9.17399770765943));
#49390=CARTESIAN_POINT('Ctrl Pts',(14.4432887039958,-3.57613973602564,9.0169975803072));
#49391=CARTESIAN_POINT('Ctrl Pts',(11.7101102785552,-1.50841916383422,8.85999745295492));
#49392=CARTESIAN_POINT('Ctrl Pts',(11.9270075555053,1.91191530312036,8.70299732560268));
#49393=CARTESIAN_POINT('Ctrl Pts',(14.8994866243195,3.61781699652394,8.54599719825042));
#49394=CARTESIAN_POINT('Ctrl Pts',(17.9620970086125,2.07958747065415,8.38899707089818));
#49395=CARTESIAN_POINT('Ctrl Pts',(18.3685665845007,-1.32342808525659,8.23199694354591));
#49396=CARTESIAN_POINT('Ctrl Pts',(15.7544101894084,-3.53971298366467,8.07499681619367));
#49397=CARTESIAN_POINT('Ctrl Pts',(12.4637669390099,-2.58190328946754,7.91799668884141));
#49398=CARTESIAN_POINT('Ctrl Pts',(11.4473882064255,0.691123852849571,7.76099656148916));
#49399=CARTESIAN_POINT('Ctrl Pts',(13.6166705510885,3.34441360725337,7.60399643413689));
#49400=CARTESIAN_POINT('Ctrl Pts',(17.0263976837988,2.99873559323853,7.44699630678466));
#49401=CARTESIAN_POINT('Ctrl Pts',(18.6190345729722,-0.0359373922966709,
7.2899961794324));
#49402=CARTESIAN_POINT('Ctrl Pts',(16.9664484412042,-3.03838498006983,7.13299605208014));
#49403=CARTESIAN_POINT('Ctrl Pts',(13.5505291268344,-3.3162835943375,6.97599592472789));
#49404=CARTESIAN_POINT('Ctrl Pts',(11.4343642502377,-0.620438919723572,
6.81899579737564));
#49405=CARTESIAN_POINT('Ctrl Pts',(12.5155391572145,2.63175933537736,6.66199567002338));
#49406=CARTESIAN_POINT('Ctrl Pts',(15.824553937525,3.52403365117268,6.50499554267113));
#49407=CARTESIAN_POINT('Ctrl Pts',(18.3941832901488,1.25627336953411,6.34799541531888));
#49408=CARTESIAN_POINT('Ctrl Pts',(17.9202159270872,-2.13799965619268,6.19099528796662));
#49409=CARTESIAN_POINT('Ctrl Pts',(14.8276629212552,-3.61510717519363,6.03399516061437));
#49410=CARTESIAN_POINT('Ctrl Pts',(11.889646238299,-1.85051477939823,5.87699503326212));
#49411=CARTESIAN_POINT('Ctrl Pts',(11.7407135913467,1.57345464202167,5.71999490590987));
#49412=CARTESIAN_POINT('Ctrl Pts',(14.5144143770745,3.58648699137295,5.56299477855761));
#49413=CARTESIAN_POINT('Ctrl Pts',(17.7235443678513,2.3834921742297,5.40599465120536));
#49414=CARTESIAN_POINT('Ctrl Pts',(18.4904461542425,-0.956822661448993,
5.2489945238531));
#49415=CARTESIAN_POINT('Ctrl Pts',(16.1274310791049,-3.43910703392132,5.09199439650085));
#49416=CARTESIAN_POINT('Ctrl Pts',(12.7534383414036,-2.83758592474999,4.9349942691486));
#49417=CARTESIAN_POINT('Ctrl Pts',(11.3939578227468,0.308571354444121,4.77799414179634));
#49418=CARTESIAN_POINT('Ctrl Pts',(13.2680522040149,3.17774609218688,4.62099401444409));
#49419=CARTESIAN_POINT('Ctrl Pts',(16.6951963308219,3.19795784272698,4.46399388709183));
#49420=CARTESIAN_POINT('Ctrl Pts',(18.6022504225887,0.349454018091392,4.30699375973959));
#49421=CARTESIAN_POINT('Ctrl Pts',(17.2791139286761,-2.8103099931699,4.14999363238733));
#49422=CARTESIAN_POINT('Ctrl Pts',(13.9123194271849,-3.45415924122653,3.99299350503508));
#49423=CARTESIAN_POINT('Ctrl Pts',(11.5206656746196,-0.992299917670973,
3.83599337768282));
#49424=CARTESIAN_POINT('Ctrl Pts',(12.0071840495542,1.22915673814367,3.73132662611465));
#49425=CARTESIAN_POINT('Ctrl Pts',(12.6639373423039,1.99730155693067,3.67899325033057));
#49426=CARTESIAN_POINT('Ctrl Pts',(14.254067145653,-2.79017756984214,12.1070022498898));
#49427=CARTESIAN_POINT('Ctrl Pts',(13.336600126218,-2.54489970653572,12.0546688741057));
#49428=CARTESIAN_POINT('Ctrl Pts',(11.7773885635194,-1.08355169108889,11.9500021225376));
#49429=CARTESIAN_POINT('Ctrl Pts',(12.3190945608781,2.0959735459863,11.7930019951853));
#49430=CARTESIAN_POINT('Ctrl Pts',(15.2690792172061,3.38946506942463,11.636001867833));
#49431=CARTESIAN_POINT('Ctrl Pts',(17.9756215455284,1.64680323898379,11.4790017404808));
#49432=CARTESIAN_POINT('Ctrl Pts',(18.014998535442,-1.57419763542533,11.3220016131285));
#49433=CARTESIAN_POINT('Ctrl Pts',(15.3502314210832,-3.38276237669027,11.1650014857763));
#49434=CARTESIAN_POINT('Ctrl Pts',(12.3716990232057,-2.15840181359085,11.008001358424));
#49435=CARTESIAN_POINT('Ctrl Pts',(11.7498401140189,1.00163923773859,10.8510012310718));
#49436=CARTESIAN_POINT('Ctrl Pts',(14.0425073736352,3.26338735947497,10.6940011037195));
#49437=CARTESIAN_POINT('Ctrl Pts',(17.1937281143572,2.59888296616453,10.5370009763673));
#49438=CARTESIAN_POINT('Ctrl Pts',(18.3778320113351,-0.396094619906611,
10.380000849015));
#49439=CARTESIAN_POINT('Ctrl Pts',(16.5329911647418,-3.03587500472764,10.2230007216628));
#49440=CARTESIAN_POINT('Ctrl Pts',(13.3135077605849,-2.95336503289398,10.0660005943105));
#49441=CARTESIAN_POINT('Ctrl Pts',(11.6063153917746,-0.222540253923235,
9.90900046695825));
#49442=CARTESIAN_POINT('Ctrl Pts',(12.9422739731982,2.70783642665787,9.75200033960602));
#49443=CARTESIAN_POINT('Ctrl Pts',(16.1234145025873,3.21007127321255,9.59500021225374));
#49444=CARTESIAN_POINT('Ctrl Pts',(18.297178840283,0.83380386486479,9.43800008490151));
#49445=CARTESIAN_POINT('Ctrl Pts',(17.5143310900362,-2.29014318677205,9.28099995754924));
#49446=CARTESIAN_POINT('Ctrl Pts',(14.4768586275985,-3.36049701673381,9.12399983019701));
#49447=CARTESIAN_POINT('Ctrl Pts',(11.9084920024447,-1.41746085841783,8.96699970284473));
#49448=CARTESIAN_POINT('Ctrl Pts',(12.1123102830297,1.79662601202607,8.8099995754925));
#49449=CARTESIAN_POINT('Ctrl Pts',(14.9055476228422,3.39966112102182,8.65299944814023));
#49450=CARTESIAN_POINT('Ctrl Pts',(17.7834813221759,1.95418747784641,8.49599932078799));
#49451=CARTESIAN_POINT('Ctrl Pts',(18.1654406129175,-1.24362481912106,8.33899919343572));
#49452=CARTESIAN_POINT('Ctrl Pts',(15.7089189399847,-3.32626681275013,8.18199906608348));
#49453=CARTESIAN_POINT('Ctrl Pts',(12.6167028515863,-2.42621344304447,8.02499893873122));
#49454=CARTESIAN_POINT('Ctrl Pts',(11.6616121809635,0.649448795945457,7.86799881137897));
#49455=CARTESIAN_POINT('Ctrl Pts',(13.7000858944641,3.14274407028327,7.71099868402671));
#49456=CARTESIAN_POINT('Ctrl Pts',(16.9042050573477,2.81791058485063,7.55399855667447));
#49457=CARTESIAN_POINT('Ctrl Pts',(18.4008052771018,-0.033770352535599,
7.3969984293222));
#49458=CARTESIAN_POINT('Ctrl Pts',(16.8478707791132,-2.85516909710049,7.23999830196996));
#49459=CARTESIAN_POINT('Ctrl Pts',(13.6379328257098,-3.11631030889185,7.08299817461769));
#49460=CARTESIAN_POINT('Ctrl Pts',(11.6493735747719,-0.583026193801301,
6.92599804726545));
#49461=CARTESIAN_POINT('Ctrl Pts',(12.6653531834158,2.47306314856864,6.76899791991319));
#49462=CARTESIAN_POINT('Ctrl Pts',(15.7748329908015,3.31153295055427,6.61199779256095));
#49463=CARTESIAN_POINT('Ctrl Pts',(18.1895126205188,1.18051956079695,6.45499766520868));
#49464=CARTESIAN_POINT('Ctrl Pts',(17.7441256873539,-2.00907738420709,6.29799753785643));
#49465=CARTESIAN_POINT('Ctrl Pts',(14.8380549190625,-3.39711470304921,6.14099741050418));
#49466=CARTESIAN_POINT('Ctrl Pts',(12.0772018688511,-1.73892796552204,5.98399728315193));
#49467=CARTESIAN_POINT('Ctrl Pts',(11.9372499226966,1.47857467011516,5.82699715579967));
#49468=CARTESIAN_POINT('Ctrl Pts',(14.5436953928922,3.3702203282632,5.66999702844742));
#49469=CARTESIAN_POINT('Ctrl Pts',(17.5593135052598,2.2397666009016,5.51299690109516));
#49470=CARTESIAN_POINT('Ctrl Pts',(18.2799707937134,-0.89912585544437,5.35599677374292));
#49471=CARTESIAN_POINT('Ctrl Pts',(16.0594465142784,-3.23172744378409,5.19899664639066));
#49472=CARTESIAN_POINT('Ctrl Pts',(12.888906947464,-2.66647830865965,5.04199651903841));
#49473=CARTESIAN_POINT('Ctrl Pts',(11.6114036717303,0.289964372927834,4.88499639168615));
#49474=CARTESIAN_POINT('Ctrl Pts',(13.3724893792839,2.98612667596695,4.72799626433391));
#49475=CARTESIAN_POINT('Ctrl Pts',(16.5929752842478,3.0051196495101,4.57099613698165));
#49476=CARTESIAN_POINT('Ctrl Pts',(18.3850332179946,0.328381794886706,4.41399600962939));
#49477=CARTESIAN_POINT('Ctrl Pts',(17.1416824071377,-2.64084712714285,4.25699588227714));
#49478=CARTESIAN_POINT('Ctrl Pts',(13.9779070198844,-3.24587199670379,4.09999575492489));
#49479=CARTESIAN_POINT('Ctrl Pts',(11.7304709872286,-0.932463818302713,
3.94299562757263));
#49480=CARTESIAN_POINT('Ctrl Pts',(12.1876521010099,1.15503807360185,3.83832887600446));
#49481=CARTESIAN_POINT('Ctrl Pts',(12.8048028959809,1.87686343907877,3.78599550022038));
#49482=CARTESIAN_POINT('Ctrl Pts',(14.3019335738389,-2.6111321859386,12.2140044997796));
#49483=CARTESIAN_POINT('Ctrl Pts',(13.4433403108591,-2.38159377580297,12.1616711239955));
#49484=CARTESIAN_POINT('Ctrl Pts',(11.9841831804832,-1.0140202997512,12.0570043724274));
#49485=CARTESIAN_POINT('Ctrl Pts',(12.4911279643235,1.96147515697731,11.9000042450751));
#49486=CARTESIAN_POINT('Ctrl Pts',(15.2518124338064,3.17196347341793,11.7430041177229));
#49487=CARTESIAN_POINT('Ctrl Pts',(17.7846762423587,1.54112805854926,11.5860039903706));
#49488=CARTESIAN_POINT('Ctrl Pts',(17.8215264152151,-1.47318154848477,11.4290038630184));
#49489=CARTESIAN_POINT('Ctrl Pts',(15.3277571097989,-3.16569089172983,11.2720037356661));
#49490=CARTESIAN_POINT('Ctrl Pts',(12.5403568041622,-2.01989740960257,11.1150036083138));
#49491=CARTESIAN_POINT('Ctrl Pts',(11.958402511919,0.937364159409468,10.9580034809616));
#49492=CARTESIAN_POINT('Ctrl Pts',(14.1039495688293,3.05397615607396,10.8010033536093));
#49493=CARTESIAN_POINT('Ctrl Pts',(17.0529568255832,2.43211293567374,10.6440032262571));
#49494=CARTESIAN_POINT('Ctrl Pts',(18.1610769073704,-0.370677272261844,
10.4870030989048));
#49495=CARTESIAN_POINT('Ctrl Pts',(16.4346192924356,-2.8410632437918,10.3300029715526));
#49496=CARTESIAN_POINT('Ctrl Pts',(13.4217297797568,-2.76384792766124,10.1730028442003));
#49497=CARTESIAN_POINT('Ctrl Pts',(11.8240877551162,-0.208259870614178,
10.0160027168481));
#49498=CARTESIAN_POINT('Ctrl Pts',(13.0743180231609,2.5340748647418,9.85900258949582));
#49499=CARTESIAN_POINT('Ctrl Pts',(16.0513251190755,3.00408135712897,9.70200246214356));
#49500=CARTESIAN_POINT('Ctrl Pts',(18.085599241322,0.780298763720488,9.54500233479132));
#49501=CARTESIAN_POINT('Ctrl Pts',(17.3529867440197,-2.14318495353929,9.38800220743906));
#49502=CARTESIAN_POINT('Ctrl Pts',(14.5104285512012,-3.14485429744199,9.23100208008681));
#49503=CARTESIAN_POINT('Ctrl Pts',(12.1068737263342,-1.32650255300144,9.07400195273456));
#49504=CARTESIAN_POINT('Ctrl Pts',(12.2976130105542,1.68133672093178,8.9170018253823));
#49505=CARTESIAN_POINT('Ctrl Pts',(14.9116086213649,3.1815052455197,8.76000169803005));
#49506=CARTESIAN_POINT('Ctrl Pts',(17.6048656357394,1.82878748503868,8.60300157067779));
#49507=CARTESIAN_POINT('Ctrl Pts',(17.9623146413344,-1.16382155298553,8.44600144332554));
#49508=CARTESIAN_POINT('Ctrl Pts',(15.663427690561,-3.11282064183558,8.28900131597329));
#49509=CARTESIAN_POINT('Ctrl Pts',(12.7696387641627,-2.27052359662139,8.13200118862103));
#49510=CARTESIAN_POINT('Ctrl Pts',(11.8758361555014,0.607773739041346,7.97500106126878));
#49511=CARTESIAN_POINT('Ctrl Pts',(13.7835012378397,2.94107453331316,7.81800093391652));
#49512=CARTESIAN_POINT('Ctrl Pts',(16.7820124308966,2.63708557646273,7.66100080656428));
#49513=CARTESIAN_POINT('Ctrl Pts',(18.1825759812315,-0.031603312774529,
7.50400067921202));
#49514=CARTESIAN_POINT('Ctrl Pts',(16.7292931170223,-2.67195321413115,7.34700055185977));
#49515=CARTESIAN_POINT('Ctrl Pts',(13.7253365245851,-2.9163370234462,7.1900004245075));
#49516=CARTESIAN_POINT('Ctrl Pts',(11.8643828993062,-0.545613467879027,
7.03300029715527));
#49517=CARTESIAN_POINT('Ctrl Pts',(12.8151672096171,2.31436696175991,6.876000169803));
#49518=CARTESIAN_POINT('Ctrl Pts',(15.725112044078,3.09903224993587,6.71900004245076));
#49519=CARTESIAN_POINT('Ctrl Pts',(17.9848419508889,1.10476575205979,6.56199991509849));
#49520=CARTESIAN_POINT('Ctrl Pts',(17.5680354476207,-1.8801551122215,6.40499978774625));
#49521=CARTESIAN_POINT('Ctrl Pts',(14.8484469168698,-3.17912223090478,6.24799966039399));
#49522=CARTESIAN_POINT('Ctrl Pts',(12.2647574994032,-1.62734115164585,6.09099953304174));
#49523=CARTESIAN_POINT('Ctrl Pts',(12.1337862540464,1.38369469820864,5.93399940568949));
#49524=CARTESIAN_POINT('Ctrl Pts',(14.5729764087098,3.15395366515346,5.77699927833723));
#49525=CARTESIAN_POINT('Ctrl Pts',(17.3950826426682,2.0960410275735,5.61999915098498));
#49526=CARTESIAN_POINT('Ctrl Pts',(18.0694954331843,-0.841429049439745,
5.46299902363272));
#49527=CARTESIAN_POINT('Ctrl Pts',(15.991461949452,-3.02434785364687,5.30599889628047));
#49528=CARTESIAN_POINT('Ctrl Pts',(13.0243755535244,-2.49537069256931,5.14899876892822));
#49529=CARTESIAN_POINT('Ctrl Pts',(11.8288495207139,0.271357391411547,4.99199864157596));
#49530=CARTESIAN_POINT('Ctrl Pts',(13.4769265545529,2.79450725974701,4.83499851422372));
#49531=CARTESIAN_POINT('Ctrl Pts',(16.4907542376736,2.81228145629323,4.67799838687145));
#49532=CARTESIAN_POINT('Ctrl Pts',(18.1678160134006,0.307309571682018,4.52099825951921));
#49533=CARTESIAN_POINT('Ctrl Pts',(17.0042508855994,-2.47138426111579,4.36399813216695));
#49534=CARTESIAN_POINT('Ctrl Pts',(14.0434946125838,-3.03758475218105,4.2069980048147));
#49535=CARTESIAN_POINT('Ctrl Pts',(11.9402762998377,-0.872627718934448,
4.04999787746244));
#49536=CARTESIAN_POINT('Ctrl Pts',(12.3681201524657,1.08091940906002,3.94533112589428));
#49537=CARTESIAN_POINT('Ctrl Pts',(12.9456684496579,1.75642532122687,3.89299775011019));
#49538=CARTESIAN_POINT('Ctrl Pts',(14.3498000020249,-2.43208680203506,12.3210067496694));
#49539=CARTESIAN_POINT('Ctrl Pts',(13.5500804955002,-2.21828784507023,12.2686733738853));
#49540=CARTESIAN_POINT('Ctrl Pts',(12.1909777974471,-0.944488908413503,
12.1640066223172));
#49541=CARTESIAN_POINT('Ctrl Pts',(12.6631613677687,1.82697676796832,12.0070064949649));
#49542=CARTESIAN_POINT('Ctrl Pts',(15.2345456504068,2.95446187741122,11.8500063676127));
#49543=CARTESIAN_POINT('Ctrl Pts',(17.593730939189,1.43545287811473,11.6930062402604));
#49544=CARTESIAN_POINT('Ctrl Pts',(17.6280542949882,-1.37216546154421,11.5360061129082));
#49545=CARTESIAN_POINT('Ctrl Pts',(15.3052827985147,-2.94861940676938,11.3790059855559));
#49546=CARTESIAN_POINT('Ctrl Pts',(12.7090145851187,-1.88139300561428,11.2220058582036));
#49547=CARTESIAN_POINT('Ctrl Pts',(12.1669649098191,0.873089081080348,11.0650057308514));
#49548=CARTESIAN_POINT('Ctrl Pts',(14.1653917640233,2.84456495267294,10.9080056034991));
#49549=CARTESIAN_POINT('Ctrl Pts',(16.9121855368091,2.26534290518294,10.7510054761469));
#49550=CARTESIAN_POINT('Ctrl Pts',(17.9443218034057,-0.345259924617078,
10.5940053487946));
#49551=CARTESIAN_POINT('Ctrl Pts',(16.3362474201295,-2.64625148285596,10.4370052214424));
#49552=CARTESIAN_POINT('Ctrl Pts',(13.5299517989286,-2.57433082242851,10.2800050940901));
#49553=CARTESIAN_POINT('Ctrl Pts',(12.0418601184578,-0.193979487305122,
10.1230049667379));
#49554=CARTESIAN_POINT('Ctrl Pts',(13.2063620731236,2.36031330282573,9.96600483938562));
#49555=CARTESIAN_POINT('Ctrl Pts',(15.9792357355636,2.79809144104539,9.80900471203338));
#49556=CARTESIAN_POINT('Ctrl Pts',(17.874019642361,0.726793662576183,9.65200458468112));
#49557=CARTESIAN_POINT('Ctrl Pts',(17.1916423980032,-1.99622672030653,9.49500445732887));
#49558=CARTESIAN_POINT('Ctrl Pts',(14.5439984748038,-2.92921157815017,9.33800432997662));
#49559=CARTESIAN_POINT('Ctrl Pts',(12.3052554502237,-1.23554424758505,9.18100420262436));
#49560=CARTESIAN_POINT('Ctrl Pts',(12.4829157380786,1.56604742983749,9.02400407527211));
#49561=CARTESIAN_POINT('Ctrl Pts',(14.9176696198875,2.96334937001758,8.86700394791986));
#49562=CARTESIAN_POINT('Ctrl Pts',(17.4262499493028,1.70338749223094,8.7100038205676));
#49563=CARTESIAN_POINT('Ctrl Pts',(17.7591886697512,-1.08401828684999,8.55300369321535));
#49564=CARTESIAN_POINT('Ctrl Pts',(15.6179364411373,-2.89937447092104,8.3960035658631));
#49565=CARTESIAN_POINT('Ctrl Pts',(12.922574676739,-2.11483375019832,8.23900343851085));
#49566=CARTESIAN_POINT('Ctrl Pts',(12.0900601300394,0.566098682137233,8.08200331115859));
#49567=CARTESIAN_POINT('Ctrl Pts',(13.8669165812153,2.73940499634305,7.92500318380633));
#49568=CARTESIAN_POINT('Ctrl Pts',(16.6598198044455,2.45626056807483,7.76800305645408));
#49569=CARTESIAN_POINT('Ctrl Pts',(17.9643466853611,-0.029436273013457,
7.61100292910183));
#49570=CARTESIAN_POINT('Ctrl Pts',(16.6107154549314,-2.4887373311618,7.45400280174958));
#49571=CARTESIAN_POINT('Ctrl Pts',(13.8127402234604,-2.71636373800054,7.29700267439732));
#49572=CARTESIAN_POINT('Ctrl Pts',(12.0793922238404,-0.508200741956758,
7.14000254704508));
#49573=CARTESIAN_POINT('Ctrl Pts',(12.9649812358183,2.15567077495119,6.98300241969281));
#49574=CARTESIAN_POINT('Ctrl Pts',(15.6753910973545,2.88653154931746,6.82600229234056));
#49575=CARTESIAN_POINT('Ctrl Pts',(17.780171281259,1.02901194332264,6.66900216498831));
#49576=CARTESIAN_POINT('Ctrl Pts',(17.3919452078874,-1.75123284023591,6.51200203763606));
#49577=CARTESIAN_POINT('Ctrl Pts',(14.8588389146771,-2.96112975876036,6.3550019102838));
#49578=CARTESIAN_POINT('Ctrl Pts',(12.4523131299553,-1.51575433776966,6.19800178293155));
#49579=CARTESIAN_POINT('Ctrl Pts',(12.3303225853962,1.28881472630212,6.04100165557929));
#49580=CARTESIAN_POINT('Ctrl Pts',(14.6022574245275,2.93768700204372,5.88400152822705));
#49581=CARTESIAN_POINT('Ctrl Pts',(17.2308517800767,1.95231545424541,5.72700140087478));
#49582=CARTESIAN_POINT('Ctrl Pts',(17.8590200726551,-0.783732243435121,
5.57000127352254));
#49583=CARTESIAN_POINT('Ctrl Pts',(15.9234773846255,-2.81696826350965,5.41300114617029));
#49584=CARTESIAN_POINT('Ctrl Pts',(13.1598441595847,-2.32426307647897,5.25600101881803));
#49585=CARTESIAN_POINT('Ctrl Pts',(12.0462953696974,0.252750409895257,5.09900089146578));
#49586=CARTESIAN_POINT('Ctrl Pts',(13.5813637298219,2.60288784352708,4.94200076411352));
#49587=CARTESIAN_POINT('Ctrl Pts',(16.3885331910994,2.61944326307635,4.78500063676127));
#49588=CARTESIAN_POINT('Ctrl Pts',(17.9505988088066,0.286237348477332,4.62800050940901));
#49589=CARTESIAN_POINT('Ctrl Pts',(16.8668193640612,-2.30192139508873,4.47100038205677));
#49590=CARTESIAN_POINT('Ctrl Pts',(14.1090822052833,-2.82929750765831,4.3140002547045));
#49591=CARTESIAN_POINT('Ctrl Pts',(12.1500816124467,-0.812791619566185,
4.15700012735226));
#49592=CARTESIAN_POINT('Ctrl Pts',(12.5485882039215,1.0068007445182,4.05233337578409));
#49593=CARTESIAN_POINT('Ctrl Pts',(13.086534003335,1.63598720337497,4.));
#49594=CARTESIAN_POINT('Ctrl Pts',(12.4841021658346,0.00201143405015815,
11.112583302492));
#49595=CARTESIAN_POINT('Ctrl Pts',(12.4821471482924,0.253216278985343,11.0967241119451));
#49596=CARTESIAN_POINT('Ctrl Pts',(12.5168205167969,0.503894392425629,11.0808649213983));
#49597=CARTESIAN_POINT('Ctrl Pts',(12.5903776647364,0.742588045230009,11.0650057308514));
#49598=CARTESIAN_POINT('Ctrl Pts',(12.8331071945538,1.53024770494455,11.0126723550673));
#49599=CARTESIAN_POINT('Ctrl Pts',(13.4992494792886,2.18740632880874,10.9603389792832));
#49600=CARTESIAN_POINT('Ctrl Pts',(14.2901195837869,2.41944863282584,10.9080056034991));
#49601=CARTESIAN_POINT('Ctrl Pts',(15.0809896882853,2.65149093684294,10.8556722277151));
#49602=CARTESIAN_POINT('Ctrl Pts',(15.9965876125472,2.45841692101294,10.803338851931));
#49603=CARTESIAN_POINT('Ctrl Pts',(16.6264092857776,1.92677944146461,10.7510054761469));
#49604=CARTESIAN_POINT('Ctrl Pts',(17.256230959008,1.39514196191627,10.6986721003628));
#49605=CARTESIAN_POINT('Ctrl Pts',(17.6002763812068,0.524941018649596,10.6463387245787));
#49606=CARTESIAN_POINT('Ctrl Pts',(17.5042866950936,-0.293658046023555,
10.5940053487946));
#49607=CARTESIAN_POINT('Ctrl Pts',(17.4082970089803,-1.11225711069671,10.5416719730106));
#49608=CARTESIAN_POINT('Ctrl Pts',(16.8722722145549,-1.87925429677634,10.4893385972265));
#49609=CARTESIAN_POINT('Ctrl Pts',(16.1365438804754,-2.25076611307824,10.4370052214424));
#49610=CARTESIAN_POINT('Ctrl Pts',(15.4008155463959,-2.62227792938014,10.3846718456583));
#49611=CARTESIAN_POINT('Ctrl Pts',(14.4653836726623,-2.59830437590432,10.3323384698742));
#49612=CARTESIAN_POINT('Ctrl Pts',(13.749652455717,-2.18959237664585,10.2800050940901));
#49613=CARTESIAN_POINT('Ctrl Pts',(13.0339212387717,-1.78088037738738,10.2276717183061));
#49614=CARTESIAN_POINT('Ctrl Pts',(12.5378906786147,-0.98742993234625,10.175338342522));
#49615=CARTESIAN_POINT('Ctrl Pts',(12.4839590576472,-0.164989244803877,
10.1230049667379));
#49616=CARTESIAN_POINT('Ctrl Pts',(12.4803790780928,-0.110395654006944,
10.1195310786559));
#49617=CARTESIAN_POINT('Ctrl Pts',(12.4787471194664,-0.0556743234800699,
10.1160571905739));
#49618=CARTESIAN_POINT('Ctrl Pts',(12.4790122776664,-0.000936909191352325,
10.112583302492));
#49619=CARTESIAN_POINT('Ctrl Pts',(14.2062007174671,-2.96922295374568,12.));
#49620=CARTESIAN_POINT('Ctrl Pts',(14.1131167498864,-2.9351724226013,12.));
#49621=CARTESIAN_POINT('Ctrl Pts',(14.0220959175279,-2.89635937351053,12.));
#49622=CARTESIAN_POINT('Ctrl Pts',(13.9333480734334,-2.85311020134011,12.));
#49623=CARTESIAN_POINT('Ctrl Pts',(13.8426550828426,-2.80891310782501,12.));
#49624=CARTESIAN_POINT('Ctrl Pts',(13.7543351402525,-2.76008268621842,12.));
#49625=CARTESIAN_POINT('Ctrl Pts',(13.6686411145779,-2.7069217762808,12.));
#49626=CARTESIAN_POINT('Ctrl Pts',(13.5868027530609,-2.65615275554924,12.));
#49627=CARTESIAN_POINT('Ctrl Pts',(13.5073590893475,-2.60143327816087,12.));
#49628=CARTESIAN_POINT('Ctrl Pts',(13.4305625059366,-2.54299781905995,12.));
#49629=CARTESIAN_POINT('Ctrl Pts',(13.3633654954521,-2.49186679234665,12.));
#49630=CARTESIAN_POINT('Ctrl Pts',(13.298195438544,-2.43789004325195,12.));
#49631=CARTESIAN_POINT('Ctrl Pts',(13.235245315039,-2.38121225533745,12.));
#49632=CARTESIAN_POINT('Ctrl Pts',(13.2201383978307,-2.36761058782836,12.));
#49633=CARTESIAN_POINT('Ctrl Pts',(13.2051557596309,-2.35384973663533,12.));
#49634=CARTESIAN_POINT('Ctrl Pts',(13.1903225084953,-2.33995287271397,12.));
#49635=CARTESIAN_POINT('Ctrl Pts',(13.1178922144325,-2.27209492767057,12.));
#49636=CARTESIAN_POINT('Ctrl Pts',(13.0489277577742,-2.20091637429481,12.));
#49637=CARTESIAN_POINT('Ctrl Pts',(12.9836701413723,-2.12670552844038,12.));
#49638=CARTESIAN_POINT('Ctrl Pts',(12.9187777778625,-2.05291004752833,12.));
#49639=CARTESIAN_POINT('Ctrl Pts',(12.8575503884276,-1.97611533073339,12.));
#49640=CARTESIAN_POINT('Ctrl Pts',(12.800268550456,-1.89657810132058,12.));
#49641=CARTESIAN_POINT('Ctrl Pts',(12.7459133734412,-1.82110461204208,12.));
#49642=CARTESIAN_POINT('Ctrl Pts',(12.6951108248742,-1.74316096291563,12.));
#49643=CARTESIAN_POINT('Ctrl Pts',(12.6481432361601,-1.66295348615981,12.));
#49644=CARTESIAN_POINT('Ctrl Pts',(12.6107661639977,-1.59912392350293,12.));
#49645=CARTESIAN_POINT('Ctrl Pts',(12.5758185286433,-1.533860318552,12.));
#49646=CARTESIAN_POINT('Ctrl Pts',(12.5434639629309,-1.46726456665475,12.));
#49647=CARTESIAN_POINT('Ctrl Pts',(12.5375614518629,-1.45511536440159,12.));
#49648=CARTESIAN_POINT('Ctrl Pts',(12.5317470084536,-1.4429252625298,12.));
#49649=CARTESIAN_POINT('Ctrl Pts',(12.5260248255016,-1.43070222232707,12.));
#49650=CARTESIAN_POINT('Ctrl Pts',(12.4854475610481,-1.34402594180728,12.));
#49651=CARTESIAN_POINT('Ctrl Pts',(12.4494522312093,-1.25558570069036,12.));
#49652=CARTESIAN_POINT('Ctrl Pts',(12.4183023908741,-1.16562505800954,12.));
#49653=CARTESIAN_POINT('Ctrl Pts',(12.3871525505389,-1.07566441532873,12.));
#49654=CARTESIAN_POINT('Ctrl Pts',(12.3608477335802,-0.984182637916221,
12.));
#49655=CARTESIAN_POINT('Ctrl Pts',(12.3397077040223,-0.891413467157708,
12.));
#49656=CARTESIAN_POINT('Ctrl Pts',(12.3185427547458,-0.798534940751147,
12.));
#49657=CARTESIAN_POINT('Ctrl Pts',(12.3025555503081,-0.704364799779564,
12.));
#49658=CARTESIAN_POINT('Ctrl Pts',(12.2916706351494,-0.609311329981899,
12.));
#49659=CARTESIAN_POINT('Ctrl Pts',(12.2861036872675,-0.560697472671795,
12.));
#49660=CARTESIAN_POINT('Ctrl Pts',(12.2818721595795,-0.511852737800975,
12.));
#49661=CARTESIAN_POINT('Ctrl Pts',(12.2789708979829,-0.462833545994333,
12.));
#49662=CARTESIAN_POINT('Ctrl Pts',(12.2781343831999,-0.448699943341852,
12.));
#49663=CARTESIAN_POINT('Ctrl Pts',(12.277408477694,-0.434551848133338,12.));
#49664=CARTESIAN_POINT('Ctrl Pts',(12.2767931065317,-0.42039064034991,12.));
#49665=CARTESIAN_POINT('Ctrl Pts',(12.2761719502385,-0.406096302442059,
12.));
#49666=CARTESIAN_POINT('Ctrl Pts',(12.2756638189297,-0.391797511344244,
12.));
#49667=CARTESIAN_POINT('Ctrl Pts',(12.2752682723578,-0.377498729044968,
12.));
#49668=CARTESIAN_POINT('Ctrl Pts',(12.2726875200461,-0.28420600930709,12.));
#49669=CARTESIAN_POINT('Ctrl Pts',(12.2748931639065,-0.190870392884388,
12.));
#49670=CARTESIAN_POINT('Ctrl Pts',(12.2817566653744,-0.0978690578159151,
12.));
#49671=CARTESIAN_POINT('Ctrl Pts',(12.2886243750566,-0.004810700899435,
12.));
#49672=CARTESIAN_POINT('Ctrl Pts',(12.3001560328895,0.0879139420894839,
12.));
#49673=CARTESIAN_POINT('Ctrl Pts',(12.3162734180046,0.179914286846824,12.));
#49674=CARTESIAN_POINT('Ctrl Pts',(12.3321476400437,0.270526621907842,12.));
#49675=CARTESIAN_POINT('Ctrl Pts',(12.3524707190227,0.360437184721369,12.));
#49676=CARTESIAN_POINT('Ctrl Pts',(12.3772105840448,0.449247114668589,12.));
#49677=CARTESIAN_POINT('Ctrl Pts',(12.387089561874,0.484710175124557,12.));
#49678=CARTESIAN_POINT('Ctrl Pts',(12.3976732487818,0.519997379566271,12.));
#49679=CARTESIAN_POINT('Ctrl Pts',(12.4089613041164,0.555081714039806,12.));
#49680=CARTESIAN_POINT('Ctrl Pts',(12.4149082466012,0.573565368933964,12.));
#49681=CARTESIAN_POINT('Ctrl Pts',(12.4210507056737,0.591992698996559,12.));
#49682=CARTESIAN_POINT('Ctrl Pts',(12.427388732547,0.610359631690939,12.));
#49683=CARTESIAN_POINT('Ctrl Pts',(12.4327450955641,0.62588180617673,12.));
#49684=CARTESIAN_POINT('Ctrl Pts',(12.4382385696775,0.641353302839583,12.));
#49685=CARTESIAN_POINT('Ctrl Pts',(12.4438669442654,0.656766888688516,12.));
#49686=CARTESIAN_POINT('Ctrl Pts',(12.4746822935363,0.741156266835812,12.));
#49687=CARTESIAN_POINT('Ctrl Pts',(12.5095548332415,0.823860554446091,12.));
#49688=CARTESIAN_POINT('Ctrl Pts',(12.5484325218527,0.904509504080283,12.));
#49689=CARTESIAN_POINT('Ctrl Pts',(12.5775387438767,0.964888253895875,12.));
#49690=CARTESIAN_POINT('Ctrl Pts',(12.6088907149234,1.02411455960934,12.));
#49691=CARTESIAN_POINT('Ctrl Pts',(12.6424801735134,1.08201977519688,12.));
#49692=CARTESIAN_POINT('Ctrl Pts',(12.6553986892758,1.10429013833142,12.));
#49693=CARTESIAN_POINT('Ctrl Pts',(12.6686482828058,1.12636495172308,12.));
#49694=CARTESIAN_POINT('Ctrl Pts',(12.6822288987083,1.1482340709878,12.));
#49695=CARTESIAN_POINT('Ctrl Pts',(12.6939913183076,1.16717531480961,12.));
#49696=CARTESIAN_POINT('Ctrl Pts',(12.706004041963,1.18596501264398,12.));
#49697=CARTESIAN_POINT('Ctrl Pts',(12.7182527989854,1.20457528100954,12.));
#49698=CARTESIAN_POINT('Ctrl Pts',(12.765524404259,1.27639785521913,12.));
#49699=CARTESIAN_POINT('Ctrl Pts',(12.8163473248132,1.34561526270953,12.));
#49700=CARTESIAN_POINT('Ctrl Pts',(12.8706925767079,1.41187353983322,12.));
#49701=CARTESIAN_POINT('Ctrl Pts',(12.9128273378038,1.46324466389474,12.));
#49702=CARTESIAN_POINT('Ctrl Pts',(12.9570801591186,1.51283644006015,12.));
#49703=CARTESIAN_POINT('Ctrl Pts',(13.0034499581199,1.56046614478315,12.));
#49704=CARTESIAN_POINT('Ctrl Pts',(13.0293158880168,1.58703487335031,12.));
#49705=CARTESIAN_POINT('Ctrl Pts',(13.0558407610521,1.61299275362867,12.));
#49706=CARTESIAN_POINT('Ctrl Pts',(13.0829974340784,1.63832794503775,12.));
#49707=CARTESIAN_POINT('Origin',(15.,0.,7.5));
#49708=CARTESIAN_POINT('Origin',(-7.5,12.9903810567666,4.));
#49709=CARTESIAN_POINT('Ctrl Pts',(-9.41346599666504,14.6263682601415,4.));
#49710=CARTESIAN_POINT('Ctrl Pts',(-9.47563132777586,14.5679481137415,4.));
#49711=CARTESIAN_POINT('Ctrl Pts',(-9.53442555802215,14.506276247837,4.));
#49712=CARTESIAN_POINT('Ctrl Pts',(-9.58983471826803,14.4417285757633,4.));
#49713=CARTESIAN_POINT('Ctrl Pts',(-9.64659435921208,14.3756076911582,4.));
#49714=CARTESIAN_POINT('Ctrl Pts',(-9.69980238305237,14.3064686172689,4.));
#49715=CARTESIAN_POINT('Ctrl Pts',(-9.7494149473681,14.2346691598829,4.));
#49716=CARTESIAN_POINT('Ctrl Pts',(-9.76242041292079,14.2158476096845,4.));
#49717=CARTESIAN_POINT('Ctrl Pts',(-9.77517863474719,14.1968430256296,4.));
#49718=CARTESIAN_POINT('Ctrl Pts',(-9.78768844229491,14.177661413676,4.));
#49719=CARTESIAN_POINT('Ctrl Pts',(-9.79776816908292,14.1622059074975,4.));
#49720=CARTESIAN_POINT('Ctrl Pts',(-9.80768698071961,14.1466346904616,4.));
#49721=CARTESIAN_POINT('Ctrl Pts',(-9.81743563533852,14.1309651390747,4.));
#49722=CARTESIAN_POINT('Ctrl Pts',(-9.86491280549081,14.0546524593777,4.));
#49723=CARTESIAN_POINT('Ctrl Pts',(-9.90840772399799,13.9759343990068,4.));
#49724=CARTESIAN_POINT('Ctrl Pts',(-9.94788354450479,13.8952025688597,4.));
#49725=CARTESIAN_POINT('Ctrl Pts',(-9.97942538424941,13.8306964885275,4.));
#49726=CARTESIAN_POINT('Ctrl Pts',(-10.0084008056984,13.7649036744675,4.));
#49727=CARTESIAN_POINT('Ctrl Pts',(-10.0347744493784,13.6980066802042,4.));
#49728=CARTESIAN_POINT('Ctrl Pts',(-10.0434535064654,13.6759921705975,4.));
#49729=CARTESIAN_POINT('Ctrl Pts',(-10.0518506786378,13.6538579807081,4.));
#49730=CARTESIAN_POINT('Ctrl Pts',(-10.0599643178554,13.6316103344208,4.));
#49731=CARTESIAN_POINT('Ctrl Pts',(-10.0673321856527,13.6114075977388,4.));
#49732=CARTESIAN_POINT('Ctrl Pts',(-10.0744676826305,13.591106675655,4.));
#49733=CARTESIAN_POINT('Ctrl Pts',(-10.0813601244641,13.5707407736482,4.));
#49734=CARTESIAN_POINT('Ctrl Pts',(-10.110937889366,13.4833439009404,4.));
#49735=CARTESIAN_POINT('Ctrl Pts',(-10.1360768470728,13.3946653712955,4.));
#49736=CARTESIAN_POINT('Ctrl Pts',(-10.1567422986514,13.3051020151044,4.));
#49737=CARTESIAN_POINT('Ctrl Pts',(-10.1777244132853,13.2141662521254,4.));
#49738=CARTESIAN_POINT('Ctrl Pts',(-10.194095376586,13.1223175335281,4.));
#49739=CARTESIAN_POINT('Ctrl Pts',(-10.205777094777,13.0299380601523,4.));
#49740=CARTESIAN_POINT('Ctrl Pts',(-10.2173678863481,12.938277637958,4.));
#49741=CARTESIAN_POINT('Ctrl Pts',(-10.2243424959595,12.8460937642312,4.));
#49742=CARTESIAN_POINT('Ctrl Pts',(-10.2265776894176,12.7537405691803,4.));
#49743=CARTESIAN_POINT('Ctrl Pts',(-10.2276571919675,12.7091379379498,4.));
#49744=CARTESIAN_POINT('Ctrl Pts',(-10.2276305022847,12.6644956114825,4.));
#49745=CARTESIAN_POINT('Ctrl Pts',(-10.226479393828,12.619852841063,4.));
#49746=CARTESIAN_POINT('Ctrl Pts',(-10.2261091350259,12.6054933090796,4.));
#49747=CARTESIAN_POINT('Ctrl Pts',(-10.2256225193086,12.5911337303501,4.));
#49748=CARTESIAN_POINT('Ctrl Pts',(-10.225018873735,12.5767754108853,4.));
#49749=CARTESIAN_POINT('Ctrl Pts',(-10.2243878291515,12.5617653783061,4.));
#49750=CARTESIAN_POINT('Ctrl Pts',(-10.2236292144324,12.5467651944381,4.));
#49751=CARTESIAN_POINT('Ctrl Pts',(-10.2227430773117,12.5317818464922,4.));
#49752=CARTESIAN_POINT('Ctrl Pts',(-10.21709364836,12.436257849471,4.));
#49753=CARTESIAN_POINT('Ctrl Pts',(-10.2062620470353,12.3413497626712,4.));
#49754=CARTESIAN_POINT('Ctrl Pts',(-10.1901757223778,12.2474518873064,4.));
#49755=CARTESIAN_POINT('Ctrl Pts',(-10.1886872627285,12.2387635634276,4.));
#49756=CARTESIAN_POINT('Ctrl Pts',(-10.1871537792193,12.2300838755081,4.));
#49757=CARTESIAN_POINT('Ctrl Pts',(-10.1855751929644,12.2214131286805,4.));
#49758=CARTESIAN_POINT('Ctrl Pts',(-10.1691864185716,12.1313940289104,4.));
#49759=CARTESIAN_POINT('Ctrl Pts',(-10.1479406949308,12.0423388878924,4.));
#49760=CARTESIAN_POINT('Ctrl Pts',(-10.1221403086027,11.9544825435439,4.));
#49761=CARTESIAN_POINT('Ctrl Pts',(-10.095748827746,11.8646133842016,4.));
#49762=CARTESIAN_POINT('Ctrl Pts',(-10.0645913960745,11.7759978814463,4.));
#49763=CARTESIAN_POINT('Ctrl Pts',(-10.0289372513566,11.6888902934565,4.));
#49764=CARTESIAN_POINT('Ctrl Pts',(-10.0090455594271,11.6402923725491,4.));
#49765=CARTESIAN_POINT('Ctrl Pts',(-9.98775327367975,11.5921639163278,4.));
#49766=CARTESIAN_POINT('Ctrl Pts',(-9.96510045219232,11.5445507349067,4.));
#49767=CARTESIAN_POINT('Ctrl Pts',(-9.95876521331174,11.5312349155799,4.));
#49768=CARTESIAN_POINT('Ctrl Pts',(-9.95232326498233,11.517959024353,4.));
#49769=CARTESIAN_POINT('Ctrl Pts',(-9.94578250287666,11.504737914807,4.));
#49770=CARTESIAN_POINT('Ctrl Pts',(-9.90302508933715,11.4183106087567,4.));
#49771=CARTESIAN_POINT('Ctrl Pts',(-9.85598190542476,11.3340799660434,4.));
#49772=CARTESIAN_POINT('Ctrl Pts',(-9.80499298346813,11.2522993127725,4.));
#49773=CARTESIAN_POINT('Ctrl Pts',(-9.75299886407878,11.1689064327755,4.));
#49774=CARTESIAN_POINT('Ctrl Pts',(-9.69690158938222,11.0880603146916,4.));
#49775=CARTESIAN_POINT('Ctrl Pts',(-9.63700679973682,11.0100365149775,4.));
#49776=CARTESIAN_POINT('Ctrl Pts',(-9.57664072131881,10.9313987763712,4.));
#49777=CARTESIAN_POINT('Ctrl Pts',(-9.5124166745289,10.855627103721,4.00000000000001));
#49778=CARTESIAN_POINT('Ctrl Pts',(-9.44459833298039,10.7830228983692,4.00000000000001));
#49779=CARTESIAN_POINT('Ctrl Pts',(-9.40866399637306,10.7445527161936,4.00000000000001));
#49780=CARTESIAN_POINT('Ctrl Pts',(-9.37171976510391,10.706972211061,4.));
#49781=CARTESIAN_POINT('Ctrl Pts',(-9.33380001260192,10.67032964942,4.));
#49782=CARTESIAN_POINT('Ctrl Pts',(-9.31851279266197,10.655557324655,4.));
#49783=CARTESIAN_POINT('Ctrl Pts',(-9.30306698875868,10.6409374727743,4.00000000000001));
#49784=CARTESIAN_POINT('Ctrl Pts',(-9.28746471547238,10.6264733925429,4.00000000000001));
#49785=CARTESIAN_POINT('Ctrl Pts',(-9.27676484992977,10.616554087142,4.00000000000001));
#49786=CARTESIAN_POINT('Ctrl Pts',(-9.265998221379,10.6067143856922,4.00000000000001));
#49787=CARTESIAN_POINT('Ctrl Pts',(-9.25516722641356,10.5969563651344,4.00000000000001));
#49788=CARTESIAN_POINT('Ctrl Pts',(-9.17938034347013,10.5286773229844,4.));
#49789=CARTESIAN_POINT('Ctrl Pts',(-9.10042408605055,10.4643755397515,4.));
#49790=CARTESIAN_POINT('Ctrl Pts',(-9.01862125042457,10.4043372079866,4.));
#49791=CARTESIAN_POINT('Ctrl Pts',(-8.9367488325877,10.344247807089,4.));
#49792=CARTESIAN_POINT('Ctrl Pts',(-8.85202442117708,10.2884282704825,4.));
#49793=CARTESIAN_POINT('Ctrl Pts',(-8.76472673601652,10.2371917535793,4.00000000000001));
#49794=CARTESIAN_POINT('Ctrl Pts',(-8.67911981959232,10.1869475780055,4.00000000000001));
#49795=CARTESIAN_POINT('Ctrl Pts',(-8.59103768625539,10.1411099279233,4.));
#49796=CARTESIAN_POINT('Ctrl Pts',(-8.50070929346997,10.1000104724858,4.));
#49797=CARTESIAN_POINT('Ctrl Pts',(-8.47449841652962,10.0880845128227,4.));
#49798=CARTESIAN_POINT('Ctrl Pts',(-8.4480982164028,10.0765577851635,4.));
#49799=CARTESIAN_POINT('Ctrl Pts',(-8.42151385798486,10.0654391093543,4.));
#49800=CARTESIAN_POINT('Ctrl Pts',(-8.38003010456224,10.0480888916659,4.));
#49801=CARTESIAN_POINT('Ctrl Pts',(-8.33809795636191,10.0317321930114,4.));
#49802=CARTESIAN_POINT('Ctrl Pts',(-8.29574920379127,10.0163624306404,4.));
#49803=CARTESIAN_POINT('Ctrl Pts',(-6.70620071746715,10.0211581030209,4.));
#49804=CARTESIAN_POINT('Ctrl Pts',(-6.61134536198573,10.0558566157721,4.));
#49805=CARTESIAN_POINT('Ctrl Pts',(-6.51853047906358,10.0955386450798,4.));
#49806=CARTESIAN_POINT('Ctrl Pts',(-6.42799833026157,10.1398859077314,4.));
#49807=CARTESIAN_POINT('Ctrl Pts',(-6.33621672682966,10.1848452169695,4.));
#49808=CARTESIAN_POINT('Ctrl Pts',(-6.24678063208038,10.2346001195317,4.));
#49809=CARTESIAN_POINT('Ctrl Pts',(-6.15997649545542,10.288859611306,4.));
#49810=CARTESIAN_POINT('Ctrl Pts',(-6.13531542249315,10.3042747440124,4.));
#49811=CARTESIAN_POINT('Ctrl Pts',(-6.11086702515844,10.3200536672633,4.));
#49812=CARTESIAN_POINT('Ctrl Pts',(-6.0866384800126,10.3361901726906,4.));
#49813=CARTESIAN_POINT('Ctrl Pts',(-6.06744058816026,10.3489762019054,4.));
#49814=CARTESIAN_POINT('Ctrl Pts',(-6.04837875428141,10.3619882719582,4.));
#49815=CARTESIAN_POINT('Ctrl Pts',(-6.0294755109822,10.37520976247,4.));
#49816=CARTESIAN_POINT('Ctrl Pts',(-5.9467711696009,10.43305563831,4.));
#49817=CARTESIAN_POINT('Ctrl Pts',(-5.86702033335456,10.4949586291912,4.));
#49818=CARTESIAN_POINT('Ctrl Pts',(-5.79049045427403,10.5606238082624,4.));
#49819=CARTESIAN_POINT('Ctrl Pts',(-5.73202499106291,10.6107891183003,4.));
#49820=CARTESIAN_POINT('Ctrl Pts',(-5.67544001899664,10.6631510546145,4.));
#49821=CARTESIAN_POINT('Ctrl Pts',(-5.62087181378523,10.7175895430331,4.));
#49822=CARTESIAN_POINT('Ctrl Pts',(-5.59237441395403,10.7460192002787,4.));
#49823=CARTESIAN_POINT('Ctrl Pts',(-5.56442730562685,10.7750153331146,4.));
#49824=CARTESIAN_POINT('Ctrl Pts',(-5.53705172637329,10.8045615976092,4.));
#49825=CARTESIAN_POINT('Ctrl Pts',(-5.52590399611565,10.8165932621689,4.));
#49826=CARTESIAN_POINT('Ctrl Pts',(-5.51485083286264,10.828716515658,4.));
#49827=CARTESIAN_POINT('Ctrl Pts',(-5.50390377375039,10.8409187451704,4.));
#49828=CARTESIAN_POINT('Ctrl Pts',(-5.43813900242605,10.9142239886428,4.));
#49829=CARTESIAN_POINT('Ctrl Pts',(-5.37610793089156,10.9904753850308,4.));
#49830=CARTESIAN_POINT('Ctrl Pts',(-5.31805547404601,11.0693968127291,4.));
#49831=CARTESIAN_POINT('Ctrl Pts',(-5.26107067938322,11.14686677001,4.));
#49832=CARTESIAN_POINT('Ctrl Pts',(-5.20791915062963,11.2269102402285,4.));
#49833=CARTESIAN_POINT('Ctrl Pts',(-5.15887680160751,11.3092877421736,4.));
#49834=CARTESIAN_POINT('Ctrl Pts',(-5.11076852001942,11.390096270703,4.));
#49835=CARTESIAN_POINT('Ctrl Pts',(-5.0666140967032,11.4731514387505,4.));
#49836=CARTESIAN_POINT('Ctrl Pts',(-5.0267215928916,11.558237595229,4.));
#49837=CARTESIAN_POINT('Ctrl Pts',(-5.00642757575884,11.6015224169963,4.));
#49838=CARTESIAN_POINT('Ctrl Pts',(-4.98723731004213,11.6453329516309,4.));
#49839=CARTESIAN_POINT('Ctrl Pts',(-4.96919657902753,11.6896410472644,4.));
#49840=CARTESIAN_POINT('Ctrl Pts',(-4.96034359773442,11.7113839988919,4.));
#49841=CARTESIAN_POINT('Ctrl Pts',(-4.95176748954608,11.7332467663051,4.));
#49842=CARTESIAN_POINT('Ctrl Pts',(-4.94347399674913,11.7552260059165,4.));
#49843=CARTESIAN_POINT('Ctrl Pts',(-4.93874124380541,11.7677686479032,4.));
#49844=CARTESIAN_POINT('Ctrl Pts',(-4.93410183231377,11.780345881655,4.));
#49845=CARTESIAN_POINT('Ctrl Pts',(-4.92955939125163,11.7929492290495,4.));
#49846=CARTESIAN_POINT('Ctrl Pts',(-4.89805310423436,11.8803658129868,4.));
#49847=CARTESIAN_POINT('Ctrl Pts',(-4.87116553516298,11.9691490179121,4.));
#49848=CARTESIAN_POINT('Ctrl Pts',(-4.84914983533523,12.059077444786,4.));
#49849=CARTESIAN_POINT('Ctrl Pts',(-4.84589756836606,12.0723621123006,4.));
#49850=CARTESIAN_POINT('Ctrl Pts',(-4.84275170968814,12.0856717889067,4.));
#49851=CARTESIAN_POINT('Ctrl Pts',(-4.83971317200452,12.0990057760668,4.));
#49852=CARTESIAN_POINT('Ctrl Pts',(-4.81880138299547,12.1907727887468,4.));
#49853=CARTESIAN_POINT('Ctrl Pts',(-4.80296850182884,12.2836914928978,4.));
#49854=CARTESIAN_POINT('Ctrl Pts',(-4.792106149773,12.377370023065,4.));
#49855=CARTESIAN_POINT('Ctrl Pts',(-4.78082380016171,12.4746706742486,4.));
#49856=CARTESIAN_POINT('Ctrl Pts',(-4.77490383217972,12.5727922441963,4.));
#49857=CARTESIAN_POINT('Ctrl Pts',(-4.77428144864228,12.6712822681824,4.));
#49858=CARTESIAN_POINT('Ctrl Pts',(-4.77410039443767,12.6999334645636,4.));
#49859=CARTESIAN_POINT('Ctrl Pts',(-4.77436800145517,12.72861569198,4.));
#49860=CARTESIAN_POINT('Ctrl Pts',(-4.77508351480076,12.7573173782009,4.));
#49861=CARTESIAN_POINT('Ctrl Pts',(-4.77547910205812,12.7731857353794,4.));
#49862=CARTESIAN_POINT('Ctrl Pts',(-4.77601160613275,12.7890600363428,4.));
#49863=CARTESIAN_POINT('Ctrl Pts',(-4.77668094646708,12.8049382921795,4.));
#49864=CARTESIAN_POINT('Ctrl Pts',(-4.77726157393708,12.8187120796562,4.));
#49865=CARTESIAN_POINT('Ctrl Pts',(-4.77794517105296,12.8324874411773,4.));
#49866=CARTESIAN_POINT('Ctrl Pts',(-4.77873077105928,12.846250960695,4.));
#49867=CARTESIAN_POINT('Ctrl Pts',(-4.7840331030193,12.9391465167459,4.));
#49868=CARTESIAN_POINT('Ctrl Pts',(-4.79398369008647,13.0316542436184,4.));
#49869=CARTESIAN_POINT('Ctrl Pts',(-4.80846381204201,13.1234011743035,4.));
#49870=CARTESIAN_POINT('Ctrl Pts',(-4.82290319752883,13.2148899962528,4.));
#49871=CARTESIAN_POINT('Ctrl Pts',(-4.84184707271793,13.3056232412176,4.));
#49872=CARTESIAN_POINT('Ctrl Pts',(-4.86522626081521,13.3952139858104,4.));
#49873=CARTESIAN_POINT('Ctrl Pts',(-4.88820180858057,13.4832579513734,4.));
#49874=CARTESIAN_POINT('Ctrl Pts',(-4.91546130118121,13.5701993091168,4.));
#49875=CARTESIAN_POINT('Ctrl Pts',(-4.94697947428434,13.6556416339958,4.));
#49876=CARTESIAN_POINT('Ctrl Pts',(-4.9623719301486,13.6973689006853,4.));
#49877=CARTESIAN_POINT('Ctrl Pts',(-4.97878066818245,13.7387381251278,4.));
#49878=CARTESIAN_POINT('Ctrl Pts',(-4.99620585058615,13.779699693788,4.));
#49879=CARTESIAN_POINT('Ctrl Pts',(-5.00196797407456,13.7932447810892,4.));
#49880=CARTESIAN_POINT('Ctrl Pts',(-5.00784125922211,13.8067452713773,4.));
#49881=CARTESIAN_POINT('Ctrl Pts',(-5.01382575727085,13.8201993070928,4.));
#49882=CARTESIAN_POINT('Ctrl Pts',(-5.01951346999181,13.8329861255467,4.));
#49883=CARTESIAN_POINT('Ctrl Pts',(-5.02529821878992,13.8457232464252,4.));
#49884=CARTESIAN_POINT('Ctrl Pts',(-5.03117811610162,13.8584059204054,4.));
#49885=CARTESIAN_POINT('Ctrl Pts',(-5.06862984407309,13.9391876127847,4.));
#49886=CARTESIAN_POINT('Ctrl Pts',(-5.10995846184345,14.0178080548726,4.));
#49887=CARTESIAN_POINT('Ctrl Pts',(-5.15509821873846,14.0939187469392,4.));
#49888=CARTESIAN_POINT('Ctrl Pts',(-5.19948177774165,14.1687544045606,4.));
#49889=CARTESIAN_POINT('Ctrl Pts',(-5.24755030145435,14.2411643668113,4.));
#49890=CARTESIAN_POINT('Ctrl Pts',(-5.299277628138,14.3107831411822,4.));
#49891=CARTESIAN_POINT('Ctrl Pts',(-5.34947359960038,14.37834089519,4.));
#49892=CARTESIAN_POINT('Ctrl Pts',(-5.40311538240653,14.4432707274223,4.));
#49893=CARTESIAN_POINT('Ctrl Pts',(-5.46020707398797,14.5051981890779,4.));
#49894=CARTESIAN_POINT('Ctrl Pts',(-5.47440626361873,14.5206000758857,4.));
#49895=CARTESIAN_POINT('Ctrl Pts',(-5.48881897228929,14.5358160294758,4.));
#49896=CARTESIAN_POINT('Ctrl Pts',(-5.50344549658044,14.5508398362218,4.));
#49897=CARTESIAN_POINT('Ctrl Pts',(-5.52930175835117,14.5773984001217,4.));
#49898=CARTESIAN_POINT('Ctrl Pts',(-5.55582619547196,14.603356583853,4.));
#49899=CARTESIAN_POINT('Ctrl Pts',(-5.58299280741585,14.6287008947316,4.));
#49900=CARTESIAN_POINT('Origin',(-7.5,12.9903810567666,14.2084234471775));
#49901=CARTESIAN_POINT('Ctrl Pts',(-10.5771718362758,12.9919049495641,11.7084234471775));
#49902=CARTESIAN_POINT('Ctrl Pts',(-10.5778105116372,13.0907937922778,11.7032843782051));
#49903=CARTESIAN_POINT('Ctrl Pts',(-10.5289894981275,14.1961054493059,11.6458119334487));
#49904=CARTESIAN_POINT('Ctrl Pts',(-9.19520332408216,16.188335839362,11.5360061129082));
#49905=CARTESIAN_POINT('Ctrl Pts',(-5.76804722455709,16.1681372027015,11.3790059855559));
#49906=CARTESIAN_POINT('Ctrl Pts',(-3.89395310615829,13.2989500353867,11.2220058582037));
#49907=CARTESIAN_POINT('Ctrl Pts',(-5.25343413560966,10.1527921984098,11.0650057308514));
#49908=CARTESIAN_POINT('Ctrl Pts',(-8.62743319586002,9.55126751773617,10.9080056034992));
#49909=CARTESIAN_POINT('Ctrl Pts',(-10.416413733365,11.4305453719444,10.7891448422745));
#49910=CARTESIAN_POINT('Ctrl Pts',(-10.5747253393417,12.713490324996,10.7226174568339));
#49911=CARTESIAN_POINT('Ctrl Pts',(-10.5724150045772,12.9877735244422,10.7084234471775));
#49912=CARTESIAN_POINT('Ctrl Pts',(-10.5702206634037,12.9870745539208,11.7915765528226));
#49913=CARTESIAN_POINT('Ctrl Pts',(-10.5655505963514,13.6681072977096,11.7563842836469));
#49914=CARTESIAN_POINT('Ctrl Pts',(-10.0102057878341,15.3711021382601,11.6688586386871));
#49915=CARTESIAN_POINT('Ctrl Pts',(-7.21365218567195,16.5973810760335,11.5289996179432));
#49916=CARTESIAN_POINT('Ctrl Pts',(-4.33342713054201,14.7428462583649,11.371999490591));
#49917=CARTESIAN_POINT('Ctrl Pts',(-4.29152522806557,11.3151739482887,11.2149993632387));
#49918=CARTESIAN_POINT('Ctrl Pts',(-7.12729264284838,9.39053585671186,11.0579992358865));
#49919=CARTESIAN_POINT('Ctrl Pts',(-9.97678331927841,10.5618592714599,10.9168582990811));
#49920=CARTESIAN_POINT('Ctrl Pts',(-10.5660598502819,12.2874997426315,10.8280507380598));
#49921=CARTESIAN_POINT('Ctrl Pts',(-10.5715490487462,12.9928368154298,10.7915765528225));
#49922=CARTESIAN_POINT('Ctrl Pts',(-5.58653400333492,14.6263682601415,12.));
#49923=CARTESIAN_POINT('Ctrl Pts',(-5.04858820392146,13.9971818012847,11.9476666242159));
#49924=CARTESIAN_POINT('Ctrl Pts',(-4.6501298356162,12.1775391083675,11.8429998726477));
#49925=CARTESIAN_POINT('Ctrl Pts',(-6.60905434274384,10.1611067275626,11.6859997452955));
#49926=CARTESIAN_POINT('Ctrl Pts',(-9.36683572422696,10.6884384302024,11.5289996179432));
#49927=CARTESIAN_POINT('Ctrl Pts',(-10.4505967777648,13.2766298839747,11.371999490591));
#49928=CARTESIAN_POINT('Ctrl Pts',(-8.88853891927017,15.609821813293,11.2149993632387));
#49929=CARTESIAN_POINT('Ctrl Pts',(-6.0813596511542,15.5932771353061,11.0579992358865));
#49930=CARTESIAN_POINT('Ctrl Pts',(-4.5462915063457,13.2431295206274,10.9009991085342));
#49931=CARTESIAN_POINT('Ctrl Pts',(-5.65984071462414,10.666115577374,10.743998981182));
#49932=CARTESIAN_POINT('Ctrl Pts',(-8.42347911845702,10.1734074649302,10.5869988538297));
#49933=CARTESIAN_POINT('Ctrl Pts',(-10.3590245740303,12.2066479805288,10.4299987264775));
#49934=CARTESIAN_POINT('Ctrl Pts',(-9.73085545152254,14.9426994258741,10.2729985991252));
#49935=CARTESIAN_POINT('Ctrl Pts',(-7.10225674886102,15.9280729453192,10.115998471773));
#49936=CARTESIAN_POINT('Ctrl Pts',(-4.8303182837872,14.2791977933351,9.9589983444207));
#49937=CARTESIAN_POINT('Ctrl Pts',(-4.95230900060974,11.4746243081013,9.80199821706846));
#49938=CARTESIAN_POINT('Ctrl Pts',(-7.35883869070172,10.0292464861065,9.64499808971619));
#49939=CARTESIAN_POINT('Ctrl Pts',(-9.89194907460283,11.2391453960705,9.48799796236395));
#49940=CARTESIAN_POINT('Ctrl Pts',(-10.2801757792987,14.0193946579201,9.33099783501168));
#49941=CARTESIAN_POINT('Ctrl Pts',(-8.17539218920641,15.8769172785782,9.17399770765945));
#49942=CARTESIAN_POINT('Ctrl Pts',(-5.46497794449781,15.1460553165716,9.01699758030717));
#49943=CARTESIAN_POINT('Ctrl Pts',(-4.57938749963505,12.4821794938336,8.85999745295494));
#49944=CARTESIAN_POINT('Ctrl Pts',(-6.31273830315983,10.2740129245224,8.70299732560267));
#49945=CARTESIAN_POINT('Ctrl Pts',(-9.11071806020523,10.501639700397,8.54599719825042));
#49946=CARTESIAN_POINT('Ctrl Pts',(-10.4643514801813,12.96094473598,8.38899707089817));
#49947=CARTESIAN_POINT('Ctrl Pts',(-9.15982248917363,15.4466455979041,8.23199694354592));
#49948=CARTESIAN_POINT('Ctrl Pts',(-6.36691474847379,15.7297904840163,8.07499681619367));
#49949=CARTESIAN_POINT('Ctrl Pts',(-4.59005542323444,13.5564806545976,7.91799668884141));
#49950=CARTESIAN_POINT('Ctrl Pts',(-5.42257131653894,10.8755438858135,7.76099656148916));
#49951=CARTESIAN_POINT('Ctrl Pts',(-8.11793744062105,10.0910018961859,7.6039964341369));
#49952=CARTESIAN_POINT('Ctrl Pts',(-10.2591931327486,11.9063610164495,7.44699630678465));
#49953=CARTESIAN_POINT('Ctrl Pts',(-9.92625387366264,14.6937713043528,7.2899961794324));
#49954=CARTESIAN_POINT('Ctrl Pts',(-7.41766948685395,15.953735219701,7.13299605208014));
#49955=CARTESIAN_POINT('Ctrl Pts',(-4.98291166647307,14.5564310201707,6.97599592472789));
#49956=CARTESIAN_POINT('Ctrl Pts',(-4.80525109196198,11.7548348097635,6.81899579737564));
#49957=CARTESIAN_POINT('Ctrl Pts',(-7.04399773638617,10.061164742401,6.66199567002339));
#49958=CARTESIAN_POINT('Ctrl Pts',(-9.69164594449512,10.9941511043189,6.50499554267113));
#49959=CARTESIAN_POINT('Ctrl Pts',(-10.3740242882686,13.7171759009976,6.34799541531889));
#49960=CARTESIAN_POINT('Ctrl Pts',(-8.47923732450549,15.7884770124268,6.19099528796661));
#49961=CARTESIAN_POINT('Ctrl Pts',(-5.70635916288519,15.3506981982192,6.03399516061438));
#49962=CARTESIAN_POINT('Ctrl Pts',(-4.54185534982472,12.7964012172524,5.87699503326211));
#49963=CARTESIAN_POINT('Ctrl Pts',(-6.02994939266268,10.4160461410637,5.71999490590986));
#49964=CARTESIAN_POINT('Ctrl Pts',(-8.83624963123305,10.3441251642037,5.56299477855761));
#49965=CARTESIAN_POINT('Ctrl Pts',(-10.4443264801503,12.6451208096654,5.40599465120535));
#49966=CARTESIAN_POINT('Ctrl Pts',(-9.41218877466708,15.2557271980297,5.24899452385311));
#49967=CARTESIAN_POINT('Ctrl Pts',(-6.66539017469168,15.834951382638,5.09199439650085));
#49968=CARTESIAN_POINT('Ctrl Pts',(-4.66696070971034,13.863470166724,4.9349942691486));
#49969=CARTESIAN_POINT('Ctrl Pts',(-5.20901029900842,11.1089874665202,4.77799414179634));
#49970=CARTESIAN_POINT('Ctrl Pts',(-7.8052841019297,10.0417525531808,4.62099401444409));
#49971=CARTESIAN_POINT('Ctrl Pts',(-10.128057595771,11.6182209055488,4.46399388709184));
#49972=CARTESIAN_POINT('Ctrl Pts',(-10.093735767433,14.4258233247707,4.30699375973958));
#49973=CARTESIAN_POINT('Ctrl Pts',(-7.73454710646218,15.9448696981551,4.14999363238733));
#49974=CARTESIAN_POINT('Ctrl Pts',(-5.16315153543426,14.8173229408266,3.99299350503507));
#49975=CARTESIAN_POINT('Ctrl Pts',(-4.69098902991507,12.045960940047,3.83599337768282));
#49976=CARTESIAN_POINT('Ctrl Pts',(-6.05008049550023,10.7720932116963,3.73132662611465));
#49977=CARTESIAN_POINT('Ctrl Pts',(-6.84980000202491,10.5582942547315,3.67899325033057));
#49978=CARTESIAN_POINT('Ctrl Pts',(-5.44566844965789,14.7468063779934,12.1070022498898));
#49979=CARTESIAN_POINT('Ctrl Pts',(-4.86812015246569,14.0713004658265,12.0546688741057));
#49980=CARTESIAN_POINT('Ctrl Pts',(-4.44032807310083,12.1176993038908,11.9500021225376));
#49981=CARTESIAN_POINT('Ctrl Pts',(-6.54346469885977,9.95282118939152,11.7930019951853));
#49982=CARTESIAN_POINT('Ctrl Pts',(-9.50426845016806,10.5189740011564,11.6360018678331));
#49983=CARTESIAN_POINT('Ctrl Pts',(-10.6678138328376,13.2977029522207,11.4790017404808));
#49984=CARTESIAN_POINT('Ctrl Pts',(-8.99076038754082,15.8026598219827,11.3220016131285));
#49985=CARTESIAN_POINT('Ctrl Pts',(-5.97692217562184,15.7848971577712,11.1650014857763));
#49986=CARTESIAN_POINT('Ctrl Pts',(-4.32884537294989,13.2617363588805,11.008001358424));
#49987=CARTESIAN_POINT('Ctrl Pts',(-5.52437185495265,10.4950077843859,10.8510012310718));
#49988=CARTESIAN_POINT('Ctrl Pts',(-8.49146381092469,9.96602748253219,10.6940011037195));
#49989=CARTESIAN_POINT('Ctrl Pts',(-10.5695002659417,12.1489511132149,10.5370009763673));
#49990=CARTESIAN_POINT('Ctrl Pts',(-9.89508658439861,15.0864252137885,10.380000849015));
#49991=CARTESIAN_POINT('Ctrl Pts',(-7.07297568330216,16.144339968164,10.2230007216628));
#49992=CARTESIAN_POINT('Ctrl Pts',(-4.63378163576147,14.3740779132334,10.0660005943105));
#49993=CARTESIAN_POINT('Ctrl Pts',(-4.76475306606344,11.3630373167398,9.90900046695826));
#49994=CARTESIAN_POINT('Ctrl Pts',(-7.34844667640581,9.81125365971957,9.75200033960601));
#49995=CARTESIAN_POINT('Ctrl Pts',(-10.068039598996,11.1102229164483,9.59500021225375));
#49996=CARTESIAN_POINT('Ctrl Pts',(-10.4848467800654,14.0951485887035,9.43800008490151));
#49997=CARTESIAN_POINT('Ctrl Pts',(-8.22511321630987,16.0894183231763,9.28099995754925));
#49998=CARTESIAN_POINT('Ctrl Pts',(-5.31516367599608,15.3047517599283,9.12399983019699));
#49999=CARTESIAN_POINT('Ctrl Pts',(-4.36437782731425,12.4447667074727,8.96699970284474));
#50000=CARTESIAN_POINT('Ctrl Pts',(-6.22533446291578,10.0740393155813,8.80999957549249));
#50001=CARTESIAN_POINT('Ctrl Pts',(-9.22929591409124,10.3184235210999,8.65299944814023));
#50002=CARTESIAN_POINT('Ctrl Pts',(-10.6825811290368,12.9587776927019,8.49599932078798));
#50003=CARTESIAN_POINT('Ctrl Pts',(-9.28201531326903,15.6274708987809,8.33899919343573));
#50004=CARTESIAN_POINT('Ctrl Pts',(-6.2834992701754,15.9314603471809,8.18199906608347));
#50005=CARTESIAN_POINT('Ctrl Pts',(-4.37583110219086,13.5981557789132,8.02499893873123));
#50006=CARTESIAN_POINT('Ctrl Pts',(-5.26963515659132,10.7198537875612,7.86799881137897));
#50007=CARTESIAN_POINT('Ctrl Pts',(-8.16342876362473,9.87755538002796,7.71099868402671));
#50008=CARTESIAN_POINT('Ctrl Pts',(-10.4623194328887,11.8265576212272,7.55399855667447));
#50009=CARTESIAN_POINT('Ctrl Pts',(-10.1048698490028,14.8191715000043,7.39699842932221));
#50010=CARTESIAN_POINT('Ctrl Pts',(-7.4116084785376,16.1718914480481,7.23999830196995));
#50011=CARTESIAN_POINT('Ctrl Pts',(-4.79760863920515,14.6717204977811,7.0829981746177));
#50012=CARTESIAN_POINT('Ctrl Pts',(-4.60686904722592,11.6638763571539,6.92599804726545));
#50013=CARTESIAN_POINT('Ctrl Pts',(-7.01042775842265,9.84552167443846,6.7689979199132));
#50014=CARTESIAN_POINT('Ctrl Pts',(-9.85299055159733,10.8471926331423,6.61199779256093));
#50015=CARTESIAN_POINT('Ctrl Pts',(-10.585604229252,13.770681089133,6.4549976652087));
#50016=CARTESIAN_POINT('Ctrl Pts',(-8.55132682499211,15.9944672608673,6.29799753785643));
#50017=CARTESIAN_POINT('Ctrl Pts',(-5.57431489867653,15.5244600427274,6.14099741050419));
#50018=CARTESIAN_POINT('Ctrl Pts',(-4.32408263542585,12.7821208080144,5.98399728315193));
#50019=CARTESIAN_POINT('Ctrl Pts',(-5.92172719634629,10.2265287344922,5.82699715579967));
#50020=CARTESIAN_POINT('Ctrl Pts',(-8.93462166631621,10.149313078634,5.66999702844742));
#50021=CARTESIAN_POINT('Ctrl Pts',(-10.6610819284076,12.61970343828,5.51299690109516));
#50022=CARTESIAN_POINT('Ctrl Pts',(-9.55296030180576,15.4224974667542,5.35599677374291));
#50023=CARTESIAN_POINT('Ctrl Pts',(-6.60394786249421,16.0443629816032,5.19899664639066));
#50024=CARTESIAN_POINT('Ctrl Pts',(-4.45839800260659,13.927745247179,5.04199651903841));
#50025=CARTESIAN_POINT('Ctrl Pts',(-5.04035220251703,10.9704830194925,4.88499639168615));
#50026=CARTESIAN_POINT('Ctrl Pts',(-7.82775850916875,9.82468039853088,4.7279962643339));
#50027=CARTESIAN_POINT('Ctrl Pts',(-10.3215299589949,11.5172052095439,4.57099613698165));
#50028=CARTESIAN_POINT('Ctrl Pts',(-10.2846814260484,14.53149772411,4.41399600962939));
#50029=CARTESIAN_POINT('Ctrl Pts',(-7.75181399705376,16.1623732644724,4.25699588227714));
#50030=CARTESIAN_POINT('Ctrl Pts',(-4.99111740815211,14.9518187617518,4.09999575492489));
#50031=CARTESIAN_POINT('Ctrl Pts',(-4.48419523986314,11.9764346130167,3.94299562757263));
#50032=CARTESIAN_POINT('Ctrl Pts',(-5.94334031085913,10.6087872809636,3.83832887600446));
#50033=CARTESIAN_POINT('Ctrl Pts',(-6.80193357383899,10.379248870828,3.78599550022038));
#50034=CARTESIAN_POINT('Ctrl Pts',(-5.30480289598085,14.8672444958453,12.2140044997796));
#50035=CARTESIAN_POINT('Ctrl Pts',(-4.68765210100993,14.1454191303684,12.1616711239955));
#50036=CARTESIAN_POINT('Ctrl Pts',(-4.23052631058544,12.0578594994142,12.0570043724274));
#50037=CARTESIAN_POINT('Ctrl Pts',(-6.47787505497571,9.74453565122039,11.9000042450751));
#50038=CARTESIAN_POINT('Ctrl Pts',(-9.64170117610916,10.3495095721105,11.7430041177229));
#50039=CARTESIAN_POINT('Ctrl Pts',(-10.8850308879103,13.3187760204667,11.5860039903706));
#50040=CARTESIAN_POINT('Ctrl Pts',(-9.09298185581149,15.9954978306723,11.4290038630184));
#50041=CARTESIAN_POINT('Ctrl Pts',(-5.87248470008946,15.9765171802363,11.2720037356661));
#50042=CARTESIAN_POINT('Ctrl Pts',(-4.11139923955409,13.2803431971336,11.1150036083138));
#50043=CARTESIAN_POINT('Ctrl Pts',(-5.38890299528115,10.3238999913978,10.9580034809616));
#50044=CARTESIAN_POINT('Ctrl Pts',(-8.55944850339236,9.75864750013418,10.8010033536093));
#50045=CARTESIAN_POINT('Ctrl Pts',(-10.7799759578531,12.091254245901,10.6440032262571));
#50046=CARTESIAN_POINT('Ctrl Pts',(-10.0593177172747,15.230151001703,10.4870030989048));
#50047=CARTESIAN_POINT('Ctrl Pts',(-7.04369461774331,16.3606069910088,10.3300029715526));
#50048=CARTESIAN_POINT('Ctrl Pts',(-4.43724498773573,14.4689580331317,10.1730028442003));
#50049=CARTESIAN_POINT('Ctrl Pts',(-4.57719713151714,11.2514503253782,10.0160027168481));
#50050=CARTESIAN_POINT('Ctrl Pts',(-7.33805466210989,9.59326083333269,9.85900258949581));
#50051=CARTESIAN_POINT('Ctrl Pts',(-10.2441301233891,10.9813004368261,9.70200246214358));
#50052=CARTESIAN_POINT('Ctrl Pts',(-10.689517780832,14.1709025194869,9.5450023347913));
#50053=CARTESIAN_POINT('Ctrl Pts',(-8.27483424341331,16.3019193677744,9.38800220743907));
#50054=CARTESIAN_POINT('Ctrl Pts',(-5.16534940749437,15.463448203285,9.2310020800868));
#50055=CARTESIAN_POINT('Ctrl Pts',(-4.14936815499344,12.4073539211118,9.07400195273456));
#50056=CARTESIAN_POINT('Ctrl Pts',(-6.13793062267174,9.87406570664018,8.9170018253823));
#50057=CARTESIAN_POINT('Ctrl Pts',(-9.34787376797726,10.1352073418028,8.76000169803005));
#50058=CARTESIAN_POINT('Ctrl Pts',(-10.9008107778922,12.9566106494239,8.6030015706778));
#50059=CARTESIAN_POINT('Ctrl Pts',(-9.40420813736444,15.8082961996578,8.44600144332554));
#50060=CARTESIAN_POINT('Ctrl Pts',(-6.20008379187702,16.1331302103455,8.28900131597328));
#50061=CARTESIAN_POINT('Ctrl Pts',(-4.16160678114728,13.6398309032289,8.13200118862104));
#50062=CARTESIAN_POINT('Ctrl Pts',(-5.1166989966437,10.564163689309,7.97500106126877));
#50063=CARTESIAN_POINT('Ctrl Pts',(-8.20892008662842,9.66410886387002,7.81800093391653));
#50064=CARTESIAN_POINT('Ctrl Pts',(-10.6654457330288,11.7467542260049,7.66100080656427));
#50065=CARTESIAN_POINT('Ctrl Pts',(-10.2834858243429,14.9445716956558,7.50400067921202));
#50066=CARTESIAN_POINT('Ctrl Pts',(-7.40554747022126,16.3900476763952,7.34700055185976));
#50067=CARTESIAN_POINT('Ctrl Pts',(-4.61230561193723,14.7870099753915,7.19000042450751));
#50068=CARTESIAN_POINT('Ctrl Pts',(-4.40848700248986,11.5729179045444,7.03300029715526));
#50069=CARTESIAN_POINT('Ctrl Pts',(-6.97685778045915,9.6298786064759,6.876000169803));
#50070=CARTESIAN_POINT('Ctrl Pts',(-10.0143351586995,10.7002341619658,6.71900004245076));
#50071=CARTESIAN_POINT('Ctrl Pts',(-10.7971841702354,13.8241862772684,6.5619999150985));
#50072=CARTESIAN_POINT('Ctrl Pts',(-8.62341632547871,16.2004575093079,6.40499978774625));
#50073=CARTESIAN_POINT('Ctrl Pts',(-5.44227063446788,15.6982218872355,6.24799966039399));
#50074=CARTESIAN_POINT('Ctrl Pts',(-4.10630992102698,12.7678403987764,6.09099953304174));
#50075=CARTESIAN_POINT('Ctrl Pts',(-5.81350500002991,10.0370113279208,5.93399940568948));
#50076=CARTESIAN_POINT('Ctrl Pts',(-9.03299370139936,9.95450099306433,5.77699927833723));
#50077=CARTESIAN_POINT('Ctrl Pts',(-10.877837376665,12.5942860668946,5.61999915098498));
#50078=CARTESIAN_POINT('Ctrl Pts',(-9.69373182894443,15.5892677354788,5.46299902363273));
#50079=CARTESIAN_POINT('Ctrl Pts',(-6.54250555029675,16.2537745805684,5.30599889628047));
#50080=CARTESIAN_POINT('Ctrl Pts',(-4.24983529550283,13.9920203276339,5.14899876892821));
#50081=CARTESIAN_POINT('Ctrl Pts',(-4.87169410602564,10.8319785724647,4.99199864157597));
#50082=CARTESIAN_POINT('Ctrl Pts',(-7.85023291640778,9.60760824388092,4.83499851422371));
#50083=CARTESIAN_POINT('Ctrl Pts',(-10.5150023222189,11.416189513539,4.67799838687146));
#50084=CARTESIAN_POINT('Ctrl Pts',(-10.4756270846638,14.6371721234493,4.52099825951921));
#50085=CARTESIAN_POINT('Ctrl Pts',(-7.76908088764536,16.3798768307898,4.36399813216695));
#50086=CARTESIAN_POINT('Ctrl Pts',(-4.81908328086994,15.086314582677,4.2069980048147));
#50087=CARTESIAN_POINT('Ctrl Pts',(-4.27740144981121,11.9069082859864,4.04999787746244));
#50088=CARTESIAN_POINT('Ctrl Pts',(-5.83660012621804,10.4454813502308,3.94533112589427));
#50089=CARTESIAN_POINT('Ctrl Pts',(-6.75406714565307,10.2002034869244,3.89299775011019));
#50090=CARTESIAN_POINT('Ctrl Pts',(-5.16393734230382,14.9876826136972,12.3210067496694));
#50091=CARTESIAN_POINT('Ctrl Pts',(-4.50718404955416,14.2195377949102,12.2686733738853));
#50092=CARTESIAN_POINT('Ctrl Pts',(-4.02072454807007,11.9980196949375,12.1640066223172));
#50093=CARTESIAN_POINT('Ctrl Pts',(-6.41228541109164,9.53625011304927,12.0070064949649));
#50094=CARTESIAN_POINT('Ctrl Pts',(-9.77913390205027,10.1800451430645,11.8500063676127));
#50095=CARTESIAN_POINT('Ctrl Pts',(-11.1022479429831,13.3398490887126,11.6930062402604));
#50096=CARTESIAN_POINT('Ctrl Pts',(-9.19520332408216,16.188335839362,11.5360061129082));
#50097=CARTESIAN_POINT('Ctrl Pts',(-5.76804722455709,16.1681372027015,11.3790059855559));
#50098=CARTESIAN_POINT('Ctrl Pts',(-3.89395310615829,13.2989500353867,11.2220058582037));
#50099=CARTESIAN_POINT('Ctrl Pts',(-5.25343413560966,10.1527921984098,11.0650057308514));
#50100=CARTESIAN_POINT('Ctrl Pts',(-8.62743319586002,9.55126751773617,10.9080056034992));
#50101=CARTESIAN_POINT('Ctrl Pts',(-10.9904516497645,12.0335573785871,10.7510054761469));
#50102=CARTESIAN_POINT('Ctrl Pts',(-10.2235488501508,15.3738767896174,10.5940053487946));
#50103=CARTESIAN_POINT('Ctrl Pts',(-7.01441355218445,16.5768740138536,10.4370052214424));
#50104=CARTESIAN_POINT('Ctrl Pts',(-4.24070833971001,14.56383815303,10.2800050940901));
#50105=CARTESIAN_POINT('Ctrl Pts',(-4.38964119697082,11.1398633340167,10.1230049667379));
#50106=CARTESIAN_POINT('Ctrl Pts',(-7.32766264781398,9.3752680069458,9.96600483938563));
#50107=CARTESIAN_POINT('Ctrl Pts',(-10.4202206477823,10.8523779572038,9.80900471203337));
#50108=CARTESIAN_POINT('Ctrl Pts',(-10.8941887815987,14.2466564502702,9.65200458468113));
#50109=CARTESIAN_POINT('Ctrl Pts',(-8.32455527051676,16.5144204123725,9.49500445732887));
#50110=CARTESIAN_POINT('Ctrl Pts',(-5.01553513899265,15.6221446466417,9.33800432997661));
#50111=CARTESIAN_POINT('Ctrl Pts',(-3.93435848267263,12.3699411347509,9.18100420262437));
#50112=CARTESIAN_POINT('Ctrl Pts',(-6.0505267824277,9.67409209769908,9.02400407527211));
#50113=CARTESIAN_POINT('Ctrl Pts',(-9.46645162186327,9.95199116250562,8.86700394791985));
#50114=CARTESIAN_POINT('Ctrl Pts',(-11.1190404267477,12.9544436061459,8.71000382056761));
#50115=CARTESIAN_POINT('Ctrl Pts',(-9.52640096145984,15.9891215005347,8.55300369321535));
#50116=CARTESIAN_POINT('Ctrl Pts',(-6.11666831357863,16.3348000735102,8.3960035658631));
#50117=CARTESIAN_POINT('Ctrl Pts',(-3.9473824601037,13.6815060275445,8.23900343851085));
#50118=CARTESIAN_POINT('Ctrl Pts',(-4.9637628366961,10.4084735910568,8.08200331115859));
#50119=CARTESIAN_POINT('Ctrl Pts',(-8.25441140963209,9.45066234771208,7.92500318380633));
#50120=CARTESIAN_POINT('Ctrl Pts',(-10.8685720331689,11.6669508307826,7.76800305645408));
#50121=CARTESIAN_POINT('Ctrl Pts',(-10.4621017996831,15.0699718913073,7.61100292910183));
#50122=CARTESIAN_POINT('Ctrl Pts',(-7.39948646190492,16.6082039047423,7.45400280174958));
#50123=CARTESIAN_POINT('Ctrl Pts',(-4.42700258466931,14.902299453002,7.29700267439732));
#50124=CARTESIAN_POINT('Ctrl Pts',(-4.21010495775379,11.4819594519348,7.14000254704507));
#50125=CARTESIAN_POINT('Ctrl Pts',(-6.94328780249567,9.41423553851335,6.98300241969282));
#50126=CARTESIAN_POINT('Ctrl Pts',(-10.1756797658017,10.5532756907892,6.82600229234056));
#50127=CARTESIAN_POINT('Ctrl Pts',(-11.0087641112188,13.8776914654038,6.66900216498831));
#50128=CARTESIAN_POINT('Ctrl Pts',(-8.69550582596531,16.4064477577484,6.51200203763606));
#50129=CARTESIAN_POINT('Ctrl Pts',(-5.31022637025923,15.8719837317436,6.3550019102838));
#50130=CARTESIAN_POINT('Ctrl Pts',(-3.88853720662811,12.7535599895385,6.19800178293155));
#50131=CARTESIAN_POINT('Ctrl Pts',(-5.70528280371351,9.84749392134933,6.04100165557929));
#50132=CARTESIAN_POINT('Ctrl Pts',(-9.13136573648253,9.75968890749465,5.88400152822705));
#50133=CARTESIAN_POINT('Ctrl Pts',(-11.0945928249223,12.5688686955092,5.72700140087479));
#50134=CARTESIAN_POINT('Ctrl Pts',(-9.83450335608313,15.7560380042034,5.57000127352253));
#50135=CARTESIAN_POINT('Ctrl Pts',(-6.48106323809927,16.4631861795336,5.41300114617029));
#50136=CARTESIAN_POINT('Ctrl Pts',(-4.04127258839909,14.0562954080889,5.25600101881802));
#50137=CARTESIAN_POINT('Ctrl Pts',(-4.70303600953422,10.693474125437,5.09900089146578));
#50138=CARTESIAN_POINT('Ctrl Pts',(-7.87270732364685,9.390536089231,4.94200076411351));
#50139=CARTESIAN_POINT('Ctrl Pts',(-10.7084746854428,11.3151738175341,4.78500063676127));
#50140=CARTESIAN_POINT('Ctrl Pts',(-10.6665727432792,14.7428465227886,4.62800050940901));
#50141=CARTESIAN_POINT('Ctrl Pts',(-7.78634777823694,16.5973803971072,4.47100038205676));
#50142=CARTESIAN_POINT('Ctrl Pts',(-4.64704915358778,15.2208104036021,4.31400025470451));
#50143=CARTESIAN_POINT('Ctrl Pts',(-4.07060765975928,11.8373819589561,4.15700012735225));
#50144=CARTESIAN_POINT('Ctrl Pts',(-5.72985994157694,10.2821754194981,4.05233337578409));
#50145=CARTESIAN_POINT('Ctrl Pts',(-6.70620071746715,10.0211581030209,4.));
#50146=CARTESIAN_POINT('Ctrl Pts',(-5.58653400333492,14.6263682601415,12.));
#50147=CARTESIAN_POINT('Ctrl Pts',(-5.52489667247578,14.5684443043264,12.));
#50148=CARTESIAN_POINT('Ctrl Pts',(-5.46662450511892,14.5073716307993,12.));
#50149=CARTESIAN_POINT('Ctrl Pts',(-5.41171706416437,14.4435345397783,12.));
#50150=CARTESIAN_POINT('Ctrl Pts',(-5.35535922399003,14.3780111697138,12.));
#50151=CARTESIAN_POINT('Ctrl Pts',(-5.30254577876706,14.3095749751578,12.));
#50152=CARTESIAN_POINT('Ctrl Pts',(-5.25330168675279,14.2385929714213,12.));
#50153=CARTESIAN_POINT('Ctrl Pts',(-5.20312907342738,14.1662725674732,12.));
#50154=CARTESIAN_POINT('Ctrl Pts',(-5.15666120991867,14.0913088475707,12.));
#50155=CARTESIAN_POINT('Ctrl Pts',(-5.1139575408143,14.0140482152174,12.));
#50156=CARTESIAN_POINT('Ctrl Pts',(-5.09461512222896,13.9790533887192,12.));
#50157=CARTESIAN_POINT('Ctrl Pts',(-5.07604545116087,13.9435868239722,12.));
#50158=CARTESIAN_POINT('Ctrl Pts',(-5.05825663128179,13.9076784991748,12.));
#50159=CARTESIAN_POINT('Ctrl Pts',(-5.04815176560046,13.887280923541,12.));
#50160=CARTESIAN_POINT('Ctrl Pts',(-5.03829889260597,13.8667407800149,12.));
#50161=CARTESIAN_POINT('Ctrl Pts',(-5.02869974914025,13.846063404379,12.));
#50162=CARTESIAN_POINT('Ctrl Pts',(-5.02048275827117,13.8283633035935,12.));
#50163=CARTESIAN_POINT('Ctrl Pts',(-5.0124495628302,13.8105575032607,12.));
#50164=CARTESIAN_POINT('Ctrl Pts',(-5.00461403680565,13.7926790499403,12.));
#50165=CARTESIAN_POINT('Ctrl Pts',(-4.96800796729637,13.7091543570335,12.));
#50166=CARTESIAN_POINT('Ctrl Pts',(-4.93566374876766,13.6239462866792,12.));
#50167=CARTESIAN_POINT('Ctrl Pts',(-4.90760852459924,13.5374526993157,12.));
#50168=CARTESIAN_POINT('Ctrl Pts',(-4.87909391214457,13.449542828816,12.));
#50169=CARTESIAN_POINT('Ctrl Pts',(-4.85500940725962,13.3603042433618,12.));
#50170=CARTESIAN_POINT('Ctrl Pts',(-4.83542253240114,13.2701175707646,12.));
#50171=CARTESIAN_POINT('Ctrl Pts',(-4.81671792757447,13.1839932613098,12.));
#50172=CARTESIAN_POINT('Ctrl Pts',(-4.80211484736484,13.0970034290495,12.));
#50173=CARTESIAN_POINT('Ctrl Pts',(-4.79171068325589,13.0094587764721,12.));
#50174=CARTESIAN_POINT('Ctrl Pts',(-4.78712088419529,12.9708384356209,12.));
#50175=CARTESIAN_POINT('Ctrl Pts',(-4.78334877386587,12.9321099201028,12.));
#50176=CARTESIAN_POINT('Ctrl Pts',(-4.78040530851934,12.893299212279,12.));
#50177=CARTESIAN_POINT('Ctrl Pts',(-4.77903296806464,12.8752043824944,12.));
#50178=CARTESIAN_POINT('Ctrl Pts',(-4.77784077628839,12.8570916824141,12.));
#50179=CARTESIAN_POINT('Ctrl Pts',(-4.77682996946529,12.8389637304098,12.));
#50180=CARTESIAN_POINT('Ctrl Pts',(-4.77585594563052,12.8214954497015,12.));
#50181=CARTESIAN_POINT('Ctrl Pts',(-4.7750503477527,12.8040101811658,12.));
#50182=CARTESIAN_POINT('Ctrl Pts',(-4.77441493543858,12.7865348449805,12.));
#50183=CARTESIAN_POINT('Ctrl Pts',(-4.77095144017316,12.6912805623749,12.));
#50184=CARTESIAN_POINT('Ctrl Pts',(-4.77253057533756,12.5961742600887,12.));
#50185=CARTESIAN_POINT('Ctrl Pts',(-4.77921451714525,12.501614579937,12.));
#50186=CARTESIAN_POINT('Ctrl Pts',(-4.78586350142022,12.4075494542275,12.));
#50187=CARTESIAN_POINT('Ctrl Pts',(-4.7975636844451,12.3140242926481,12.));
#50188=CARTESIAN_POINT('Ctrl Pts',(-4.81442425859455,12.2214137249389,12.));
#50189=CARTESIAN_POINT('Ctrl Pts',(-4.83092299201404,12.1307906503674,12.));
#50190=CARTESIAN_POINT('Ctrl Pts',(-4.85236265681916,12.0410424028911,12.));
#50191=CARTESIAN_POINT('Ctrl Pts',(-4.87846866601438,11.9524107169388,12.));
#50192=CARTESIAN_POINT('Ctrl Pts',(-4.89379308908251,11.9003832529699,12.));
#50193=CARTESIAN_POINT('Ctrl Pts',(-4.91072644984389,11.8487405476717,12.));
#50194=CARTESIAN_POINT('Ctrl Pts',(-4.92922132646561,11.7975326456,12.));
#50195=CARTESIAN_POINT('Ctrl Pts',(-4.93398223972469,11.7843508123318,12.));
#50196=CARTESIAN_POINT('Ctrl Pts',(-4.93884748217419,11.7711956209025,12.));
#50197=CARTESIAN_POINT('Ctrl Pts',(-4.94381359460063,11.7580750750315,12.));
#50198=CARTESIAN_POINT('Ctrl Pts',(-4.97686200318078,11.6707606682067,12.));
#50199=CARTESIAN_POINT('Ctrl Pts',(-5.01429316281797,11.5851876670551,12.));
#50200=CARTESIAN_POINT('Ctrl Pts',(-5.05577609967284,11.5015918684293,12.));
#50201=CARTESIAN_POINT('Ctrl Pts',(-5.09882544403038,11.414839468654,12.));
#50202=CARTESIAN_POINT('Ctrl Pts',(-5.14623844362019,11.330215691903,12.));
#50203=CARTESIAN_POINT('Ctrl Pts',(-5.19770129474244,11.2479859989681,12.));
#50204=CARTESIAN_POINT('Ctrl Pts',(-5.2497890294851,11.1647578384569,12.));
#50205=CARTESIAN_POINT('Ctrl Pts',(-5.30602595623937,11.0839814330439,12.));
#50206=CARTESIAN_POINT('Ctrl Pts',(-5.36613892032226,11.0059457826021,12.));
#50207=CARTESIAN_POINT('Ctrl Pts',(-5.4056128756235,10.9547026635106,12.));
#50208=CARTESIAN_POINT('Ctrl Pts',(-5.44675926231209,10.9046416780186,12.));
#50209=CARTESIAN_POINT('Ctrl Pts',(-5.48951145353165,10.8558504805206,12.));
#50210=CARTESIAN_POINT('Ctrl Pts',(-5.50097088386534,10.8427723361571,12.));
#50211=CARTESIAN_POINT('Ctrl Pts',(-5.5125457300662,10.8297854541688,12.));
#50212=CARTESIAN_POINT('Ctrl Pts',(-5.52423480193837,10.8168915966514,12.));
#50213=CARTESIAN_POINT('Ctrl Pts',(-5.53538763239833,10.8045892506277,12.));
#50214=CARTESIAN_POINT('Ctrl Pts',(-5.54663877351141,10.7923778862678,12.));
#50215=CARTESIAN_POINT('Ctrl Pts',(-5.55798379608792,10.7802620173577,12.));
#50216=CARTESIAN_POINT('Ctrl Pts',(-5.62980564817047,10.7035601739863,12.));
#50217=CARTESIAN_POINT('Ctrl Pts',(-5.70542329107336,10.630641847274,12.));
#50218=CARTESIAN_POINT('Ctrl Pts',(-5.78449319659024,10.5618401471187,12.));
#50219=CARTESIAN_POINT('Ctrl Pts',(-5.84379562572791,10.5102388720023,12.));
#50220=CARTESIAN_POINT('Ctrl Pts',(-5.90504126576837,10.4609534569649,12.));
#50221=CARTESIAN_POINT('Ctrl Pts',(-5.96810424452339,10.4141359861561,12.));
#50222=CARTESIAN_POINT('Ctrl Pts',(-5.99074689198795,10.39732625868,12.));
#50223=CARTESIAN_POINT('Ctrl Pts',(-6.01362396161954,10.3808348014861,12.));
#50224=CARTESIAN_POINT('Ctrl Pts',(-6.03673007192386,10.3646690702049,12.));
#50225=CARTESIAN_POINT('Ctrl Pts',(-6.05604446520068,10.351156138454,12.));
#50226=CARTESIAN_POINT('Ctrl Pts',(-6.07552143283976,10.3378692705033,12.));
#50227=CARTESIAN_POINT('Ctrl Pts',(-6.09513718668148,10.3248263089414,12.));
#50228=CARTESIAN_POINT('Ctrl Pts',(-6.18010809783264,10.2683272145418,12.));
#50229=CARTESIAN_POINT('Ctrl Pts',(-6.26775573276173,10.2163476819429,12.));
#50230=CARTESIAN_POINT('Ctrl Pts',(-6.35779277794461,10.1691997545039,12.));
#50231=CARTESIAN_POINT('Ctrl Pts',(-6.4298686728608,10.131457189133,12.));
#50232=CARTESIAN_POINT('Ctrl Pts',(-6.50347672461637,10.0968111469865,12.));
#50233=CARTESIAN_POINT('Ctrl Pts',(-6.57848633664494,10.0654390261441,12.));
#50234=CARTESIAN_POINT('Ctrl Pts',(-6.61998971216275,10.0480805986452,12.));
#50235=CARTESIAN_POINT('Ctrl Pts',(-6.6619224176942,10.0317247798523,12.));
#50236=CARTESIAN_POINT('Ctrl Pts',(-6.70425100699966,10.0163623331919,12.));
#50237=CARTESIAN_POINT('Ctrl Pts',(-10.0166112816083,12.988245230306,10.387416697508));
#50238=CARTESIAN_POINT('Ctrl Pts',(-10.0185036739199,12.7635802052187,10.4016107071645));
#50239=CARTESIAN_POINT('Ctrl Pts',(-9.99083720988162,12.539373330507,10.415804716821));
#50240=CARTESIAN_POINT('Ctrl Pts',(-9.93173881101679,12.3237831354866,10.4299987264775));
#50241=CARTESIAN_POINT('Ctrl Pts',(-9.71384275550587,11.5289011419959,10.4823321022615));
#50242=CARTESIAN_POINT('Ctrl Pts',(-9.06866093698144,10.8511543034631,10.5346654780456));
#50243=CARTESIAN_POINT('Ctrl Pts',(-8.28546362708042,10.5943989029373,10.5869988538297));
#50244=CARTESIAN_POINT('Ctrl Pts',(-7.50226631717939,10.3376435024115,10.6393322296138));
#50245=CARTESIAN_POINT('Ctrl Pts',(-6.58105351590176,10.5018795398927,10.6916656053979));
#50246=CARTESIAN_POINT('Ctrl Pts',(-5.93485558054988,11.0134998825089,10.743998981182));
#50247=CARTESIAN_POINT('Ctrl Pts',(-5.28865764519799,11.5251202251251,10.796332356966));
#50248=CARTESIAN_POINT('Ctrl Pts',(-4.91747457577184,12.3841248728762,10.8486657327501));
#50249=CARTESIAN_POINT('Ctrl Pts',(-4.98772773186019,13.2053184658649,10.9009991085342));
#50250=CARTESIAN_POINT('Ctrl Pts',(-5.05798088794854,14.0265120588536,10.9533324843183));
#50251=CARTESIAN_POINT('Ctrl Pts',(-5.56967026955137,14.8098945970798,11.0056658601024));
#50252=CARTESIAN_POINT('Ctrl Pts',(-6.29337817170545,15.2043433125241,11.0579992358865));
#50253=CARTESIAN_POINT('Ctrl Pts',(-7.01708607385953,15.5987920279684,11.1103326116706));
#50254=CARTESIAN_POINT('Ctrl Pts',(-7.95281249656485,15.6043069206307,11.1626659874546));
#50255=CARTESIAN_POINT('Ctrl Pts',(-8.68101868433327,15.2181990454088,11.2149993632387));
#50256=CARTESIAN_POINT('Ctrl Pts',(-9.4092248721017,14.8320911701869,11.2673327390228));
#50257=CARTESIAN_POINT('Ctrl Pts',(-9.92991082493323,14.0543605270808,11.3196661148069));
#50258=CARTESIAN_POINT('Ctrl Pts',(-10.0096269590927,13.2341299632324,11.371999490591));
#50259=CARTESIAN_POINT('Ctrl Pts',(-10.0174549790803,13.1535843959402,11.3771385595633));
#50260=CARTESIAN_POINT('Ctrl Pts',(-10.0210307346825,13.0726290026425,11.3822776285357));
#50261=CARTESIAN_POINT('Ctrl Pts',(-10.020507596494,12.9916292754481,11.387416697508));
#50262=CARTESIAN_POINT('Ctrl Pts',(-8.29379928253292,10.0211581030209,12.));
#50263=CARTESIAN_POINT('Ctrl Pts',(-9.27014005842312,10.2821754194981,11.9476666242159));
#50264=CARTESIAN_POINT('Ctrl Pts',(-10.9293920526294,11.8373837255142,11.8429998726477));
#50265=CARTESIAN_POINT('Ctrl Pts',(-10.3529510979028,15.2208095229378,11.6859997452955));
#50266=CARTESIAN_POINT('Ctrl Pts',(-7.21365218567195,16.5973810760335,11.5289996179432));
#50267=CARTESIAN_POINT('Ctrl Pts',(-4.33342713054201,14.7428462583649,11.371999490591));
#50268=CARTESIAN_POINT('Ctrl Pts',(-4.29152522806557,11.3151739482887,11.2149993632387));
#50269=CARTESIAN_POINT('Ctrl Pts',(-7.12729264284838,9.39053585671186,11.0579992358865));
#50270=CARTESIAN_POINT('Ctrl Pts',(-10.2969641018483,10.6934741072896,10.9009991085342));
#50271=CARTESIAN_POINT('Ctrl Pts',(-10.9587275214881,14.0562954105675,10.743998981182));
#50272=CARTESIAN_POINT('Ctrl Pts',(-8.5189368031419,16.4631863186891,10.5869988538297));
#50273=CARTESIAN_POINT('Ctrl Pts',(-5.16549655959477,15.7560380892136,10.4299987264775));
#50274=CARTESIAN_POINT('Ctrl Pts',(-3.90540705298465,12.5688686867556,10.2729985991252));
#50275=CARTESIAN_POINT('Ctrl Pts',(-5.86863420589283,9.75968879265402,10.115998471773));
#50276=CARTESIAN_POINT('Ctrl Pts',(-9.29471725902464,9.84749381445728,9.9589983444207));
#50277=CARTESIAN_POINT('Ctrl Pts',(-11.1114629177913,12.7535599804133,9.80199821706845));
#50278=CARTESIAN_POINT('Ctrl Pts',(-9.68977370564798,15.8719838318464,9.64499808971619));
#50279=CARTESIAN_POINT('Ctrl Pts',(-6.30449413259093,16.4064478755407,9.48799796236394));
#50280=CARTESIAN_POINT('Ctrl Pts',(-3.99123576757957,13.8776914962184,9.3309978350117));
#50281=CARTESIAN_POINT('Ctrl Pts',(-4.82432014168349,10.5532756064786,9.17399770765943));
#50282=CARTESIAN_POINT('Ctrl Pts',(-8.05671221676616,9.41423541495656,9.0169975803072));
#50283=CARTESIAN_POINT('Ctrl Pts',(-10.7898951559407,11.481959399778,8.85999745295492));
#50284=CARTESIAN_POINT('Ctrl Pts',(-10.572997521546,14.902299519094,8.70299732560269));
#50285=CARTESIAN_POINT('Ctrl Pts',(-7.60051354156566,16.6082040297755,8.54599719825042));
#50286=CARTESIAN_POINT('Ctrl Pts',(-4.53789809794217,15.0699719631857,8.38899707089818));
#50287=CARTESIAN_POINT('Ctrl Pts',(-4.1314278504052,11.6669507850401,8.23199694354592));
#50288=CARTESIAN_POINT('Ctrl Pts',(-6.74558856429446,9.45066222537301,8.07499681619367));
#50289=CARTESIAN_POINT('Ctrl Pts',(-10.0362372509614,10.4084735018199,7.91799668884141));
#50290=CARTESIAN_POINT('Ctrl Pts',(-11.0526176626825,13.6815060514322,7.76099656148917));
#50291=CARTESIAN_POINT('Ctrl Pts',(-8.88333173423194,16.3348001890992,7.6039964341369));
#50292=CARTESIAN_POINT('Ctrl Pts',(-5.47359896850368,15.9891216041795,7.44699630678466));
#50293=CARTESIAN_POINT('Ctrl Pts',(-3.88095944817013,12.9544436048999,7.28999617943239));
#50294=CARTESIAN_POINT('Ctrl Pts',(-5.53354831017302,9.95199105749957,7.13299605208015));
#50295=CARTESIAN_POINT('Ctrl Pts',(-8.9494732676674,9.67409198306777,6.97599592472789));
#50296=CARTESIAN_POINT('Ctrl Pts',(-11.0656416405671,12.3699411133323,6.81899579737564));
#50297=CARTESIAN_POINT('Ctrl Pts',(-9.98446494686864,15.6221447375545,6.66199567002338));
#50298=CARTESIAN_POINT('Ctrl Pts',(-6.67544470099851,16.5144205342573,6.50499554267113));
#50299=CARTESIAN_POINT('Ctrl Pts',(-4.10581110106408,14.2466564935293,6.34799541531888));
#50300=CARTESIAN_POINT('Ctrl Pts',(-4.57977925134152,10.8523778836063,6.19099528796662));
#50301=CARTESIAN_POINT('Ctrl Pts',(-7.67233735803906,9.3752678814539,6.03399516061438));
#50302=CARTESIAN_POINT('Ctrl Pts',(-10.6103589107324,11.1398632710606,5.87699503326211));
#50303=CARTESIAN_POINT('Ctrl Pts',(-10.7592917725406,14.5638382055826,5.71999490590987));
#50304=CARTESIAN_POINT('Ctrl Pts',(-7.98558646537732,16.576874141135,5.56299477855761));
#50305=CARTESIAN_POINT('Ctrl Pts',(-4.77645105419042,15.3738768659897,5.40599465120536));
#50306=CARTESIAN_POINT('Ctrl Pts',(-4.00954823259222,12.0335573562934,5.24899452385311));
#50307=CARTESIAN_POINT('Ctrl Pts',(-6.37256675930357,9.55126737969704,5.09199439650085));
#50308=CARTESIAN_POINT('Ctrl Pts',(-9.74656595354479,10.1527921341227,4.9349942691486));
#50309=CARTESIAN_POINT('Ctrl Pts',(-11.1060469959117,13.2989499872504,4.77799414179634));
#50310=CARTESIAN_POINT('Ctrl Pts',(-9.2319528795399,16.1681374132995,4.62099401444409));
#50311=CARTESIAN_POINT('Ctrl Pts',(-5.80479653057489,16.1883357805992,4.46399388709183));
#50312=CARTESIAN_POINT('Ctrl Pts',(-3.89775210281319,13.3398493780975,4.30699375973959));
#50313=CARTESIAN_POINT('Ctrl Pts',(-5.22086568363505,10.1800446040033,4.14999363238733));
#50314=CARTESIAN_POINT('Ctrl Pts',(-8.58771529500726,9.53625069635182,3.99299350503508));
#50315=CARTESIAN_POINT('Ctrl Pts',(-10.9792742142571,11.9980184020288,3.83599337768282));
#50316=CARTESIAN_POINT('Ctrl Pts',(-10.4928159504458,14.2195377949103,3.73132662611465));
#50317=CARTESIAN_POINT('Ctrl Pts',(-9.83606265769613,14.9876826136973,3.67899325033057));
#50318=CARTESIAN_POINT('Ctrl Pts',(-8.245932854347,10.2002034869244,12.1070022498898));
#50319=CARTESIAN_POINT('Ctrl Pts',(-9.16339987378202,10.4454813502309,12.0546688741057));
#50320=CARTESIAN_POINT('Ctrl Pts',(-10.7225982799205,11.9069099460203,11.9500021225376));
#50321=CARTESIAN_POINT('Ctrl Pts',(-10.1809169554557,15.086313755117,11.7930019951853));
#50322=CARTESIAN_POINT('Ctrl Pts',(-7.23091907843985,16.3798774687766,11.636001867833));
#50323=CARTESIAN_POINT('Ctrl Pts',(-4.52437279676603,14.6371718749705,11.4790017404808));
#50324=CARTESIAN_POINT('Ctrl Pts',(-4.48499759650499,11.4161896364091,11.3220016131285));
#50325=CARTESIAN_POINT('Ctrl Pts',(-7.14976705210776,9.60760802538281,11.1650014857763));
#50326=CARTESIAN_POINT('Ctrl Pts',(-10.1283059986405,10.8319785554116,11.008001358424));
#50327=CARTESIAN_POINT('Ctrl Pts',(-10.7501648077581,13.992020329963,10.8510012310718));
#50328=CARTESIAN_POINT('Ctrl Pts',(-8.45749448845756,16.2537747113328,10.6940011037195));
#50329=CARTESIAN_POINT('Ctrl Pts',(-5.30626809181812,15.5892678153629,10.5370009763673));
#50330=CARTESIAN_POINT('Ctrl Pts',(-4.12216250860425,12.5942860586688,10.380000849015));
#50331=CARTESIAN_POINT('Ctrl Pts',(-5.96700624445078,9.95450088514863,10.2230007216628));
#50332=CARTESIAN_POINT('Ctrl Pts',(-9.18649505892511,10.0370112274744,10.0660005943105));
#50333=CARTESIAN_POINT('Ctrl Pts',(-10.8936901958899,12.7678403902015,9.90900046695827));
#50334=CARTESIAN_POINT('Ctrl Pts',(-9.5577294368621,15.6982219813021,9.752000339606));
#50335=CARTESIAN_POINT('Ctrl Pts',(-6.3765836355766,16.2004576199972,9.59500021225376));
#50336=CARTESIAN_POINT('Ctrl Pts',(-4.20281571587151,13.8241863062249,9.4380000849015));
#50337=CARTESIAN_POINT('Ctrl Pts',(-4.98566475436435,10.7002340827391,9.28099995754925));
#50338=CARTESIAN_POINT('Ctrl Pts',(-8.02314223764118,9.62987849036962,9.123999830197));
#50339=CARTESIAN_POINT('Ctrl Pts',(-10.5915131043488,11.5729178555327,8.96699970284474));
#50340=CARTESIAN_POINT('Ctrl Pts',(-10.3876944878733,14.7870100374982,8.80999957549249));
#50341=CARTESIAN_POINT('Ctrl Pts',(-7.59445253304005,16.3900477938888,8.65299944814024));
#50342=CARTESIAN_POINT('Ctrl Pts',(-4.71651407945554,14.9445717631999,8.49599932078798));
#50343=CARTESIAN_POINT('Ctrl Pts',(-4.33455415756585,11.7467541830206,8.33899919343573));
#50344=CARTESIAN_POINT('Ctrl Pts',(-6.79107988887037,9.66410874890807,8.18199906608347));
#50345=CARTESIAN_POINT('Ctrl Pts',(-9.88330108572798,10.5641636054531,8.02499893873122));
#50346=CARTESIAN_POINT('Ctrl Pts',(-10.8383933342348,13.6398309256761,7.86799881137897));
#50347=CARTESIAN_POINT('Ctrl Pts',(-8.79991625305057,16.1331303189645,7.71099868402671));
#50348=CARTESIAN_POINT('Ctrl Pts',(-5.59579179682231,15.8082962970528,7.55399855667447));
#50349=CARTESIAN_POINT('Ctrl Pts',(-4.09918910456809,12.956610648253,7.39699842932221));
#50350=CARTESIAN_POINT('Ctrl Pts',(-5.65212616815729,10.1352072431286,7.23999830196996));
#50351=CARTESIAN_POINT('Ctrl Pts',(-8.86206942440258,9.8740655989212,7.0829981746177));
#50352=CARTESIAN_POINT('Ctrl Pts',(-10.8506319608149,12.4073539009847,6.92599804726545));
#50353=CARTESIAN_POINT('Ctrl Pts',(-9.83465067318943,15.4634482887157,6.76899791991319));
#50354=CARTESIAN_POINT('Ctrl Pts',(-6.72516572981961,16.3019194823095,6.61199779256095));
#50355=CARTESIAN_POINT('Ctrl Pts',(-4.3104821089062,14.1709025601374,6.45499766520868));
#50356=CARTESIAN_POINT('Ctrl Pts',(-4.75586978181755,10.9813003676665,6.29799753785644));
#50357=CARTESIAN_POINT('Ctrl Pts',(-7.6619453433902,9.59326071540802,6.14099741050417));
#50358=CARTESIAN_POINT('Ctrl Pts',(-10.4228029696916,11.2514502662184,5.98399728315193));
#50359=CARTESIAN_POINT('Ctrl Pts',(-10.5627551177461,14.4689580825154,5.82699715579967));
#50360=CARTESIAN_POINT('Ctrl Pts',(-7.95630539875948,16.360607110615,5.66999702844743));
#50361=CARTESIAN_POINT('Ctrl Pts',(-4.94068219283476,15.23015107347,5.51299690109516));
#50362=CARTESIAN_POINT('Ctrl Pts',(-4.22002393159755,12.0912542249516,5.35599677374292));
#50363=CARTESIAN_POINT('Ctrl Pts',(-6.44055145447491,9.75864737041887,5.19899664639066));
#50364=CARTESIAN_POINT('Ctrl Pts',(-9.61109708849724,10.3238999309873,5.04199651903841));
#50365=CARTESIAN_POINT('Ctrl Pts',(-10.8886008563611,13.2803431519,4.88499639168615));
#50366=CARTESIAN_POINT('Ctrl Pts',(-9.12751539773043,15.9765173781352,4.72799626433391));
#50367=CARTESIAN_POINT('Ctrl Pts',(-5.9070180076098,15.995497775453,4.57099613698164));
#50368=CARTESIAN_POINT('Ctrl Pts',(-4.11496915512444,13.3187762924015,4.4139960096294));
#50369=CARTESIAN_POINT('Ctrl Pts',(-5.35829843455949,10.3495090655549,4.25699588227714));
#50370=CARTESIAN_POINT('Ctrl Pts',(-8.52212560854514,9.74453619934955,4.09999575492489));
#50371=CARTESIAN_POINT('Ctrl Pts',(-10.7694725263739,12.0578582844684,3.94299562757263));
#50372=CARTESIAN_POINT('Ctrl Pts',(-10.31234789899,14.1454191303684,3.83832887600446));
#50373=CARTESIAN_POINT('Ctrl Pts',(-9.6951971040191,14.8672444958454,3.78599550022038));
#50374=CARTESIAN_POINT('Ctrl Pts',(-8.19806642616107,10.379248870828,12.2140044997796));
#50375=CARTESIAN_POINT('Ctrl Pts',(-9.05665968914092,10.6087872809636,12.1616711239955));
#50376=CARTESIAN_POINT('Ctrl Pts',(-10.5158045072117,11.9764361665263,12.0570043724274));
#50377=CARTESIAN_POINT('Ctrl Pts',(-10.0088828130085,14.9518179872963,11.9000042450751));
#50378=CARTESIAN_POINT('Ctrl Pts',(-7.24818597120775,16.1623738615197,11.7430041177229));
#50379=CARTESIAN_POINT('Ctrl Pts',(-4.71531846299006,14.531497491576,11.5860039903706));
#50380=CARTESIAN_POINT('Ctrl Pts',(-4.67846996494438,11.5172053245294,11.4290038630183));
#50381=CARTESIAN_POINT('Ctrl Pts',(-7.17224146136718,9.82468019405374,11.2720037356661));
#50382=CARTESIAN_POINT('Ctrl Pts',(-9.9596478954327,10.9704830035337,11.1150036083138));
#50383=CARTESIAN_POINT('Ctrl Pts',(-10.5416020940281,13.9277452493586,10.9580034809616));
#50384=CARTESIAN_POINT('Ctrl Pts',(-8.39605217377323,16.0443631039765,10.8010033536093));
#50385=CARTESIAN_POINT('Ctrl Pts',(-5.44703962404145,15.4224975415121,10.6440032262571));
#50386=CARTESIAN_POINT('Ctrl Pts',(-4.33891796422385,12.6197034305821,10.4870030989048));
#50387=CARTESIAN_POINT('Ctrl Pts',(-6.06537828300873,10.1493129776432,10.3300029715526));
#50388=CARTESIAN_POINT('Ctrl Pts',(-9.07827285882558,10.2265286404914,10.1730028442003));
#50389=CARTESIAN_POINT('Ctrl Pts',(-10.6759174739885,12.7821207999897,10.0160027168481));
#50390=CARTESIAN_POINT('Ctrl Pts',(-9.4256851680762,15.5244601307577,9.85900258949583));
#50391=CARTESIAN_POINT('Ctrl Pts',(-6.4486731385623,15.9944673644538,9.70200246214356));
#50392=CARTESIAN_POINT('Ctrl Pts',(-4.41439566416342,13.7706811162314,9.54500233479132));
#50393=CARTESIAN_POINT('Ctrl Pts',(-5.14700936704523,10.8471925589996,9.38800220743905));
#50394=CARTESIAN_POINT('Ctrl Pts',(-7.98957225851618,9.84552156578271,9.23100208008681));
#50395=CARTESIAN_POINT('Ctrl Pts',(-10.393131052757,11.6638763112873,9.07400195273455));
#50396=CARTESIAN_POINT('Ctrl Pts',(-10.2023914542005,14.6717205559024,8.9170018253823));
#50397=CARTESIAN_POINT('Ctrl Pts',(-7.58839152451442,16.1718915580022,8.76000169803004));
#50398=CARTESIAN_POINT('Ctrl Pts',(-4.89513006096893,14.8191715632141,8.6030015706778));
#50399=CARTESIAN_POINT('Ctrl Pts',(-4.53768046472649,11.8265575810012,8.44600144332554));
#50400=CARTESIAN_POINT('Ctrl Pts',(-6.83657121344629,9.87755527244308,8.28900131597329));
#50401=CARTESIAN_POINT('Ctrl Pts',(-9.73036492049458,10.7198537090864,8.13200118862103));
#50402=CARTESIAN_POINT('Ctrl Pts',(-10.6241690057872,13.59815579992,7.97500106126879));
#50403=CARTESIAN_POINT('Ctrl Pts',(-8.71650077186918,15.9314604488298,7.81800093391652));
#50404=CARTESIAN_POINT('Ctrl Pts',(-5.71798462514094,15.6274709899262,7.66100080656428));
#50405=CARTESIAN_POINT('Ctrl Pts',(-4.31741876096606,12.9587776916062,7.50400067921201));
#50406=CARTESIAN_POINT('Ctrl Pts',(-5.77070402614152,10.3184234287576,7.34700055185978));
#50407=CARTESIAN_POINT('Ctrl Pts',(-8.7746655811378,10.0740392147746,7.19000042450751));
#50408=CARTESIAN_POINT('Ctrl Pts',(-10.6356222810626,12.4447666886372,7.03300029715527));
#50409=CARTESIAN_POINT('Ctrl Pts',(-9.68483639951025,15.304751839877,6.876000169803));
#50410=CARTESIAN_POINT('Ctrl Pts',(-6.77488675864068,16.0894184303616,6.71900004245076));
#50411=CARTESIAN_POINT('Ctrl Pts',(-4.51515311674835,14.0951486267455,6.56199991509849));
#50412=CARTESIAN_POINT('Ctrl Pts',(-4.93196031229355,11.1102228517267,6.40499978774625));
#50413=CARTESIAN_POINT('Ctrl Pts',(-7.65155332874137,9.81125354936211,6.24799966039399));
#50414=CARTESIAN_POINT('Ctrl Pts',(-10.2352470286507,11.3630372613762,6.09099953304174));
#50415=CARTESIAN_POINT('Ctrl Pts',(-10.3662184629517,14.3740779594481,5.93399940568949));
#50416=CARTESIAN_POINT('Ctrl Pts',(-7.92702433214164,16.1443400800951,5.77699927833723));
#50417=CARTESIAN_POINT('Ctrl Pts',(-5.10491333147909,15.0864252809503,5.61999915098498));
#50418=CARTESIAN_POINT('Ctrl Pts',(-4.4304996306029,12.1489510936098,5.46299902363272));
#50419=CARTESIAN_POINT('Ctrl Pts',(-6.50853614964623,9.96602736114071,5.30599889628047));
#50420=CARTESIAN_POINT('Ctrl Pts',(-9.47562822344969,10.4950077278519,5.14899876892822));
#50421=CARTESIAN_POINT('Ctrl Pts',(-10.6711547168104,13.2617363165495,4.99199864157597));
#50422=CARTESIAN_POINT('Ctrl Pts',(-9.02307791592096,15.7848973429709,4.83499851422371));
#50423=CARTESIAN_POINT('Ctrl Pts',(-6.0092394846447,15.8026597703067,4.67799838687145));
#50424=CARTESIAN_POINT('Ctrl Pts',(-4.33218620743569,13.2977032067055,4.52099825951921));
#50425=CARTESIAN_POINT('Ctrl Pts',(-5.49573118548395,10.5189735271065,4.36399813216694));
#50426=CARTESIAN_POINT('Ctrl Pts',(-8.45653592208301,9.95282170234728,4.20699800481471));
#50427=CARTESIAN_POINT('Ctrl Pts',(-10.5596708384907,12.117698166908,4.04999787746244));
#50428=CARTESIAN_POINT('Ctrl Pts',(-10.1318798475343,14.0713004658266,3.94533112589427));
#50429=CARTESIAN_POINT('Ctrl Pts',(-9.55433155034207,14.7468063779934,3.89299775011019));
#50430=CARTESIAN_POINT('Ctrl Pts',(-8.15019999797515,10.5582942547315,12.3210067496694));
#50431=CARTESIAN_POINT('Ctrl Pts',(-8.94991950449982,10.7720932116964,12.2686733738853));
#50432=CARTESIAN_POINT('Ctrl Pts',(-10.3090107345028,12.0459623870324,12.1640066223172));
#50433=CARTESIAN_POINT('Ctrl Pts',(-9.83684867056136,14.8173222194755,12.0070064949649));
#50434=CARTESIAN_POINT('Ctrl Pts',(-7.26545286397565,15.9448702542628,11.8500063676127));
#50435=CARTESIAN_POINT('Ctrl Pts',(-4.90626412921408,14.4258231081815,11.6930062402604));
#50436=CARTESIAN_POINT('Ctrl Pts',(-4.87194233338379,11.6182210126498,11.5360061129081));
#50437=CARTESIAN_POINT('Ctrl Pts',(-7.19471587062657,10.0417523627247,11.3790059855559));
#50438=CARTESIAN_POINT('Ctrl Pts',(-9.79098979222489,11.1089874516557,11.2220058582036));
#50439=CARTESIAN_POINT('Ctrl Pts',(-10.3330393802981,13.8634701687541,11.0650057308514));
#50440=CARTESIAN_POINT('Ctrl Pts',(-8.33460985908889,15.8349514966202,10.9080056034991));
#50441=CARTESIAN_POINT('Ctrl Pts',(-5.5878111562648,15.2557272676614,10.7510054761469));
#50442=CARTESIAN_POINT('Ctrl Pts',(-4.55567341984345,12.6451208024954,10.5940053487946));
#50443=CARTESIAN_POINT('Ctrl Pts',(-6.16375032156668,10.3441250701379,10.4370052214424));
#50444=CARTESIAN_POINT('Ctrl Pts',(-8.97005065872605,10.4160460535085,10.2800050940901));
#50445=CARTESIAN_POINT('Ctrl Pts',(-10.4581447520871,12.796401209778,10.1230049667379));
#50446=CARTESIAN_POINT('Ctrl Pts',(-9.29364089929031,15.3506982802133,9.96600483938563));
#50447=CARTESIAN_POINT('Ctrl Pts',(-6.52076264154797,15.7884771089103,9.80900471203338));
#50448=CARTESIAN_POINT('Ctrl Pts',(-4.62597561245536,13.7171759262378,9.65200458468112));
#50449=CARTESIAN_POINT('Ctrl Pts',(-5.3083539797261,10.9941510352601,9.49500445732887));
#50450=CARTESIAN_POINT('Ctrl Pts',(-7.95600227939119,10.0611646411958,9.33800432997662));
#50451=CARTESIAN_POINT('Ctrl Pts',(-10.1947490011651,11.7548347670419,9.18100420262436));
#50452=CARTESIAN_POINT('Ctrl Pts',(-10.0170884205278,14.5564310743066,9.02400407527211));
#50453=CARTESIAN_POINT('Ctrl Pts',(-7.5823305159888,15.9537353221155,8.86700394791986));
#50454=CARTESIAN_POINT('Ctrl Pts',(-5.07374604248231,14.6937713632283,8.71000382056761));
#50455=CARTESIAN_POINT('Ctrl Pts',(-4.74080677188713,11.9063609789818,8.55300369321535));
#50456=CARTESIAN_POINT('Ctrl Pts',(-6.88206253802222,10.0910017959781,8.3960035658631));
#50457=CARTESIAN_POINT('Ctrl Pts',(-9.57742875526118,10.8755438127196,8.23900343851084));
#50458=CARTESIAN_POINT('Ctrl Pts',(-10.4099446773395,13.5564806741639,8.0820033111586));
#50459=CARTESIAN_POINT('Ctrl Pts',(-8.63308529068779,15.7297905786951,7.92500318380633));
#50460=CARTESIAN_POINT('Ctrl Pts',(-5.84017745345957,15.4466456827995,7.7680030564541));
#50461=CARTESIAN_POINT('Ctrl Pts',(-4.53564841736402,12.9609447349594,7.61100292910181));
#50462=CARTESIAN_POINT('Ctrl Pts',(-5.88928188412577,10.5016396143867,7.45400280174959));
#50463=CARTESIAN_POINT('Ctrl Pts',(-8.687261737873,10.2740128306281,7.29700267439731));
#50464=CARTESIAN_POINT('Ctrl Pts',(-10.4206126013104,12.4821794762896,7.14000254704508));
#50465=CARTESIAN_POINT('Ctrl Pts',(-9.53502212583107,15.1460553910382,6.98300241969281));
#50466=CARTESIAN_POINT('Ctrl Pts',(-6.82460778746177,15.8769173784138,6.82600229234057));
#50467=CARTESIAN_POINT('Ctrl Pts',(-4.71982412459047,14.0193946933536,6.66900216498831));
#50468=CARTESIAN_POINT('Ctrl Pts',(-5.10805084276957,11.2391453357869,6.51200203763605));
#50469=CARTESIAN_POINT('Ctrl Pts',(-7.64116131409251,10.0292463833162,6.35500191028381));
#50470=CARTESIAN_POINT('Ctrl Pts',(-10.0476910876099,11.474624256534,6.19800178293155));
#50471=CARTESIAN_POINT('Ctrl Pts',(-10.1696818081572,14.2791978363808,6.0410016555793));
#50472=CARTESIAN_POINT('Ctrl Pts',(-7.89774326552381,15.9280730495752,5.88400152822705));
#50473=CARTESIAN_POINT('Ctrl Pts',(-5.26914447012342,14.9426994884306,5.72700140087479));
#50474=CARTESIAN_POINT('Ctrl Pts',(-4.64097532960824,12.206647962268,5.57000127352254));
#50475=CARTESIAN_POINT('Ctrl Pts',(-6.57652084481755,10.1734073518625,5.41300114617028));
#50476=CARTESIAN_POINT('Ctrl Pts',(-9.34015935840215,10.6661155247165,5.25600101881803));
#50477=CARTESIAN_POINT('Ctrl Pts',(-10.4537085772597,13.243129481199,5.09900089146578));
#50478=CARTESIAN_POINT('Ctrl Pts',(-8.91864043411149,15.5932773078066,4.94200076411352));
#50479=CARTESIAN_POINT('Ctrl Pts',(-6.11146096167962,15.6098217651605,4.78500063676127));
#50480=CARTESIAN_POINT('Ctrl Pts',(-4.54940325974693,13.2766301210095,4.62800050940902));
#50481=CARTESIAN_POINT('Ctrl Pts',(-5.63316393640839,10.6884379886581,4.47100038205676));
#50482=CARTESIAN_POINT('Ctrl Pts',(-8.39094623562089,10.161107205345,4.31400025470451));
#50483=CARTESIAN_POINT('Ctrl Pts',(-10.3498691506075,12.1775380493476,4.15700012735225));
#50484=CARTESIAN_POINT('Ctrl Pts',(-9.95141179607851,13.9971818012848,4.05233337578409));
#50485=CARTESIAN_POINT('Ctrl Pts',(-9.41346599666504,14.6263682601415,4.));
#50486=CARTESIAN_POINT('Ctrl Pts',(-10.0159019782719,12.9923925656114,11.112583302492));
#50487=CARTESIAN_POINT('Ctrl Pts',(-10.017856950592,13.2435976299952,11.0967241119451));
#50488=CARTESIAN_POINT('Ctrl Pts',(-9.98318348246503,13.4942759769916,11.0808649213983));
#50489=CARTESIAN_POINT('Ctrl Pts',(-9.90962619541772,13.7329699372154,11.0650057308514));
#50490=CARTESIAN_POINT('Ctrl Pts',(-9.66689620656173,14.5206306113761,11.0126723550673));
#50491=CARTESIAN_POINT('Ctrl Pts',(-9.00075303282531,15.1777910539982,10.9603389792832));
#50492=CARTESIAN_POINT('Ctrl Pts',(-8.20988166215309,15.409833903816,10.9080056034991));
#50493=CARTESIAN_POINT('Ctrl Pts',(-7.41901029148087,15.6418767536339,10.8556722277151));
#50494=CARTESIAN_POINT('Ctrl Pts',(-6.50341072387283,15.4488020106477,10.803338851931));
#50495=CARTESIAN_POINT('Ctrl Pts',(-5.87358798399859,14.9171635616269,10.7510054761469));
#50496=CARTESIAN_POINT('Ctrl Pts',(-5.24376524412435,14.3855251126061,10.6986721003628));
#50497=CARTESIAN_POINT('Ctrl Pts',(-4.8997193319839,13.5153229575507,10.6463387245787));
#50498=CARTESIAN_POINT('Ctrl Pts',(-4.99570919286755,12.6967225912968,10.5940053487946));
#50499=CARTESIAN_POINT('Ctrl Pts',(-5.09169905375119,11.8781222250429,10.5416719730106));
#50500=CARTESIAN_POINT('Ctrl Pts',(-5.62772468765894,11.1111236475904,10.4893385972265));
#50501=CARTESIAN_POINT('Ctrl Pts',(-6.3634542274727,10.7396111894259,10.4370052214424));
#50502=CARTESIAN_POINT('Ctrl Pts',(-7.09918376728647,10.3680987312614,10.3846718456583));
#50503=CARTESIAN_POINT('Ctrl Pts',(-8.03461721300627,10.392072392385,10.3323384698742));
#50504=CARTESIAN_POINT('Ctrl Pts',(-8.750349618093,10.800785082325,10.2800050940901));
#50505=CARTESIAN_POINT('Ctrl Pts',(-9.46608202317973,11.209497772265,10.227671718306));
#50506=CARTESIAN_POINT('Ctrl Pts',(-9.9621133876334,12.0029494910215,10.175338342522));
#50507=CARTESIAN_POINT('Ctrl Pts',(-10.0160450943941,12.8253915288056,10.1230049667379));
#50508=CARTESIAN_POINT('Ctrl Pts',(-10.0196250796435,12.8799852092316,10.1195310786559));
#50509=CARTESIAN_POINT('Ctrl Pts',(-10.0212570407989,12.9347066297247,10.116057190574));
#50510=CARTESIAN_POINT('Ctrl Pts',(-10.0209918820407,12.9894441341194,10.112583302492));
#50511=CARTESIAN_POINT('Ctrl Pts',(-8.29379928253292,10.0211581030209,12.));
#50512=CARTESIAN_POINT('Ctrl Pts',(-8.38688154479599,10.0552080103525,12.));
#50513=CARTESIAN_POINT('Ctrl Pts',(-8.4779006806254,10.0940206699959,12.));
#50514=CARTESIAN_POINT('Ctrl Pts',(-8.56664686325615,10.1372696205127,12.));
#50515=CARTESIAN_POINT('Ctrl Pts',(-8.65733903335545,10.1814669150961,12.));
#50516=CARTESIAN_POINT('Ctrl Pts',(-8.74565814612796,10.2302978026812,12.));
#50517=CARTESIAN_POINT('Ctrl Pts',(-8.83135135493958,10.2834593640583,12.));
#50518=CARTESIAN_POINT('Ctrl Pts',(-8.91318992856164,10.3342296224599,12.));
#50519=CARTESIAN_POINT('Ctrl Pts',(-8.99263375816446,10.3889506025256,12.));
#50520=CARTESIAN_POINT('Ctrl Pts',(-9.06943047246088,10.4473877517771,12.));
#50521=CARTESIAN_POINT('Ctrl Pts',(-9.13662759747024,10.4985202573722,12.));
#50522=CARTESIAN_POINT('Ctrl Pts',(-9.20179774209257,10.5524986289602,12.));
#50523=CARTESIAN_POINT('Ctrl Pts',(-9.26474793392036,10.6091781306825,12.));
#50524=CARTESIAN_POINT('Ctrl Pts',(-9.27985634938565,10.6227815437226,12.));
#50525=CARTESIAN_POINT('Ctrl Pts',(-9.29484046111391,10.636544177759,12.));
#50526=CARTESIAN_POINT('Ctrl Pts',(-9.30967515586603,10.6504428556362,12.));
#50527=CARTESIAN_POINT('Ctrl Pts',(-9.38210515214773,10.718302774818,12.));
#50528=CARTESIAN_POINT('Ctrl Pts',(-9.45106930229927,10.7894833711807,12.));
#50529=CARTESIAN_POINT('Ctrl Pts',(-9.51632661790574,10.8636962448604,12.));
#50530=CARTESIAN_POINT('Ctrl Pts',(-9.58121902341258,10.9374941301685,12.));
#50531=CARTESIAN_POINT('Ctrl Pts',(-9.64244642197802,11.0142912680357,12.));
#50532=CARTESIAN_POINT('Ctrl Pts',(-9.69972824598415,11.0938308479656,12.));
#50533=CARTESIAN_POINT('Ctrl Pts',(-9.75408303717497,11.169306050327,12.));
#50534=CARTESIAN_POINT('Ctrl Pts',(-9.80488522775839,11.2472513152745,12.));
#50535=CARTESIAN_POINT('Ctrl Pts',(-9.85185250012922,11.3274602381139,12.));
#50536=CARTESIAN_POINT('Ctrl Pts',(-9.88922975528545,11.3912916940074,12.));
#50537=CARTESIAN_POINT('Ctrl Pts',(-9.92417754353756,11.4565571180282,12.));
#50538=CARTESIAN_POINT('Ctrl Pts',(-9.95653223361561,11.5231545729247,12.));
#50539=CARTESIAN_POINT('Ctrl Pts',(-9.96243512991986,11.5353048321122,12.));
#50540=CARTESIAN_POINT('Ctrl Pts',(-9.96824994557655,11.5474959894548,12.));
#50541=CARTESIAN_POINT('Ctrl Pts',(-9.97397248881904,11.5597200854486,12.));
#50542=CARTESIAN_POINT('Ctrl Pts',(-10.0145489524258,11.6463966845059,12.));
#50543=CARTESIAN_POINT('Ctrl Pts',(-10.0505436256048,11.7348369448931,12.));
#50544=CARTESIAN_POINT('Ctrl Pts',(-10.0816929753162,11.8247972357439,12.));
#50545=CARTESIAN_POINT('Ctrl Pts',(-10.1128423250276,11.9147575265948,12.));
#50546=CARTESIAN_POINT('Ctrl Pts',(-10.1391468173479,12.0062385811789,12.));
#50547=CARTESIAN_POINT('Ctrl Pts',(-10.1602867132728,12.0990065815937,12.));
#50548=CARTESIAN_POINT('Ctrl Pts',(-10.1814517508012,12.1918849106638,12.));
#50549=CARTESIAN_POINT('Ctrl Pts',(-10.197439126489,12.286054432468,12.));
#50550=CARTESIAN_POINT('Ctrl Pts',(-10.2083242813819,12.381106938598,12.));
#50551=CARTESIAN_POINT('Ctrl Pts',(-10.2138913557349,12.4297203367777,12.));
#50552=CARTESIAN_POINT('Ctrl Pts',(-10.2181230259612,12.4785645227018,12.));
#50553=CARTESIAN_POINT('Ctrl Pts',(-10.2210244442513,12.527583085919,12.));
#50554=CARTESIAN_POINT('Ctrl Pts',(-10.2218610165225,12.5417167152898,12.));
#50555=CARTESIAN_POINT('Ctrl Pts',(-10.2225869774383,12.5558648310221,12.));
#50556=CARTESIAN_POINT('Ctrl Pts',(-10.2232024018895,12.5700260533185,12.));
#50557=CARTESIAN_POINT('Ctrl Pts',(-10.2238236012139,12.5843201583174,12.));
#50558=CARTESIAN_POINT('Ctrl Pts',(-10.2243317772527,12.598618709654,12.));
#50559=CARTESIAN_POINT('Ctrl Pts',(-10.2247273702154,12.6129172463203,12.));
#50560=CARTESIAN_POINT('Ctrl Pts',(-10.227308430526,12.7062085557579,12.));
#50561=CARTESIAN_POINT('Ctrl Pts',(-10.2251031453087,12.7995425030326,12.));
#50562=CARTESIAN_POINT('Ctrl Pts',(-10.2182400386914,12.8925419864032,12.));
#50563=CARTESIAN_POINT('Ctrl Pts',(-10.2113727169558,12.985598587323,12.));
#50564=CARTESIAN_POINT('Ctrl Pts',(-10.1998414736524,13.0783212906945,12.));
#50565=CARTESIAN_POINT('Ctrl Pts',(-10.1837245157332,13.1703195860503,12.));
#50566=CARTESIAN_POINT('Ctrl Pts',(-10.167850633777,13.2609303630954,12.));
#50567=CARTESIAN_POINT('Ctrl Pts',(-10.1475278620093,13.3508392541549,12.));
#50568=CARTESIAN_POINT('Ctrl Pts',(-10.1227882581427,13.4396474637383,12.));
#50569=CARTESIAN_POINT('Ctrl Pts',(-10.1129089853156,13.4751112705354,12.));
#50570=CARTESIAN_POINT('Ctrl Pts',(-10.102324939091,13.5103991993701,12.));
#50571=CARTESIAN_POINT('Ctrl Pts',(-10.0910364592447,13.5454842372103,12.));
#50572=CARTESIAN_POINT('Ctrl Pts',(-10.0850885997417,13.5639704176856,12.));
#50573=CARTESIAN_POINT('Ctrl Pts',(-10.0789451599571,13.5824002543575,12.));
#50574=CARTESIAN_POINT('Ctrl Pts',(-10.0726060885077,13.6007696733809,12.));
#50575=CARTESIAN_POINT('Ctrl Pts',(-10.0672512100823,13.6162870888888,12.));
#50576=CARTESIAN_POINT('Ctrl Pts',(-10.0617593012071,13.6317538427315,12.));
#50577=CARTESIAN_POINT('Ctrl Pts',(-10.05613256518,13.6471627242414,12.));
#50578=CARTESIAN_POINT('Ctrl Pts',(-10.0253173594462,13.7315505205696,12.));
#50579=CARTESIAN_POINT('Ctrl Pts',(-9.99044489732798,13.8142532308756,12.));
#50580=CARTESIAN_POINT('Ctrl Pts',(-9.95156720789968,13.8949006686344,12.));
#50581=CARTESIAN_POINT('Ctrl Pts',(-9.92246136322671,13.9552775025255,12.));
#50582=CARTESIAN_POINT('Ctrl Pts',(-9.89110978386257,14.0145019588769,12.));
#50583=CARTESIAN_POINT('Ctrl Pts',(-9.85752072526523,14.0724054243587,12.));
#50584=CARTESIAN_POINT('Ctrl Pts',(-9.84460176992236,14.0946761373823,12.));
#50585=CARTESIAN_POINT('Ctrl Pts',(-9.83135170762611,14.1167512973966,12.));
#50586=CARTESIAN_POINT('Ctrl Pts',(-9.81777059343282,14.1386207605303,12.));
#50587=CARTESIAN_POINT('Ctrl Pts',(-9.80600921691784,14.1575599275555,12.));
#50588=CARTESIAN_POINT('Ctrl Pts',(-9.79399757751539,14.1763475835755,12.));
#50589=CARTESIAN_POINT('Ctrl Pts',(-9.78174994291027,14.194955852553,12.));
#50590=CARTESIAN_POINT('Ctrl Pts',(-9.73447804437696,14.2667777374594,12.));
#50591=CARTESIAN_POINT('Ctrl Pts',(-9.68365470418875,14.3359945738428,12.));
#50592=CARTESIAN_POINT('Ctrl Pts',(-9.62930889486242,14.4022524491644,12.));
#50593=CARTESIAN_POINT('Ctrl Pts',(-9.58717510546268,14.453621550103,12.));
#50594=CARTESIAN_POINT('Ctrl Pts',(-9.54292331405751,14.5032115233845,12.));
#50595=CARTESIAN_POINT('Ctrl Pts',(-9.49655459700825,14.5508396884611,12.));
#50596=CARTESIAN_POINT('Ctrl Pts',(-9.47068873424204,14.5774081091567,12.));
#50597=CARTESIAN_POINT('Ctrl Pts',(-9.44416391721335,14.6033657382126,12.));
#50598=CARTESIAN_POINT('Ctrl Pts',(-9.41700728965907,14.6287007311509,12.));
#50599=CARTESIAN_POINT('Origin',(-7.5,12.9903810567666,7.5));
#50600=CARTESIAN_POINT('Origin',(-7.50000000000001,-12.9903810567666,4.));
#50601=CARTESIAN_POINT('Ctrl Pts',(-9.41346599666503,-11.3543938533916,
4.));
#50602=CARTESIAN_POINT('Ctrl Pts',(-9.47563125999352,-11.4128139360928,
4.));
#50603=CARTESIAN_POINT('Ctrl Pts',(-9.5344254182292,-11.4744857433087,4.));
#50604=CARTESIAN_POINT('Ctrl Pts',(-9.58983450470078,-11.5390333604437,
4.));
#50605=CARTESIAN_POINT('Ctrl Pts',(-9.64659408185619,-11.6051542024983,
4.));
#50606=CARTESIAN_POINT('Ctrl Pts',(-9.69980203857783,-11.6742932390243,
4.));
#50607=CARTESIAN_POINT('Ctrl Pts',(-9.74941453503823,-11.7460926626337,
4.));
#50608=CARTESIAN_POINT('Ctrl Pts',(-9.76241984954432,-11.7649140111248,
4.));
#50609=CARTESIAN_POINT('Ctrl Pts',(-9.77517792533989,-11.7839183899685,
4.));
#50610=CARTESIAN_POINT('Ctrl Pts',(-9.78768759195629,-11.8030997933617,
4.));
#50611=CARTESIAN_POINT('Ctrl Pts',(-9.79776752365911,-11.8185556198114,
4.));
#50612=CARTESIAN_POINT('Ctrl Pts',(-9.8076865335191,-11.8341271625133,4.));
#50613=CARTESIAN_POINT('Ctrl Pts',(-9.81743537915168,-11.8497970439193,
4.));
#50614=CARTESIAN_POINT('Ctrl Pts',(-9.86491247379083,-11.9261097142127,
4.));
#50615=CARTESIAN_POINT('Ctrl Pts',(-9.90840731623012,-12.0048277686438,
4.));
#50616=CARTESIAN_POINT('Ctrl Pts',(-9.94788306281372,-12.0855595944701,
4.));
#50617=CARTESIAN_POINT('Ctrl Pts',(-9.97942487229752,-12.150065730259,4.));
#50618=CARTESIAN_POINT('Ctrl Pts',(-10.0084002601673,-12.2158586031585,
4.));
#50619=CARTESIAN_POINT('Ctrl Pts',(-10.034773868227,-12.2827556582142,4.));
#50620=CARTESIAN_POINT('Ctrl Pts',(-10.0434527794708,-12.3047698476261,
4.));
#50621=CARTESIAN_POINT('Ctrl Pts',(-10.0518498142904,-12.326903713834,4.));
#50622=CARTESIAN_POINT('Ctrl Pts',(-10.0599633247681,-12.3491510331904,
4.));
#50623=CARTESIAN_POINT('Ctrl Pts',(-10.0673313519173,-12.369354230495,4.));
#50624=CARTESIAN_POINT('Ctrl Pts',(-10.0744669979504,-12.3896556179549,
4.));
#50625=CARTESIAN_POINT('Ctrl Pts',(-10.0813595780794,-12.4100219884372,
4.));
#50626=CARTESIAN_POINT('Ctrl Pts',(-10.110937259752,-12.4974188719965,4.));
#50627=CARTESIAN_POINT('Ctrl Pts',(-10.1360761396945,-12.5860974112731,
4.));
#50628=CARTESIAN_POINT('Ctrl Pts',(-10.1567415216565,-12.6756607739627,
4.));
#50629=CARTESIAN_POINT('Ctrl Pts',(-10.1777235800004,-12.7665966059193,
4.));
#50630=CARTESIAN_POINT('Ctrl Pts',(-10.194094489083,-12.8584453915162,4.));
#50631=CARTESIAN_POINT('Ctrl Pts',(-10.205776157801,-12.9508249271276,4.));
#50632=CARTESIAN_POINT('Ctrl Pts',(-10.2173669041142,-13.0424854413619,
4.));
#50633=CARTESIAN_POINT('Ctrl Pts',(-10.2243414700862,-13.1346694027891,
4.00000000000001));
#50634=CARTESIAN_POINT('Ctrl Pts',(-10.2265766240073,-13.2270226781325,
4.00000000000001));
#50635=CARTESIAN_POINT('Ctrl Pts',(-10.2276561070688,-13.2716253318781,
4.00000000000001));
#50636=CARTESIAN_POINT('Ctrl Pts',(-10.2276293996605,-13.3162676791034,
4.00000000000001));
#50637=CARTESIAN_POINT('Ctrl Pts',(-10.2264782755414,-13.360910468216,4.00000000000001));
#50638=CARTESIAN_POINT('Ctrl Pts',(-10.2261080116976,-13.3752700063553,
4.00000000000001));
#50639=CARTESIAN_POINT('Ctrl Pts',(-10.2256213911499,-13.3896295910271,
4.00000000000001));
#50640=CARTESIAN_POINT('Ctrl Pts',(-10.2250177409671,-13.40398791621,4.00000000000001));
#50641=CARTESIAN_POINT('Ctrl Pts',(-10.2243866916487,-13.4189979527825,
4.00000000000001));
#50642=CARTESIAN_POINT('Ctrl Pts',(-10.2236280724728,-13.4339981404011,
4.));
#50643=CARTESIAN_POINT('Ctrl Pts',(-10.2227419311859,-13.4489814918393,
4.));
#50644=CARTESIAN_POINT('Ctrl Pts',(-10.2170924746832,-13.5445055278686,
4.));
#50645=CARTESIAN_POINT('Ctrl Pts',(-10.2062608557766,-13.6394136430286,
4.));
#50646=CARTESIAN_POINT('Ctrl Pts',(-10.1901745261949,-13.7333115332678,
4.));
#50647=CARTESIAN_POINT('Ctrl Pts',(-10.1886860667379,-13.74199985474,4.));
#50648=CARTESIAN_POINT('Ctrl Pts',(-10.1871525835688,-13.7506795401449,
4.));
#50649=CARTESIAN_POINT('Ctrl Pts',(-10.1855739978038,-13.7593502843482,
4.));
#50650=CARTESIAN_POINT('Ctrl Pts',(-10.1691852106353,-13.8493694549782,
4.));
#50651=CARTESIAN_POINT('Ctrl Pts',(-10.1479394797701,-13.9384246529327,
4.));
#50652=CARTESIAN_POINT('Ctrl Pts',(-10.1221390901744,-14.0262810420052,
4.));
#50653=CARTESIAN_POINT('Ctrl Pts',(-10.0957476132678,-14.1161502222633,
4.));
#50654=CARTESIAN_POINT('Ctrl Pts',(-10.0645901923201,-14.2047657338476,
4.));
#50655=CARTESIAN_POINT('Ctrl Pts',(-10.0289360631668,-14.2918733204662,
4.));
#50656=CARTESIAN_POINT('Ctrl Pts',(-10.0090443370482,-14.3404713453517,
4.));
#50657=CARTESIAN_POINT('Ctrl Pts',(-9.98775201258348,-14.3885999003503,
4.));
#50658=CARTESIAN_POINT('Ctrl Pts',(-9.96509914777034,-14.4362131753606,
4.));
#50659=CARTESIAN_POINT('Ctrl Pts',(-9.95876399288502,-14.4495288188465,
4.));
#50660=CARTESIAN_POINT('Ctrl Pts',(-9.95232213153922,-14.4628045348086,
4.));
#50661=CARTESIAN_POINT('Ctrl Pts',(-9.94578145907892,-14.4760254702856,
4.));
#50662=CARTESIAN_POINT('Ctrl Pts',(-9.90302407067229,-14.562452772175,4.));
#50663=CARTESIAN_POINT('Ctrl Pts',(-9.85598091444247,-14.6466834011242,
4.));
#50664=CARTESIAN_POINT('Ctrl Pts',(-9.80499202080536,-14.7284640330205,
4.));
#50665=CARTESIAN_POINT('Ctrl Pts',(-9.75299794500559,-14.8118568676255,
4.));
#50666=CARTESIAN_POINT('Ctrl Pts',(-9.69690071688324,-14.8927029338428,
4.));
#50667=CARTESIAN_POINT('Ctrl Pts',(-9.63700597453379,-14.9707266774082,
4.));
#50668=CARTESIAN_POINT('Ctrl Pts',(-9.57663995749172,-15.049364341567,4.));
#50669=CARTESIAN_POINT('Ctrl Pts',(-9.51241597456512,-15.1251359367173,
4.));
#50670=CARTESIAN_POINT('Ctrl Pts',(-9.44459769690279,-15.1977400638646,
4.));
#50671=CARTESIAN_POINT('Ctrl Pts',(-9.40866340733751,-15.2362101904805,
4.));
#50672=CARTESIAN_POINT('Ctrl Pts',(-9.37171922385876,-15.2737906405076,
4.));
#50673=CARTESIAN_POINT('Ctrl Pts',(-9.33379951949355,-15.3104331478965,
4.));
#50674=CARTESIAN_POINT('Ctrl Pts',(-9.31851290781191,-15.3252048817713,
4.));
#50675=CARTESIAN_POINT('Ctrl Pts',(-9.30306772443973,-15.339824154646,4.));
#50676=CARTESIAN_POINT('Ctrl Pts',(-9.28746608368795,-15.3542876681649,
4.));
#50677=CARTESIAN_POINT('Ctrl Pts',(-9.27676581806402,-15.3642073579572,
4.));
#50678=CARTESIAN_POINT('Ctrl Pts',(-9.26599878272636,-15.3740474389504,
4.));
#50679=CARTESIAN_POINT('Ctrl Pts',(-9.25516737653956,-15.3838058321128,
4.));
#50680=CARTESIAN_POINT('Ctrl Pts',(-9.17938057199806,-15.452084818468,4.));
#50681=CARTESIAN_POINT('Ctrl Pts',(-9.10042438929677,-15.5163865482147,
4.));
#50682=CARTESIAN_POINT('Ctrl Pts',(-9.01862162231471,-15.5764248312756,
4.));
#50683=CARTESIAN_POINT('Ctrl Pts',(-8.93674927983158,-15.636514178546,4.));
#50684=CARTESIAN_POINT('Ctrl Pts',(-8.8520249381574,-15.6923336670045,4.));
#50685=CARTESIAN_POINT('Ctrl Pts',(-8.76472731465809,-15.7435701437727,
4.));
#50686=CARTESIAN_POINT('Ctrl Pts',(-8.67912044767158,-15.7938142864623,
4.));
#50687=CARTESIAN_POINT('Ctrl Pts',(-8.59103835537406,-15.8396519102272,
4.));
#50688=CARTESIAN_POINT('Ctrl Pts',(-8.50070999295064,-15.8807513482254,
4.));
#50689=CARTESIAN_POINT('Ctrl Pts',(-8.47449902628609,-15.8926773476613,
4.));
#50690=CARTESIAN_POINT('Ctrl Pts',(-8.44809873411205,-15.9042041128398,
4.));
#50691=CARTESIAN_POINT('Ctrl Pts',(-8.42151428132428,-15.9153228238725,
4.));
#50692=CARTESIAN_POINT('Ctrl Pts',(-8.38003054177093,-15.9326730291346,
4.));
#50693=CARTESIAN_POINT('Ctrl Pts',(-8.3380984052677,-15.9490297174903,4.));
#50694=CARTESIAN_POINT('Ctrl Pts',(-8.29574966236114,-15.9643994715412,
4.));
#50695=CARTESIAN_POINT('Ctrl Pts',(-6.7062007174672,-15.9596040105123,4.));
#50696=CARTESIAN_POINT('Ctrl Pts',(-6.61134542475377,-15.9249055207219,
4.));
#50697=CARTESIAN_POINT('Ctrl Pts',(-6.51853060534356,-15.8852234998271,
4.));
#50698=CARTESIAN_POINT('Ctrl Pts',(-6.42799851956089,-15.8408762347418,
4.));
#50699=CARTESIAN_POINT('Ctrl Pts',(-6.33621693362306,-15.7959169003098,
4.));
#50700=CARTESIAN_POINT('Ctrl Pts',(-6.24678085823289,-15.7461619565544,
4.));
#50701=CARTESIAN_POINT('Ctrl Pts',(-6.15997674190851,-15.691902411869,4.));
#50702=CARTESIAN_POINT('Ctrl Pts',(-6.13531568434349,-15.6764872701499,
4.));
#50703=CARTESIAN_POINT('Ctrl Pts',(-6.11086730231581,-15.6607083372246,
4.));
#50704=CARTESIAN_POINT('Ctrl Pts',(-6.08663877235659,-15.6445718215519,
4.));
#50705=CARTESIAN_POINT('Ctrl Pts',(-6.06744081682964,-15.6317857337964,
4.));
#50706=CARTESIAN_POINT('Ctrl Pts',(-6.0483789202221,-15.6187736030245,4.));
#50707=CARTESIAN_POINT('Ctrl Pts',(-6.02947561532874,-15.6055520498285,
4.));
#50708=CARTESIAN_POINT('Ctrl Pts',(-5.94677128184633,-15.5477060937462,
4.));
#50709=CARTESIAN_POINT('Ctrl Pts',(-5.86702045523495,-15.485803012119,4.));
#50710=CARTESIAN_POINT('Ctrl Pts',(-5.79049058680189,-15.4201377361794,
4.));
#50711=CARTESIAN_POINT('Ctrl Pts',(-5.73202513270763,-15.3699723529815,
4.));
#50712=CARTESIAN_POINT('Ctrl Pts',(-5.67544017028651,-15.3176103400047,
4.));
#50713=CARTESIAN_POINT('Ctrl Pts',(-5.62087197491949,-15.2631717733717,
4.));
#50714=CARTESIAN_POINT('Ctrl Pts',(-5.59237459351674,-15.2347420885356,
4.));
#50715=CARTESIAN_POINT('Ctrl Pts',(-5.56442750315923,-15.2057459282144,
4.));
#50716=CARTESIAN_POINT('Ctrl Pts',(-5.53705194133909,-15.1761996365986,
4.));
#50717=CARTESIAN_POINT('Ctrl Pts',(-5.52590419986363,-15.1641679412254,
4.));
#50718=CARTESIAN_POINT('Ctrl Pts',(-5.51485102559337,-15.1520446566585,
4.));
#50719=CARTESIAN_POINT('Ctrl Pts',(-5.50390395570898,-15.1398423958921,
4.));
#50720=CARTESIAN_POINT('Ctrl Pts',(-5.43813919199008,-15.0665370452716,
4.));
#50721=CARTESIAN_POINT('Ctrl Pts',(-5.37610812852687,-14.9902855415477,
4.));
#50722=CARTESIAN_POINT('Ctrl Pts',(-5.31805567958009,-14.9113640105217,
4.));
#50723=CARTESIAN_POINT('Ctrl Pts',(-5.26107088016972,-14.8338939348183,
4.));
#50724=CARTESIAN_POINT('Ctrl Pts',(-5.20791934818337,-14.7538503489036,
4.));
#50725=CARTESIAN_POINT('Ctrl Pts',(-5.15887699703074,-14.6714727381725,
4.));
#50726=CARTESIAN_POINT('Ctrl Pts',(-5.11076871641508,-14.5906641080731,
4.));
#50727=CARTESIAN_POINT('Ctrl Pts',(-5.0666142946296,-14.5076088453843,4.));
#50728=CARTESIAN_POINT('Ctrl Pts',(-5.02672179249125,-14.4225226052514,
4.));
#50729=CARTESIAN_POINT('Ctrl Pts',(-5.00642778712802,-14.3792377642152,
4.));
#50730=CARTESIAN_POINT('Ctrl Pts',(-4.98723753203067,-14.3354272137238,
4.));
#50731=CARTESIAN_POINT('Ctrl Pts',(-4.96919681035721,-14.2911191061582,
4.));
#50732=CARTESIAN_POINT('Ctrl Pts',(-4.96034382211253,-14.2693761203441,
4.));
#50733=CARTESIAN_POINT('Ctrl Pts',(-4.95176770738618,-14.2475133193776,
4.));
#50734=CARTESIAN_POINT('Ctrl Pts',(-4.94347420847157,-14.2255340469214,
4.));
#50735=CARTESIAN_POINT('Ctrl Pts',(-4.93874143956184,-14.2129913531307,
4.));
#50736=CARTESIAN_POINT('Ctrl Pts',(-4.93410201278753,-14.2004140677721,
4.));
#50737=CARTESIAN_POINT('Ctrl Pts',(-4.92955955708199,-14.1878106688628,
4.));
#50738=CARTESIAN_POINT('Ctrl Pts',(-4.89805327414987,-14.1003940207578,
4.));
#50739=CARTESIAN_POINT('Ctrl Pts',(-4.87116570943181,-14.0116107665047,
4.));
#50740=CARTESIAN_POINT('Ctrl Pts',(-4.8491500138814,-13.9216823090563,4.));
#50741=CARTESIAN_POINT('Ctrl Pts',(-4.84589778208928,-13.9083977781333,
4.));
#50742=CARTESIAN_POINT('Ctrl Pts',(-4.84275195632634,-13.8950882390595,
4.));
#50743=CARTESIAN_POINT('Ctrl Pts',(-4.8397134492654,-13.8817543903633,4.));
#50744=CARTESIAN_POINT('Ctrl Pts',(-4.81880165443801,-13.7899873802489,
4.));
#50745=CARTESIAN_POINT('Ctrl Pts',(-4.80296876416446,-13.6970686989268,
4.));
#50746=CARTESIAN_POINT('Ctrl Pts',(-4.7921064004091,-13.6033902081318,4.));
#50747=CARTESIAN_POINT('Ctrl Pts',(-4.78082403916422,-13.5060896023125,
4.));
#50748=CARTESIAN_POINT('Ctrl Pts',(-4.77490405625791,-13.4079680956598,
4.));
#50749=CARTESIAN_POINT('Ctrl Pts',(-4.77428165528829,-13.3094781487529,
4.));
#50750=CARTESIAN_POINT('Ctrl Pts',(-4.77410059584044,-13.2808269475559,
4.));
#50751=CARTESIAN_POINT('Ctrl Pts',(-4.77436819825548,-13.2521447164312,
4.));
#50752=CARTESIAN_POINT('Ctrl Pts',(-4.77508370765677,-13.2234430275403,
4.));
#50753=CARTESIAN_POINT('Ctrl Pts',(-4.77547928901581,-13.2075748180131,
4.));
#50754=CARTESIAN_POINT('Ctrl Pts',(-4.77601178481995,-13.19170066513,4.));
#50755=CARTESIAN_POINT('Ctrl Pts',(-4.77668111451686,-13.175822557735,4.));
#50756=CARTESIAN_POINT('Ctrl Pts',(-4.77726173830688,-13.1620487674244,
4.));
#50757=CARTESIAN_POINT('Ctrl Pts',(-4.77794533193815,-13.1482734031105,
4.));
#50758=CARTESIAN_POINT('Ctrl Pts',(-4.77873092865176,-13.1345098810533,
4.));
#50759=CARTESIAN_POINT('Ctrl Pts',(-4.78403323232826,-13.0416144140266,
4.));
#50760=CARTESIAN_POINT('Ctrl Pts',(-4.79398378921199,-12.9491067853577,
4.));
#50761=CARTESIAN_POINT('Ctrl Pts',(-4.8084638797429,-12.8573599583,4.));
#50762=CARTESIAN_POINT('Ctrl Pts',(-4.82290323568455,-12.7658712283383,
4.));
#50763=CARTESIAN_POINT('Ctrl Pts',(-4.84184708120934,-12.6751380809488,
4.));
#50764=CARTESIAN_POINT('Ctrl Pts',(-4.86522624014646,-12.5855474359577,
4.));
#50765=CARTESIAN_POINT('Ctrl Pts',(-4.88820176586815,-12.4975035429353,
4.));
#50766=CARTESIAN_POINT('Ctrl Pts',(-4.9154612393753,-12.4105622603287,4.));
#50767=CARTESIAN_POINT('Ctrl Pts',(-4.94697939694318,-12.3251200100783,
4.));
#50768=CARTESIAN_POINT('Ctrl Pts',(-4.96237184169077,-12.2833927894037,
4.));
#50769=CARTESIAN_POINT('Ctrl Pts',(-4.9787805689918,-12.2420236106898,4.));
#50770=CARTESIAN_POINT('Ctrl Pts',(-4.99620574112456,-12.2010620870672,
4.));
#50771=CARTESIAN_POINT('Ctrl Pts',(-5.00196784663073,-12.1875170489459,
4.));
#50772=CARTESIAN_POINT('Ctrl Pts',(-5.00784111328384,-12.1740166075363,
4.));
#50773=CARTESIAN_POINT('Ctrl Pts',(-5.01382559232837,-12.160562620369,4.));
#50774=CARTESIAN_POINT('Ctrl Pts',(-5.01951333079912,-12.1477757495608,
4.));
#50775=CARTESIAN_POINT('Ctrl Pts',(-5.02529810648898,-12.135038576554,4.));
#50776=CARTESIAN_POINT('Ctrl Pts',(-5.0311780316899,-12.1223558509962,4.));
#50777=CARTESIAN_POINT('Ctrl Pts',(-5.06862974733614,-12.0415742398394,
4.));
#50778=CARTESIAN_POINT('Ctrl Pts',(-5.10995835566621,-11.9629538753605,
4.));
#50779=CARTESIAN_POINT('Ctrl Pts',(-5.15509810659155,-11.8868432541903,
4.));
#50780=CARTESIAN_POINT('Ctrl Pts',(-5.19948167106006,-11.8120076471655,
4.));
#50781=CARTESIAN_POINT('Ctrl Pts',(-5.24755020547363,-11.739597730264,4.));
#50782=CARTESIAN_POINT('Ctrl Pts',(-5.29927754869182,-11.6699789932549,
4.));
#50783=CARTESIAN_POINT('Ctrl Pts',(-5.34947355289339,-11.6024212530347,
4.));
#50784=CARTESIAN_POINT('Ctrl Pts',(-5.40311537622297,-11.5374914288171,
4.));
#50785=CARTESIAN_POINT('Ctrl Pts',(-5.46020711675472,-11.4755639671884,
4.));
#50786=CARTESIAN_POINT('Ctrl Pts',(-5.47440621920022,-11.4601621881628,
4.));
#50787=CARTESIAN_POINT('Ctrl Pts',(-5.48881883821923,-11.4449463392586,
4.));
#50788=CARTESIAN_POINT('Ctrl Pts',(-5.50344527039708,-11.4299226339363,
4.));
#50789=CARTESIAN_POINT('Ctrl Pts',(-5.52930152881858,-11.4033640855126,
4.));
#50790=CARTESIAN_POINT('Ctrl Pts',(-5.55582596313967,-11.37740591447,4.));
#50791=CARTESIAN_POINT('Ctrl Pts',(-5.58299257280551,-11.3520616136783,
4.));
#50792=CARTESIAN_POINT('Origin',(-7.50000000000001,-12.9903810567666,14.2084234471775));
#50793=CARTESIAN_POINT('Ctrl Pts',(-10.5771720267767,-12.9888570081198,
11.7084234471775));
#50794=CARTESIAN_POINT('Ctrl Pts',(-10.5778106872988,-12.8899681384638,
11.7032843782051));
#50795=CARTESIAN_POINT('Ctrl Pts',(-10.5289895265855,-11.7846562178796,
11.6458119334487));
#50796=CARTESIAN_POINT('Ctrl Pts',(-9.19520367525283,-9.79242641580684,
11.5360061129082));
#50797=CARTESIAN_POINT('Ctrl Pts',(-5.76804697299906,-9.81262440187857,
11.3790059855559));
#50798=CARTESIAN_POINT('Ctrl Pts',(-3.89395285925593,-12.6818121943635,
11.2220058582037));
#50799=CARTESIAN_POINT('Ctrl Pts',(-5.25343392007517,-15.8279700706855,
11.0650057308514));
#50800=CARTESIAN_POINT('Ctrl Pts',(-8.62743330425189,-16.429494929522,10.9080056034992));
#50801=CARTESIAN_POINT('Ctrl Pts',(-10.4164139750736,-14.5502168635008,
10.7891448422745));
#50802=CARTESIAN_POINT('Ctrl Pts',(-10.5747255939164,-13.2672718029744,
10.7226174568339));
#50803=CARTESIAN_POINT('Ctrl Pts',(-10.5724152591149,-12.9929885813497,
10.7084234471775));
#50804=CARTESIAN_POINT('Ctrl Pts',(-10.5702205181091,-12.9936861301783,
11.7915765528225));
#50805=CARTESIAN_POINT('Ctrl Pts',(-10.5655505854978,-12.3126539838428,
11.7563842836469));
#50806=CARTESIAN_POINT('Ctrl Pts',(-10.0102062672903,-10.6096615213504,
11.6688586386871));
#50807=CARTESIAN_POINT('Ctrl Pts',(-7.21365210721562,-9.38337955935061,
11.5289996179432));
#50808=CARTESIAN_POINT('Ctrl Pts',(-4.33342685529555,-11.2379164301912,
11.371999490591));
#50809=CARTESIAN_POINT('Ctrl Pts',(-4.29152503935676,-14.6655878811314,
11.2149993632387));
#50810=CARTESIAN_POINT('Ctrl Pts',(-7.12729256983938,-16.5902267633183,
11.0579992358865));
#50811=CARTESIAN_POINT('Ctrl Pts',(-9.97678353025252,-15.4189029291823,
10.9168582990811));
#50812=CARTESIAN_POINT('Ctrl Pts',(-10.5660600868159,-13.6932623961271,
10.8280507380598));
#50813=CARTESIAN_POINT('Ctrl Pts',(-10.5715492796759,-12.9879252940133,
10.7915765528226));
#50814=CARTESIAN_POINT('Ctrl Pts',(-5.5865340033349,-11.3543938533917,12.));
#50815=CARTESIAN_POINT('Ctrl Pts',(-5.04858820392145,-11.9835803122485,
11.9476666242159));
#50816=CARTESIAN_POINT('Ctrl Pts',(-4.6501322858494,-13.8032255648209,11.8429998726477));
#50817=CARTESIAN_POINT('Ctrl Pts',(-6.60905294539631,-15.8196542318734,
11.6859997452955));
#50818=CARTESIAN_POINT('Ctrl Pts',(-9.36683654413216,-15.2923247501818,
11.5289996179432));
#50819=CARTESIAN_POINT('Ctrl Pts',(-10.4505966874647,-12.7041316569579,
11.371999490591));
#50820=CARTESIAN_POINT('Ctrl Pts',(-8.88853920691362,-10.3709404162538,
11.2149993632387));
#50821=CARTESIAN_POINT('Ctrl Pts',(-6.08135944510335,-10.3874845613442,
11.0579992358865));
#50822=CARTESIAN_POINT('Ctrl Pts',(-4.54629130410829,-12.737632688099,10.9009991085342));
#50823=CARTESIAN_POINT('Ctrl Pts',(-5.65984053808011,-15.31464666358,10.743998981182));
#50824=CARTESIAN_POINT('Ctrl Pts',(-8.42347920724065,-15.8073549219566,
10.5869988538297));
#50825=CARTESIAN_POINT('Ctrl Pts',(-10.3590248070529,-13.7741141771921,
10.4299987264775));
#50826=CARTESIAN_POINT('Ctrl Pts',(-9.73085564098287,-11.0380625363732,
10.2729985991252));
#50827=CARTESIAN_POINT('Ctrl Pts',(-7.1022567140806,-10.0526889161244,10.115998471773));
#50828=CARTESIAN_POINT('Ctrl Pts',(-4.83031806145553,-11.7015642161036,
9.9589983444207));
#50829=CARTESIAN_POINT('Ctrl Pts',(-4.95230878728804,-14.5061379301299,
9.80199821706846));
#50830=CARTESIAN_POINT('Ctrl Pts',(-7.35883867910848,-15.9515158759806,
9.64499808971619));
#50831=CARTESIAN_POINT('Ctrl Pts',(-9.89194927440413,-14.7416168632348,
9.48799796236395));
#50832=CARTESIAN_POINT('Ctrl Pts',(-10.2801760117029,-11.961367369931,9.33099783501168));
#50833=CARTESIAN_POINT('Ctrl Pts',(-8.17539224562471,-10.1038445935438,
9.17399770765945));
#50834=CARTESIAN_POINT('Ctrl Pts',(-5.46497777443614,-10.8347066168947,
9.01699758030717));
#50835=CARTESIAN_POINT('Ctrl Pts',(-4.57938725553999,-13.4985826621227,
8.85999745295493));
#50836=CARTESIAN_POINT('Ctrl Pts',(-6.31273820393898,-15.7067494160557,
8.70299732560268));
#50837=CARTESIAN_POINT('Ctrl Pts',(-9.11071819481798,-15.4791226211167,
8.54599719825042));
#50838=CARTESIAN_POINT('Ctrl Pts',(-10.4643517279258,-13.0198173800209,
8.38899707089818));
#50839=CARTESIAN_POINT('Ctrl Pts',(-9.15982262789147,-10.5341163103444,
8.23199694354591));
#50840=CARTESIAN_POINT('Ctrl Pts',(-6.3669146537774,-10.2509714005752,8.07499681619367));
#50841=CARTESIAN_POINT('Ctrl Pts',(-4.59005518003756,-12.4242814116226,
7.9179966888414));
#50842=CARTESIAN_POINT('Ctrl Pts',(-5.42257114292002,-15.1052184044673,
7.76099656148916));
#50843=CARTESIAN_POINT('Ctrl Pts',(-8.11793749226372,-15.8897604596585,
7.60399643413691));
#50844=CARTESIAN_POINT('Ctrl Pts',(-10.259193363348,-14.0744011876836,7.44699630678465));
#50845=CARTESIAN_POINT('Ctrl Pts',(-9.92625407643148,-11.286990666814,7.2899961794324));
#50846=CARTESIAN_POINT('Ctrl Pts',(-7.4176694799797,-10.0270266461848,7.13299605208014));
#50847=CARTESIAN_POINT('Ctrl Pts',(-4.98291145609725,-11.4243309624572,
6.97599592472789));
#50848=CARTESIAN_POINT('Ctrl Pts',(-4.80525086677252,-14.2259274070742,
6.81899579737564));
#50849=CARTESIAN_POINT('Ctrl Pts',(-7.04399769823543,-15.9195976158556,
6.66199567002339));
#50850=CARTESIAN_POINT('Ctrl Pts',(-9.69164612773492,-14.986611176204,6.50499554267113));
#50851=CARTESIAN_POINT('Ctrl Pts',(-10.3740245283272,-12.2635861515028,
6.34799541531888));
#50852=CARTESIAN_POINT('Ctrl Pts',(-8.47923740659063,-10.1922848677994,
6.19099528796662));
#50853=CARTESIAN_POINT('Ctrl Pts',(-5.70635901253982,-10.630063717047,6.03399516061437));
#50854=CARTESIAN_POINT('Ctrl Pts',(-4.54185510339179,-13.1843609143513,
5.87699503326211));
#50855=CARTESIAN_POINT('Ctrl Pts',(-6.02994926840226,-15.5647161841919,
5.71999490590987));
#50856=CARTESIAN_POINT('Ctrl Pts',(-8.83624974536451,-15.636637176778,5.5629947785576));
#50857=CARTESIAN_POINT('Ctrl Pts',(-10.4443267219795,-13.3356413212244,
5.40599465120536));
#50858=CARTESIAN_POINT('Ctrl Pts',(-9.41218894167164,-10.7250347470945,
5.2489945238531));
#50859=CARTESIAN_POINT('Ctrl Pts',(-6.66539009301951,-10.1458104553331,
5.09199439650085));
#50860=CARTESIAN_POINT('Ctrl Pts',(-4.66696049204361,-12.1172919418034,
4.93499426914859));
#50861=CARTESIAN_POINT('Ctrl Pts',(-5.20901007842283,-14.8717746831197,
4.77799414179635));
#50862=CARTESIAN_POINT('Ctrl Pts',(-7.80528416826264,-15.9390100206221,
4.62099401444409));
#50863=CARTESIAN_POINT('Ctrl Pts',(-10.1280577671037,-14.362540949444,4.46399388709183));
#50864=CARTESIAN_POINT('Ctrl Pts',(-10.0937360173612,-11.5549393117934,
4.30699375973958));
#50865=CARTESIAN_POINT('Ctrl Pts',(-7.73454717783886,-10.0358910717557,
4.14999363238733));
#50866=CARTESIAN_POINT('Ctrl Pts',(-5.16315103760592,-11.163440915316,3.99299350503507));
#50867=CARTESIAN_POINT('Ctrl Pts',(-4.69098959926211,-13.9347976761557,
3.83599337768283));
#50868=CARTESIAN_POINT('Ctrl Pts',(-6.05008049550027,-15.2086689018369,
3.73132662611465));
#50869=CARTESIAN_POINT('Ctrl Pts',(-6.84980000202495,-15.4224678588017,
3.67899325033057));
#50870=CARTESIAN_POINT('Ctrl Pts',(-5.44566844965787,-11.2339557355398,
12.1070022498898));
#50871=CARTESIAN_POINT('Ctrl Pts',(-4.86812015246569,-11.9094616477066,
12.0546688741057));
#50872=CARTESIAN_POINT('Ctrl Pts',(-4.44033070371531,-13.8630655577342,
11.9500021225376));
#50873=CARTESIAN_POINT('Ctrl Pts',(-6.54346319864229,-16.0279396850822,
11.7930019951853));
#50874=CARTESIAN_POINT('Ctrl Pts',(-9.50426933043305,-15.4617892577673,
11.6360018678331));
#50875=CARTESIAN_POINT('Ctrl Pts',(-10.6678137358898,-12.6830585465582,
11.4790017404808));
#50876=CARTESIAN_POINT('Ctrl Pts',(-8.99076069636001,-10.1781024161048,
11.3220016131285));
#50877=CARTESIAN_POINT('Ctrl Pts',(-5.97692195440192,-10.195864508189,11.1650014857763));
#50878=CARTESIAN_POINT('Ctrl Pts',(-4.32884515582416,-12.7190258568539,
11.008001358424));
#50879=CARTESIAN_POINT('Ctrl Pts',(-5.52437166541181,-15.4857544659485,
10.8510012310718));
#50880=CARTESIAN_POINT('Ctrl Pts',(-8.49146390624439,-16.0147349244784,
10.6940011037195));
#50881=CARTESIAN_POINT('Ctrl Pts',(-10.569500516119,-13.831811047759,10.5370009763673));
#50882=CARTESIAN_POINT('Ctrl Pts',(-9.89508678780663,-10.8943367373214,
10.380000849015));
#50883=CARTESIAN_POINT('Ctrl Pts',(-7.07297564596128,-9.83642187472128,
10.2230007216628));
#50884=CARTESIAN_POINT('Ctrl Pts',(-4.6337813970622,-11.606684088542,10.0660005943105));
#50885=CARTESIAN_POINT('Ctrl Pts',(-4.76475283703741,-14.6177249306714,
9.90900046695826));
#50886=CARTESIAN_POINT('Ctrl Pts',(-7.34844666395912,-16.1695087206656,
9.75200033960601));
#50887=CARTESIAN_POINT('Ctrl Pts',(-10.0680398135062,-14.8705393535885,
9.59500021225375));
#50888=CARTESIAN_POINT('Ctrl Pts',(-10.4848470295787,-11.8856134328399,
9.43800008490151));
#50889=CARTESIAN_POINT('Ctrl Pts',(-8.22511327688156,-9.89134353117351,
9.28099995754925));
#50890=CARTESIAN_POINT('Ctrl Pts',(-5.31516349341482,-10.6760101602818,
9.123999830197));
#50891=CARTESIAN_POINT('Ctrl Pts',(-4.36437756524938,-13.5359954516068,
8.96699970284473));
#50892=CARTESIAN_POINT('Ctrl Pts',(-6.22533435639049,-15.9067230417114,
8.80999957549251));
#50893=CARTESIAN_POINT('Ctrl Pts',(-9.22929605861391,-15.6623388157249,
8.65299944814021));
#50894=CARTESIAN_POINT('Ctrl Pts',(-10.6825813950197,-13.0219844234806,
8.495999320788));
#50895=CARTESIAN_POINT('Ctrl Pts',(-9.28201546219901,-10.3532909943549,
8.33899919343572));
#50896=CARTESIAN_POINT('Ctrl Pts',(-6.28349916850765,-10.0493015205563,
8.18199906608348));
#50897=CARTESIAN_POINT('Ctrl Pts',(-4.37583084109032,-12.3826062838239,
8.02499893873122));
#50898=CARTESIAN_POINT('Ctrl Pts',(-5.26963497019092,-15.2609085157313,
7.86799881137897));
#50899=CARTESIAN_POINT('Ctrl Pts',(-8.16342881906923,-16.1032069936549,
7.71099868402671));
#50900=CARTESIAN_POINT('Ctrl Pts',(-10.4623196804644,-14.1542045895756,
7.55399855667447));
#50901=CARTESIAN_POINT('Ctrl Pts',(-10.1048700666991,-11.1615904606817,
7.3969984293222));
#50902=CARTESIAN_POINT('Ctrl Pts',(-7.41160847115729,-9.80887039960631,
7.23999830196995));
#50903=CARTESIAN_POINT('Ctrl Pts',(-4.79760841334188,-11.3090414752098,
7.08299817461771));
#50904=CARTESIAN_POINT('Ctrl Pts',(-4.60686880545846,-14.3168858672889,
6.92599804726544));
#50905=CARTESIAN_POINT('Ctrl Pts',(-7.01042771746335,-16.1352407018342,
6.7689979199132));
#50906=CARTESIAN_POINT('Ctrl Pts',(-9.85299074832685,-15.133569659674,6.61199779256094));
#50907=CARTESIAN_POINT('Ctrl Pts',(-10.5856044869832,-12.2100809588743,
6.45499766520869));
#50908=CARTESIAN_POINT('Ctrl Pts',(-8.55132691312017,-9.98629460218332,
6.29799753785643));
#50909=CARTESIAN_POINT('Ctrl Pts',(-5.57431473726304,-10.4563018579429,
6.14099741050418));
#50910=CARTESIAN_POINT('Ctrl Pts',(-4.32408237085103,-13.1986413249196,
5.98399728315193));
#50911=CARTESIAN_POINT('Ctrl Pts',(-5.92172706293806,-15.75423360635,5.82699715579966));
#50912=CARTESIAN_POINT('Ctrl Pts',(-8.9346217888498,-15.831449279092,5.66999702844743));
#50913=CARTESIAN_POINT('Ctrl Pts',(-10.6610821880398,-13.3610586938876,
5.51299690109516));
#50914=CARTESIAN_POINT('Ctrl Pts',(-9.55296048110486,-10.558264465972,5.35599677374292));
#50915=CARTESIAN_POINT('Ctrl Pts',(-6.60394777480949,-9.93639883608159,
5.19899664639066));
#50916=CARTESIAN_POINT('Ctrl Pts',(-4.45839776891566,-12.0530168609799,
5.04199651903841));
#50917=CARTESIAN_POINT('Ctrl Pts',(-5.04035196569236,-15.0102791328056,
4.88499639168615));
#50918=CARTESIAN_POINT('Ctrl Pts',(-7.82775858038497,-16.1560822091562,
4.72799626433391));
#50919=CARTESIAN_POINT('Ctrl Pts',(-10.3215301429408,-14.4635566264157,
4.57099613698164));
#50920=CARTESIAN_POINT('Ctrl Pts',(-10.2846816943758,-11.4492649509585,
4.4139960096294));
#50921=CARTESIAN_POINT('Ctrl Pts',(-7.75181407368507,-9.81838740652354,
4.25699588227714));
#50922=CARTESIAN_POINT('Ctrl Pts',(-4.99111687367461,-11.0289452226782,
4.09999575492489));
#50923=CARTESIAN_POINT('Ctrl Pts',(-4.48419585112438,-14.0043237457194,
3.94299562757263));
#50924=CARTESIAN_POINT('Ctrl Pts',(-5.94334031085918,-15.3719748325696,
3.83832887600446));
#50925=CARTESIAN_POINT('Ctrl Pts',(-6.80193357383903,-15.6015132427052,
3.78599550022038));
#50926=CARTESIAN_POINT('Ctrl Pts',(-5.30480289598084,-11.1135176176879,
12.2140044997796));
#50927=CARTESIAN_POINT('Ctrl Pts',(-4.68765210100992,-11.8353429831648,
12.1616711239955));
#50928=CARTESIAN_POINT('Ctrl Pts',(-4.23052912158122,-13.9229055506476,
12.0570043724274));
#50929=CARTESIAN_POINT('Ctrl Pts',(-6.47787345188828,-16.2362251382909,
11.9000042450751));
#50930=CARTESIAN_POINT('Ctrl Pts',(-9.64170211673396,-15.6312537653527,
11.7430041177229));
#50931=CARTESIAN_POINT('Ctrl Pts',(-10.8850307843148,-12.6619854361585,
11.5860039903706));
#50932=CARTESIAN_POINT('Ctrl Pts',(-9.09298218580643,-9.98526441595581,
11.4290038630183));
#50933=CARTESIAN_POINT('Ctrl Pts',(-5.87248446370049,-10.0042444550338,
11.2720037356661));
#50934=CARTESIAN_POINT('Ctrl Pts',(-4.11139900754004,-12.7004190256087,
11.1150036083138));
#50935=CARTESIAN_POINT('Ctrl Pts',(-5.3889027927435,-15.656862268317,10.9580034809616));
#50936=CARTESIAN_POINT('Ctrl Pts',(-8.55944860524813,-16.2221149270002,
10.8010033536093));
#50937=CARTESIAN_POINT('Ctrl Pts',(-10.7799762251851,-13.889507918326,10.6440032262571));
#50938=CARTESIAN_POINT('Ctrl Pts',(-10.0593179346304,-10.7506109382696,
10.4870030989048));
#50939=CARTESIAN_POINT('Ctrl Pts',(-7.04369457784195,-9.62015483331818,
10.3300029715526));
#50940=CARTESIAN_POINT('Ctrl Pts',(-4.43724473266885,-11.5118039609805,
10.1730028442003));
#50941=CARTESIAN_POINT('Ctrl Pts',(-4.57719688678678,-14.7293119312129,
10.0160027168481));
#50942=CARTESIAN_POINT('Ctrl Pts',(-7.33805464880973,-16.3875015653505,
9.85900258949582));
#50943=CARTESIAN_POINT('Ctrl Pts',(-10.2441303526083,-14.9994618439422,
9.70200246214357));
#50944=CARTESIAN_POINT('Ctrl Pts',(-10.6895180474545,-11.8098594957488,
9.5450023347913));
#50945=CARTESIAN_POINT('Ctrl Pts',(-8.2748343081384,-9.6788424688032,9.38800220743907));
#50946=CARTESIAN_POINT('Ctrl Pts',(-5.1653492123935,-10.517313703669,9.2310020800868));
#50947=CARTESIAN_POINT('Ctrl Pts',(-4.14936787495879,-13.5734082410908,
9.07400195273456));
#50948=CARTESIAN_POINT('Ctrl Pts',(-6.137930508842,-16.1066966673671,8.9170018253823));
#50949=CARTESIAN_POINT('Ctrl Pts',(-9.34787392240984,-15.8455550103332,
8.76000169803005));
#50950=CARTESIAN_POINT('Ctrl Pts',(-10.9008110621136,-13.0241514669403,
8.60300157067779));
#50951=CARTESIAN_POINT('Ctrl Pts',(-9.40420829650654,-10.1724656783654,
8.44600144332554));
#50952=CARTESIAN_POINT('Ctrl Pts',(-6.20008368323791,-9.84763164053746,
8.28900131597328));
#50953=CARTESIAN_POINT('Ctrl Pts',(-4.16160650214306,-12.3409311560251,
8.13200118862103));
#50954=CARTESIAN_POINT('Ctrl Pts',(-5.11669879746183,-15.4165986269953,
7.97500106126878));
#50955=CARTESIAN_POINT('Ctrl Pts',(-8.20892014587475,-16.3166535276513,
7.81800093391653));
#50956=CARTESIAN_POINT('Ctrl Pts',(-10.6654459975808,-14.2340079914677,
7.66100080656427));
#50957=CARTESIAN_POINT('Ctrl Pts',(-10.2834860569666,-11.0361902545495,
7.50400067921202));
#50958=CARTESIAN_POINT('Ctrl Pts',(-7.40554746233487,-9.59071415302789,
7.34700055185976));
#50959=CARTESIAN_POINT('Ctrl Pts',(-4.61230537058651,-11.1937519879624,
7.19000042450751));
#50960=CARTESIAN_POINT('Ctrl Pts',(-4.40848674414439,-14.4078443275035,
7.03300029715526));
#50961=CARTESIAN_POINT('Ctrl Pts',(-6.97685773669127,-16.3508837878128,
6.876000169803));
#50962=CARTESIAN_POINT('Ctrl Pts',(-10.0143353689188,-15.280528143144,6.71900004245075));
#50963=CARTESIAN_POINT('Ctrl Pts',(-10.7971844456393,-12.1565757662458,
6.5619999150985));
#50964=CARTESIAN_POINT('Ctrl Pts',(-8.62341641964973,-9.78030433656719,
6.40499978774624));
#50965=CARTESIAN_POINT('Ctrl Pts',(-5.44227046198626,-10.2825399988388,
6.24799966039399));
#50966=CARTESIAN_POINT('Ctrl Pts',(-4.10630963831026,-13.2129217354879,
6.09099953304174));
#50967=CARTESIAN_POINT('Ctrl Pts',(-5.81350485747386,-15.943751028508,5.93399940568949));
#50968=CARTESIAN_POINT('Ctrl Pts',(-9.0329938323351,-16.026261381406,5.77699927833723));
#50969=CARTESIAN_POINT('Ctrl Pts',(-10.8778376541001,-13.3864760665508,
5.61999915098497));
#50970=CARTESIAN_POINT('Ctrl Pts',(-9.69373202053811,-10.3914941848495,
5.46299902363273));
#50971=CARTESIAN_POINT('Ctrl Pts',(-6.54250545659946,-9.72698721683007,
5.30599889628047));
#50972=CARTESIAN_POINT('Ctrl Pts',(-4.24983504578773,-11.9887417801564,
5.14899876892822));
#50973=CARTESIAN_POINT('Ctrl Pts',(-4.87169385296189,-15.1487835824914,
4.99199864157596));
#50974=CARTESIAN_POINT('Ctrl Pts',(-7.85023299250732,-16.3731543976903,
4.83499851422371));
#50975=CARTESIAN_POINT('Ctrl Pts',(-10.5150025187778,-14.5645723033874,
4.67799838687146));
#50976=CARTESIAN_POINT('Ctrl Pts',(-10.4756273713904,-11.3435905901237,
4.5209982595192));
#50977=CARTESIAN_POINT('Ctrl Pts',(-7.76908096953125,-9.60088374129137,
4.36399813216695));
#50978=CARTESIAN_POINT('Ctrl Pts',(-4.81908270974332,-10.8944495300405,
4.2069980048147));
#50979=CARTESIAN_POINT('Ctrl Pts',(-4.27740210298664,-14.0738498152832,
4.04999787746244));
#50980=CARTESIAN_POINT('Ctrl Pts',(-5.83660012621808,-15.5352807633023,
3.94533112589427));
#50981=CARTESIAN_POINT('Ctrl Pts',(-6.75406714565312,-15.7805586266087,
3.89299775011019));
#50982=CARTESIAN_POINT('Ctrl Pts',(-5.1639373423038,-10.993079499836,12.3210067496694));
#50983=CARTESIAN_POINT('Ctrl Pts',(-4.50718404955416,-11.761224318623,12.2686733738853));
#50984=CARTESIAN_POINT('Ctrl Pts',(-4.02072753944713,-13.9827455435609,
12.1640066223172));
#50985=CARTESIAN_POINT('Ctrl Pts',(-6.41228370513427,-16.4445105914997,
12.0070064949649));
#50986=CARTESIAN_POINT('Ctrl Pts',(-9.77913490303484,-15.8007182729381,
11.8500063676127));
#50987=CARTESIAN_POINT('Ctrl Pts',(-11.1022478327399,-12.6409123257588,
11.6930062402604));
#50988=CARTESIAN_POINT('Ctrl Pts',(-9.19520367525283,-9.79242641580684,
11.5360061129082));
#50989=CARTESIAN_POINT('Ctrl Pts',(-5.76804697299906,-9.81262440187857,
11.3790059855559));
#50990=CARTESIAN_POINT('Ctrl Pts',(-3.89395285925593,-12.6818121943635,
11.2220058582037));
#50991=CARTESIAN_POINT('Ctrl Pts',(-5.25343392007517,-15.8279700706855,
11.0650057308514));
#50992=CARTESIAN_POINT('Ctrl Pts',(-8.62743330425189,-16.429494929522,10.9080056034992));
#50993=CARTESIAN_POINT('Ctrl Pts',(-10.9904519342511,-13.9472047888929,
10.7510054761469));
#50994=CARTESIAN_POINT('Ctrl Pts',(-10.2235490814542,-10.6068851392178,
10.5940053487946));
#50995=CARTESIAN_POINT('Ctrl Pts',(-7.01441350972263,-9.40388779191504,
10.4370052214424));
#50996=CARTESIAN_POINT('Ctrl Pts',(-4.2407080682755,-11.4169238334189,10.2800050940901));
#50997=CARTESIAN_POINT('Ctrl Pts',(-4.38964093653616,-14.8408989317544,
10.1230049667379));
#50998=CARTESIAN_POINT('Ctrl Pts',(-7.32766263366035,-16.6054944100355,
9.96600483938563));
#50999=CARTESIAN_POINT('Ctrl Pts',(-10.4202208917104,-15.1283843342959,
9.80900471203338));
#51000=CARTESIAN_POINT('Ctrl Pts',(-10.8941890653303,-11.7341055586577,
9.65200458468112));
#51001=CARTESIAN_POINT('Ctrl Pts',(-8.32455533939524,-9.46634140643289,
9.49500445732887));
#51002=CARTESIAN_POINT('Ctrl Pts',(-5.01553493137219,-10.3586172470561,
9.33800432997662));
#51003=CARTESIAN_POINT('Ctrl Pts',(-3.93435818466818,-13.6108210305748,
9.18100420262436));
#51004=CARTESIAN_POINT('Ctrl Pts',(-6.05052666129351,-16.3066702930228,
9.02400407527212));
#51005=CARTESIAN_POINT('Ctrl Pts',(-9.46645178620579,-16.0287712049414,
8.86700394791984));
#51006=CARTESIAN_POINT('Ctrl Pts',(-11.1190407292075,-13.0263185104,8.71000382056762));
#51007=CARTESIAN_POINT('Ctrl Pts',(-9.52640113081409,-9.99164036237588,
8.55300369321534));
#51008=CARTESIAN_POINT('Ctrl Pts',(-6.11666819796815,-9.64596176051859,
8.3960035658631));
#51009=CARTESIAN_POINT('Ctrl Pts',(-3.94738216319582,-12.2992560282264,
8.23900343851084));
#51010=CARTESIAN_POINT('Ctrl Pts',(-4.96376262473273,-15.5722887382593,
8.0820033111586));
#51011=CARTESIAN_POINT('Ctrl Pts',(-8.25441147268027,-16.5301000616477,
7.92500318380633));
#51012=CARTESIAN_POINT('Ctrl Pts',(-10.8685723146971,-14.3138113933598,
7.76800305645408));
#51013=CARTESIAN_POINT('Ctrl Pts',(-10.4621020472342,-10.9107900484173,
7.61100292910183));
#51014=CARTESIAN_POINT('Ctrl Pts',(-7.39948645351245,-9.37255790644949,
7.45400280174957));
#51015=CARTESIAN_POINT('Ctrl Pts',(-4.42700232783115,-11.078462500715,7.29700267439732));
#51016=CARTESIAN_POINT('Ctrl Pts',(-4.21010468283033,-14.4988027877182,
7.14000254704507));
#51017=CARTESIAN_POINT('Ctrl Pts',(-6.94328775591919,-16.5665268737914,
6.98300241969282));
#51018=CARTESIAN_POINT('Ctrl Pts',(-10.1756799895107,-15.427486626614,6.82600229234056));
#51019=CARTESIAN_POINT('Ctrl Pts',(-11.0087644042953,-12.1030705736173,
6.66900216498831));
#51020=CARTESIAN_POINT('Ctrl Pts',(-8.69550592617927,-9.57431407095109,
6.51200203763606));
#51021=CARTESIAN_POINT('Ctrl Pts',(-5.31022618670948,-10.1087781397346,
6.3550019102838));
#51022=CARTESIAN_POINT('Ctrl Pts',(-3.88853690576949,-13.2272021460562,
6.19800178293155));
#51023=CARTESIAN_POINT('Ctrl Pts',(-5.70528265200966,-16.133268450666,6.0410016555793));
#51024=CARTESIAN_POINT('Ctrl Pts',(-9.13136587582039,-16.22107348372,5.88400152822704));
#51025=CARTESIAN_POINT('Ctrl Pts',(-11.0945931201605,-13.4118934392139,
5.72700140087479));
#51026=CARTESIAN_POINT('Ctrl Pts',(-9.83450355997132,-10.224723903727,5.57000127352253));
#51027=CARTESIAN_POINT('Ctrl Pts',(-6.48106313838945,-9.51757559757857,
5.41300114617028));
#51028=CARTESIAN_POINT('Ctrl Pts',(-4.04127232265978,-11.9244666993329,
5.25600101881803));
#51029=CARTESIAN_POINT('Ctrl Pts',(-4.70303574023142,-15.2872880321773,
5.09900089146577));
#51030=CARTESIAN_POINT('Ctrl Pts',(-7.87270740462966,-16.5902265862243,
4.94200076411352));
#51031=CARTESIAN_POINT('Ctrl Pts',(-10.7084748946149,-14.6655879803591,
4.78500063676127));
#51032=CARTESIAN_POINT('Ctrl Pts',(-10.666573048405,-11.2379162292888,4.62800050940902));
#51033=CARTESIAN_POINT('Ctrl Pts',(-7.78634786537746,-9.38338007605921,
4.47100038205676));
#51034=CARTESIAN_POINT('Ctrl Pts',(-4.64704854581202,-10.7599538374027,
4.31400025470451));
#51035=CARTESIAN_POINT('Ctrl Pts',(-4.0706083548489,-14.143375884847,4.15700012735225));
#51036=CARTESIAN_POINT('Ctrl Pts',(-5.72985994157699,-15.6985866940351,
4.05233337578409));
#51037=CARTESIAN_POINT('Ctrl Pts',(-6.7062007174672,-15.9596040105123,4.));
#51038=CARTESIAN_POINT('Ctrl Pts',(-5.5865340033349,-11.3543938533917,12.));
#51039=CARTESIAN_POINT('Ctrl Pts',(-5.52489675159201,-11.412317734857,12.));
#51040=CARTESIAN_POINT('Ctrl Pts',(-5.46662466733851,-11.4733903391465,
12.));
#51041=CARTESIAN_POINT('Ctrl Pts',(-5.41171731080853,-11.5372273647712,
12.));
#51042=CARTESIAN_POINT('Ctrl Pts',(-5.35535954826471,-11.6027506782036,
12.));
#51043=CARTESIAN_POINT('Ctrl Pts',(-5.30254618320446,-11.6711868211063,
12.));
#51044=CARTESIAN_POINT('Ctrl Pts',(-5.25330217107373,-11.7421687765855,
12.));
#51045=CARTESIAN_POINT('Ctrl Pts',(-5.20312956815832,-11.8144892336791,
12.));
#51046=CARTESIAN_POINT('Ctrl Pts',(-5.1566617252503,-11.8894530177238,12.));
#51047=CARTESIAN_POINT('Ctrl Pts',(-5.11395808422126,-11.9667137220828,
12.));
#51048=CARTESIAN_POINT('Ctrl Pts',(-5.09461562078295,-12.0017086853522,
12.));
#51049=CARTESIAN_POINT('Ctrl Pts',(-5.07604591099636,-12.0371753912937,
12.));
#51050=CARTESIAN_POINT('Ctrl Pts',(-5.05825705836343,-12.0730838611618,
12.));
#51051=CARTESIAN_POINT('Ctrl Pts',(-5.04815218455416,-12.093481498052,12.));
#51052=CARTESIAN_POINT('Ctrl Pts',(-5.03829930483427,-12.1140217037901,
12.));
#51053=CARTESIAN_POINT('Ctrl Pts',(-5.02870015601257,-12.1346991425122,
12.));
#51054=CARTESIAN_POINT('Ctrl Pts',(-5.02048318017586,-12.1523992550431,
12.));
#51055=CARTESIAN_POINT('Ctrl Pts',(-5.01244999988763,-12.1702050672847,
12.));
#51056=CARTESIAN_POINT('Ctrl Pts',(-5.00461448908043,-12.1880835326347,
12.));
#51057=CARTESIAN_POINT('Ctrl Pts',(-4.96800851502513,-12.2716082261557,
12.));
#51058=CARTESIAN_POINT('Ctrl Pts',(-4.93566438777708,-12.3568162975634,
12.));
#51059=CARTESIAN_POINT('Ctrl Pts',(-4.9076092477584,-12.4433098844385,12.));
#51060=CARTESIAN_POINT('Ctrl Pts',(-4.87909470826589,-12.531219793181,12.));
#51061=CARTESIAN_POINT('Ctrl Pts',(-4.85501027288513,-12.6204584164563,
12.));
#51062=CARTESIAN_POINT('Ctrl Pts',(-4.83542346103633,-12.7106451238744,
12.));
#51063=CARTESIAN_POINT('Ctrl Pts',(-4.81671890332471,-12.7967695266993,
12.));
#51064=CARTESIAN_POINT('Ctrl Pts',(-4.80211587003395,-12.8837594508039,
12.));
#51065=CARTESIAN_POINT('Ctrl Pts',(-4.79171175017421,-12.9713041908118,
12.));
#51066=CARTESIAN_POINT('Ctrl Pts',(-4.7871219669274,-13.0099246014234,12.));
#51067=CARTESIAN_POINT('Ctrl Pts',(-4.78334987321312,-13.0486531860177,
12.));
#51068=CARTESIAN_POINT('Ctrl Pts',(-4.78040642509842,-13.0874639619222,
12.));
#51069=CARTESIAN_POINT('Ctrl Pts',(-4.7790340847621,-13.1055589278201,12.));
#51070=CARTESIAN_POINT('Ctrl Pts',(-4.77784189531648,-13.1236717640034,
12.));
#51071=CARTESIAN_POINT('Ctrl Pts',(-4.77683109303951,-13.1417998520234,
12.));
#51072=CARTESIAN_POINT('Ctrl Pts',(-4.7758570840318,-13.1592680764492,12.));
#51073=CARTESIAN_POINT('Ctrl Pts',(-4.77505149943043,-13.1767532882224,
12.));
#51074=CARTESIAN_POINT('Ctrl Pts',(-4.77441609878784,-13.1942285673893,
12.));
#51075=CARTESIAN_POINT('Ctrl Pts',(-4.77095265346117,-13.2894829154418,
12.));
#51076=CARTESIAN_POINT('Ctrl Pts',(-4.77253183089421,-13.3845892743107,
12.));
#51077=CARTESIAN_POINT('Ctrl Pts',(-4.77921580433521,-13.4791489989792,
12.));
#51078=CARTESIAN_POINT('Ctrl Pts',(-4.78586481725455,-13.5732141290278,
12.));
#51079=CARTESIAN_POINT('Ctrl Pts',(-4.79756501411883,-13.6667392834721,
12.));
#51080=CARTESIAN_POINT('Ctrl Pts',(-4.81442558423848,-13.7593498298833,
12.));
#51081=CARTESIAN_POINT('Ctrl Pts',(-4.830924328857,-13.8499729667865,12.));
#51082=CARTESIAN_POINT('Ctrl Pts',(-4.85236399681968,-13.9397212614334,
12.));
#51083=CARTESIAN_POINT('Ctrl Pts',(-4.87847000308199,-14.0283529813775,
12.));
#51084=CARTESIAN_POINT('Ctrl Pts',(-4.89379441408366,-14.0803804301784,
12.));
#51085=CARTESIAN_POINT('Ctrl Pts',(-4.91072775850773,-14.1320231162836,
12.));
#51086=CARTESIAN_POINT('Ctrl Pts',(-4.92922261500886,-14.1832309956159,
12.));
#51087=CARTESIAN_POINT('Ctrl Pts',(-4.93398351814407,-14.1964128093404,
12.));
#51088=CARTESIAN_POINT('Ctrl Pts',(-4.93884875001307,-14.2095679810762,
12.));
#51089=CARTESIAN_POINT('Ctrl Pts',(-4.94381485137731,-14.2226885070165,
12.));
#51090=CARTESIAN_POINT('Ctrl Pts',(-4.97686325186981,-14.310002954335,12.));
#51091=CARTESIAN_POINT('Ctrl Pts',(-5.01429440116268,-14.3955759829307,
12.));
#51092=CARTESIAN_POINT('Ctrl Pts',(-5.05577732713123,-14.4791717978631,
12.));
#51093=CARTESIAN_POINT('Ctrl Pts',(-5.09882663969929,-14.5659241732654,
12.));
#51094=CARTESIAN_POINT('Ctrl Pts',(-5.1462396027634,-14.6505479156747,12.));
#51095=CARTESIAN_POINT('Ctrl Pts',(-5.19770241499811,-14.7327775666312,
12.));
#51096=CARTESIAN_POINT('Ctrl Pts',(-5.24979009521262,-14.8160056604173,
12.));
#51097=CARTESIAN_POINT('Ctrl Pts',(-5.30602696260126,-14.8967819927061,
12.));
#51098=CARTESIAN_POINT('Ctrl Pts',(-5.36613986514052,-14.9748175661494,
12.));
#51099=CARTESIAN_POINT('Ctrl Pts',(-5.40561376259492,-15.0260606120477,
12.));
#51100=CARTESIAN_POINT('Ctrl Pts',(-5.44676008901899,-15.076121523717,12.));
#51101=CARTESIAN_POINT('Ctrl Pts',(-5.48951221838806,-15.1249126475777,
12.));
#51102=CARTESIAN_POINT('Ctrl Pts',(-5.50097170290556,-15.1379908529612,
12.));
#51103=CARTESIAN_POINT('Ctrl Pts',(-5.51254660460158,-15.1509777948558,
12.));
#51104=CARTESIAN_POINT('Ctrl Pts',(-5.52423573327417,-15.1638717111488,
12.));
#51105=CARTESIAN_POINT('Ctrl Pts',(-5.5353884173992,-15.1761738920537,12.));
#51106=CARTESIAN_POINT('Ctrl Pts',(-5.54663940936984,-15.1883850930378,
12.));
#51107=CARTESIAN_POINT('Ctrl Pts',(-5.55798428070717,-15.2005008010861,
12.));
#51108=CARTESIAN_POINT('Ctrl Pts',(-5.62980603833238,-15.2772025477193,
12.));
#51109=CARTESIAN_POINT('Ctrl Pts',(-5.70542358612169,-15.3501207786779,
12.));
#51110=CARTESIAN_POINT('Ctrl Pts',(-5.7844933991545,-15.4189223872958,12.));
#51111=CARTESIAN_POINT('Ctrl Pts',(-5.8437957589291,-15.4705235937591,12.));
#51112=CARTESIAN_POINT('Ctrl Pts',(-5.90504133108183,-15.519808942512,12.));
#51113=CARTESIAN_POINT('Ctrl Pts',(-5.968104244788,-15.5666263507592,12.));
#51114=CARTESIAN_POINT('Ctrl Pts',(-5.99074690383604,-15.5834360817113,
12.));
#51115=CARTESIAN_POINT('Ctrl Pts',(-6.01362398614045,-15.5999275418789,
12.));
#51116=CARTESIAN_POINT('Ctrl Pts',(-6.03673011024537,-15.6160932756601,
12.));
#51117=CARTESIAN_POINT('Ctrl Pts',(-6.05604444624562,-15.6296061613575,
12.));
#51118=CARTESIAN_POINT('Ctrl Pts',(-6.07552135620629,-15.6428929845117,
12.));
#51119=CARTESIAN_POINT('Ctrl Pts',(-6.09513705214722,-15.655935902686,12.));
#51120=CARTESIAN_POINT('Ctrl Pts',(-6.1801078936968,-15.7124349296322,12.));
#51121=CARTESIAN_POINT('Ctrl Pts',(-6.26775546621735,-15.7644144018326,
12.));
#51122=CARTESIAN_POINT('Ctrl Pts',(-6.3577924589883,-15.8115622787044,12.));
#51123=CARTESIAN_POINT('Ctrl Pts',(-6.42986829724945,-15.8493047958986,
12.));
#51124=CARTESIAN_POINT('Ctrl Pts',(-6.50347629812978,-15.8839507974289,
12.));
#51125=CARTESIAN_POINT('Ctrl Pts',(-6.57848586659695,-15.9153228867674,
12.));
#51126=CARTESIAN_POINT('Ctrl Pts',(-6.61998922672564,-15.9326813004793,
12.));
#51127=CARTESIAN_POINT('Ctrl Pts',(-6.66192191928759,-15.9490371078547,
12.));
#51128=CARTESIAN_POINT('Ctrl Pts',(-6.70425049788235,-15.9643995452955,
12.));
#51129=CARTESIAN_POINT('Ctrl Pts',(-10.0166114900998,-12.9925168768863,
10.387416697508));
#51130=CARTESIAN_POINT('Ctrl Pts',(-10.0185038824417,-13.21718192014,10.4016107071645));
#51131=CARTESIAN_POINT('Ctrl Pts',(-9.99083741615502,-13.441388813634,10.415804716821));
#51132=CARTESIAN_POINT('Ctrl Pts',(-9.93173901273922,-13.6569790278497,
10.4299987264775));
#51133=CARTESIAN_POINT('Ctrl Pts',(-9.71384294044885,-14.4518610921136,
10.4823321022616));
#51134=CARTESIAN_POINT('Ctrl Pts',(-9.06866107384475,-15.1296080070351,
10.5346654780456));
#51135=CARTESIAN_POINT('Ctrl Pts',(-8.28546369568261,-15.3863634214331,
10.5869988538297));
#51136=CARTESIAN_POINT('Ctrl Pts',(-7.50226631752047,-15.6431188358311,
10.6393322296138));
#51137=CARTESIAN_POINT('Ctrl Pts',(-6.58105342780029,-15.4788827497055,
10.6916656053979));
#51138=CARTESIAN_POINT('Ctrl Pts',(-5.9348554439449,-14.9672623773959,10.743998981182));
#51139=CARTESIAN_POINT('Ctrl Pts',(-5.2886574600895,-14.4556420050863,10.7963323569661));
#51140=CARTESIAN_POINT('Ctrl Pts',(-4.91747438209889,-13.5966373465927,
10.8486657327501));
#51141=CARTESIAN_POINT('Ctrl Pts',(-4.98772753326943,-12.7754436628867,
10.9009991085342));
#51142=CARTESIAN_POINT('Ctrl Pts',(-5.05798068443997,-11.9542499791808,
10.9533324843183));
#51143=CARTESIAN_POINT('Ctrl Pts',(-5.56967006477166,-11.1708672702625,
11.0056658601024));
#51144=CARTESIAN_POINT('Ctrl Pts',(-6.29337804857255,-10.7764185582883,
11.0579992358865));
#51145=CARTESIAN_POINT('Ctrl Pts',(-7.01708603237344,-10.3819698463141,
11.1103326116706));
#51146=CARTESIAN_POINT('Ctrl Pts',(-7.95281261964353,-10.3764551312839,
11.1626659874547));
#51147=CARTESIAN_POINT('Ctrl Pts',(-8.68101882670376,-10.7625629805529,
11.2149993632387));
#51148=CARTESIAN_POINT('Ctrl Pts',(-9.40922503376398,-11.1486708298218,
11.2673327390228));
#51149=CARTESIAN_POINT('Ctrl Pts',(-9.92991086061434,-11.9264012433898,
11.3196661148069));
#51150=CARTESIAN_POINT('Ctrl Pts',(-10.0096270834841,-12.7466319657112,
11.371999490591));
#51151=CARTESIAN_POINT('Ctrl Pts',(-10.0174551121829,-12.8271775485652,
11.3771385595633));
#51152=CARTESIAN_POINT('Ctrl Pts',(-10.0210308785667,-12.9081329611663,
11.3822776285357));
#51153=CARTESIAN_POINT('Ctrl Pts',(-10.0205077525331,-12.989132710429,11.387416697508));
#51154=CARTESIAN_POINT('Ctrl Pts',(-8.29379928253297,-15.9596040105122,
12.));
#51155=CARTESIAN_POINT('Ctrl Pts',(-9.27014005842316,-15.698586694035,11.9476666242159));
#51156=CARTESIAN_POINT('Ctrl Pts',(-10.9293914260692,-14.1433745388278,
11.8429998726477));
#51157=CARTESIAN_POINT('Ctrl Pts',(-10.3529516457367,-10.7599545073216,
11.6859997452955));
#51158=CARTESIAN_POINT('Ctrl Pts',(-7.21365210721562,-9.38337955935061,
11.5289996179432));
#51159=CARTESIAN_POINT('Ctrl Pts',(-4.33342685529555,-11.2379164301912,
11.371999490591));
#51160=CARTESIAN_POINT('Ctrl Pts',(-4.29152503935676,-14.6655878811314,
11.2149993632387));
#51161=CARTESIAN_POINT('Ctrl Pts',(-7.12729256983938,-16.5902267633183,
11.0579992358865));
#51162=CARTESIAN_POINT('Ctrl Pts',(-10.296964344732,-15.2872880462285,10.9009991085342));
#51163=CARTESIAN_POINT('Ctrl Pts',(-10.9587277612158,-11.9244666973206,
10.743998981182));
#51164=CARTESIAN_POINT('Ctrl Pts',(-8.51893689306524,-9.51757549146244,
10.5869988538297));
#51165=CARTESIAN_POINT('Ctrl Pts',(-5.16549637569413,-10.2247238388162,
10.4299987264775));
#51166=CARTESIAN_POINT('Ctrl Pts',(-3.90540678666615,-13.4118934459175,
10.2729985991252));
#51167=CARTESIAN_POINT('Ctrl Pts',(-5.86863408021139,-16.2210735713392,
10.115998471773));
#51168=CARTESIAN_POINT('Ctrl Pts',(-9.29471739586239,-16.133268532241,9.9589983444207));
#51169=CARTESIAN_POINT('Ctrl Pts',(-11.1114631891741,-13.227202153015,9.80199821706844));
#51170=CARTESIAN_POINT('Ctrl Pts',(-9.68977387121298,-10.1087780633504,
9.64499808971621));
#51171=CARTESIAN_POINT('Ctrl Pts',(-6.30449404219616,-9.57431398106461,
9.48799796236394));
#51172=CARTESIAN_POINT('Ctrl Pts',(-3.99123550321764,-12.1030705501041,
9.33099783501171));
#51173=CARTESIAN_POINT('Ctrl Pts',(-4.82431993989319,-15.4274866909495,
9.17399770765942));
#51174=CARTESIAN_POINT('Ctrl Pts',(-8.05671225877921,-16.5665269680756,
9.0169975803072));
#51175=CARTESIAN_POINT('Ctrl Pts',(-10.789895403928,-14.4988028275178,8.85999745295491));
#51176=CARTESIAN_POINT('Ctrl Pts',(-10.5729977532197,-11.0784624502813,
8.70299732560269));
#51177=CARTESIAN_POINT('Ctrl Pts',(-7.60051354913579,-9.37255781103892,
8.54599719825042));
#51178=CARTESIAN_POINT('Ctrl Pts',(-4.53789787464541,-10.9107899935683,
8.38899707089818));
#51179=CARTESIAN_POINT('Ctrl Pts',(-4.13142759646044,-14.3138114282651,
8.23199694354591));
#51180=CARTESIAN_POINT('Ctrl Pts',(-6.74558850742372,-16.5301001550025,
8.07499681619368));
#51181=CARTESIAN_POINT('Ctrl Pts',(-10.0362374421571,-15.5722888063543,
7.9179966888414));
#51182=CARTESIAN_POINT('Ctrl Pts',(-11.0526179305001,-12.2992560099981,
7.76099656148917));
#51183=CARTESIAN_POINT('Ctrl Pts',(-8.88333183851511,-9.64596167231467,
7.60399643413689));
#51184=CARTESIAN_POINT('Ctrl Pts',(-5.47359881574229,-9.99164028328652,
7.44699630678467));
#51185=CARTESIAN_POINT('Ctrl Pts',(-3.88095917534459,-13.0263185113509,
7.28999617943238));
#51186=CARTESIAN_POINT('Ctrl Pts',(-5.53354816193247,-16.0287712850697,
7.13299605208016));
#51187=CARTESIAN_POINT('Ctrl Pts',(-8.94947337693327,-16.3066703804957,
6.97599592472788));
#51188=CARTESIAN_POINT('Ctrl Pts',(-11.0656419093738,-13.610821046919,6.81899579737565));
#51189=CARTESIAN_POINT('Ctrl Pts',(-9.98446513414696,-10.3586171776818,
6.66199567002337));
#51190=CARTESIAN_POINT('Ctrl Pts',(-6.67544463886838,-9.46634131342536,
6.50499554267114));
#51191=CARTESIAN_POINT('Ctrl Pts',(-4.10581084513197,-11.7341055256468,
6.34799541531887));
#51192=CARTESIAN_POINT('Ctrl Pts',(-4.57977903131249,-15.1283843904584,
6.19099528796663));
#51193=CARTESIAN_POINT('Ctrl Pts',(-7.67233737080682,-16.6054945057935,
6.03399516061437));
#51194=CARTESIAN_POINT('Ctrl Pts',(-10.610359145649,-14.8408989797994,5.87699503326212));
#51195=CARTESIAN_POINT('Ctrl Pts',(-10.7592920173832,-11.4169237933092,
5.71999490590986));
#51196=CARTESIAN_POINT('Ctrl Pts',(-7.98558650367391,-9.40388769480238,
5.56299477855761));
#51197=CARTESIAN_POINT('Ctrl Pts',(-4.77645084555843,-10.6068850809164,
5.40599465120535));
#51198=CARTESIAN_POINT('Ctrl Pts',(-4.00954797596254,-13.9472048059447,
5.24899452385311));
#51199=CARTESIAN_POINT('Ctrl Pts',(-6.37256666156175,-16.4294950347898,
5.09199439650084));
#51200=CARTESIAN_POINT('Ctrl Pts',(-9.74656614790733,-15.8279701198543,
4.9349942691486));
#51201=CARTESIAN_POINT('Ctrl Pts',(-11.1060472187217,-12.6818122309103,
4.77799414179634));
#51202=CARTESIAN_POINT('Ctrl Pts',(-9.23195310627391,-9.81262424147309,
4.62099401444409));
#51203=CARTESIAN_POINT('Ctrl Pts',(-5.80479621412607,-9.79242646017958,
4.46399388709183));
#51204=CARTESIAN_POINT('Ctrl Pts',(-3.89775220169895,-12.6409121056472,
4.30699375973959));
#51205=CARTESIAN_POINT('Ctrl Pts',(-5.22086478169416,-15.8007186832344,
4.14999363238732));
#51206=CARTESIAN_POINT('Ctrl Pts',(-8.58771683219162,-16.4445101479194,
3.99299350503508));
#51207=CARTESIAN_POINT('Ctrl Pts',(-10.979271517566,-13.9827465287205,3.83599337768283));
#51208=CARTESIAN_POINT('Ctrl Pts',(-10.4928159504458,-11.7612243186229,
3.73132662611465));
#51209=CARTESIAN_POINT('Ctrl Pts',(-9.83606265769611,-10.9930794998359,
3.67899325033057));
#51210=CARTESIAN_POINT('Ctrl Pts',(-8.24593285434704,-15.7805586266087,
12.1070022498898));
#51211=CARTESIAN_POINT('Ctrl Pts',(-9.16339987378206,-15.5352807633023,
12.0546688741057));
#51212=CARTESIAN_POINT('Ctrl Pts',(-10.7225976911422,-14.0738485504296,
11.9500021225376));
#51213=CARTESIAN_POINT('Ctrl Pts',(-10.180917470255,-10.8944501595629,11.7930019951853));
#51214=CARTESIAN_POINT('Ctrl Pts',(-7.23091900471447,-9.60088325574055,
11.6360018678331));
#51215=CARTESIAN_POINT('Ctrl Pts',(-4.52437253811706,-11.3435907789116,
11.4790017404808));
#51216=CARTESIAN_POINT('Ctrl Pts',(-4.48499741917537,-14.5645722101431,
11.3220016131286));
#51217=CARTESIAN_POINT('Ctrl Pts',(-7.14976698350127,-16.3731545641054,
11.1650014857763));
#51218=CARTESIAN_POINT('Ctrl Pts',(-10.1283062268782,-15.1487835956953,
11.008001358424));
#51219=CARTESIAN_POINT('Ctrl Pts',(-10.7501650330301,-11.9887417782655,
10.8510012310718));
#51220=CARTESIAN_POINT('Ctrl Pts',(-8.45749457295849,-9.72698711711278,
10.6940011037196));
#51221=CARTESIAN_POINT('Ctrl Pts',(-5.30626791900676,-10.3914941238528,
10.5370009763673));
#51222=CARTESIAN_POINT('Ctrl Pts',(-4.12216225834487,-13.3864760728501,
10.380000849015));
#51223=CARTESIAN_POINT('Ctrl Pts',(-5.96700612634799,-16.0262614637418,
10.2230007216628));
#51224=CARTESIAN_POINT('Ctrl Pts',(-9.18649518751149,-15.9437511051639,
10.0660005943105));
#51225=CARTESIAN_POINT('Ctrl Pts',(-10.8936904509082,-13.2129217420271,
9.90900046695826));
#51226=CARTESIAN_POINT('Ctrl Pts',(-9.55772959244346,-10.2825399270605,
9.75200033960601));
#51227=CARTESIAN_POINT('Ctrl Pts',(-6.37658355063268,-9.78030425210093,
9.59500021225375));
#51228=CARTESIAN_POINT('Ctrl Pts',(-4.20281546745071,-12.1565757441505,
9.43800008490151));
#51229=CARTESIAN_POINT('Ctrl Pts',(-4.9856645647421,-15.2805282036001,9.28099995754924));
#51230=CARTESIAN_POINT('Ctrl Pts',(-8.02314227712081,-16.3508838764116,
9.12399983019701));
#51231=CARTESIAN_POINT('Ctrl Pts',(-10.5915133373824,-14.4078443649032,
8.96699970284473));
#51232=CARTESIAN_POINT('Ctrl Pts',(-10.387694705577,-11.1937519405699,8.8099995754925));
#51233=CARTESIAN_POINT('Ctrl Pts',(-7.59445254015368,-9.59071406337065,
8.65299944814022));
#51234=CARTESIAN_POINT('Ctrl Pts',(-4.71651386962368,-11.0361902030079,
8.49599932078799));
#51235=CARTESIAN_POINT('Ctrl Pts',(-4.33455391893407,-14.2340080242683,
8.33899919343572));
#51236=CARTESIAN_POINT('Ctrl Pts',(-6.79107983542896,-16.3166536153767,
8.18199906608348));
#51237=CARTESIAN_POINT('Ctrl Pts',(-9.88330126539458,-15.4165986909841,
8.02499893873122));
#51238=CARTESIAN_POINT('Ctrl Pts',(-10.8383935859029,-12.340931138896,7.86799881137898));
#51239=CARTESIAN_POINT('Ctrl Pts',(-8.79991635104542,-9.84763155765228,
7.7109986840267));
#51240=CARTESIAN_POINT('Ctrl Pts',(-5.59579165327249,-10.1724656040451,
7.55399855667448));
#51241=CARTESIAN_POINT('Ctrl Pts',(-4.09918884819405,-13.0241514678338,
7.3969984293222));
#51242=CARTESIAN_POINT('Ctrl Pts',(-5.65212602885569,-15.8455550856297,
7.23999830196996));
#51243=CARTESIAN_POINT('Ctrl Pts',(-8.8620695270797,-16.1066967495653,7.0829981746177));
#51244=CARTESIAN_POINT('Ctrl Pts',(-10.8506322134124,-13.5734082564495,
6.92599804726545));
#51245=CARTESIAN_POINT('Ctrl Pts',(-9.83465084917482,-10.517313638478,6.76899791991319));
#51246=CARTESIAN_POINT('Ctrl Pts',(-6.72516567143593,-9.67884238140407,
6.61199779256095));
#51247=CARTESIAN_POINT('Ctrl Pts',(-4.31048186840692,-11.8098594647285,
6.45499766520868));
#51248=CARTESIAN_POINT('Ctrl Pts',(-4.75586957505634,-14.999461896718,6.29799753785644));
#51249=CARTESIAN_POINT('Ctrl Pts',(-7.66194535538809,-16.3875016553343,
6.14099741050417));
#51250=CARTESIAN_POINT('Ctrl Pts',(-10.4228031904426,-14.7293119763608,
5.98399728315194));
#51251=CARTESIAN_POINT('Ctrl Pts',(-10.5627553478246,-11.5118039232893,
5.82699715579966));
#51252=CARTESIAN_POINT('Ctrl Pts',(-7.95630543474677,-9.62015474206144,
5.66999702844743));
#51253=CARTESIAN_POINT('Ctrl Pts',(-4.94068199678335,-10.7506108834838,
5.51299690109516));
#51254=CARTESIAN_POINT('Ctrl Pts',(-4.22002369044277,-13.8895079343495,
5.35599677374291));
#51255=CARTESIAN_POINT('Ctrl Pts',(-6.44055136262695,-16.2221150259203,
5.19899664639066));
#51256=CARTESIAN_POINT('Ctrl Pts',(-9.61109727113964,-15.6568623145209,
5.04199651903841));
#51257=CARTESIAN_POINT('Ctrl Pts',(-10.8886010657355,-12.7004190599517,
4.88499639168614));
#51258=CARTESIAN_POINT('Ctrl Pts',(-9.12751561079228,-10.0042443043008,
4.72799626433391));
#51259=CARTESIAN_POINT('Ctrl Pts',(-5.90701771024297,-9.98526445765287,
4.57099613698164));
#51260=CARTESIAN_POINT('Ctrl Pts',(-4.11496924804734,-12.6619852293197,
4.4139960096294));
#51261=CARTESIAN_POINT('Ctrl Pts',(-5.35829758700603,-15.631254150908,4.25699588227714));
#51262=CARTESIAN_POINT('Ctrl Pts',(-8.52212705303664,-16.2362247214587,
4.09999575492489));
#51263=CARTESIAN_POINT('Ctrl Pts',(-10.7694699922944,-13.9229064764016,
3.94299562757263));
#51264=CARTESIAN_POINT('Ctrl Pts',(-10.31234789899,-11.8353429831647,3.83832887600446));
#51265=CARTESIAN_POINT('Ctrl Pts',(-9.69519710401908,-11.1135176176878,
3.78599550022038));
#51266=CARTESIAN_POINT('Ctrl Pts',(-8.19806642616111,-15.6015132427052,
12.2140044997796));
#51267=CARTESIAN_POINT('Ctrl Pts',(-9.05665968914096,-15.3719748325695,
12.1616711239955));
#51268=CARTESIAN_POINT('Ctrl Pts',(-10.5158039562152,-14.0043225620313,
12.0570043724274));
#51269=CARTESIAN_POINT('Ctrl Pts',(-10.0088832947732,-11.0289458118043,
11.9000042450751));
#51270=CARTESIAN_POINT('Ctrl Pts',(-7.24818590221332,-9.81838695213045,
11.7430041177229));
#51271=CARTESIAN_POINT('Ctrl Pts',(-4.71531822093855,-11.4492651276319,
11.5860039903706));
#51272=CARTESIAN_POINT('Ctrl Pts',(-4.67846979899401,-14.4635565391549,
11.4290038630183));
#51273=CARTESIAN_POINT('Ctrl Pts',(-7.17224139716313,-16.1560823648925,
11.2720037356661));
#51274=CARTESIAN_POINT('Ctrl Pts',(-9.95964810902439,-15.0102791451622,
11.1150036083138));
#51275=CARTESIAN_POINT('Ctrl Pts',(-10.5416023048445,-12.0530168592103,
10.9580034809616));
#51276=CARTESIAN_POINT('Ctrl Pts',(-8.39605225285175,-9.93639874276315,
10.8010033536093));
#51277=CARTESIAN_POINT('Ctrl Pts',(-5.44703946231937,-10.5582644088895,
10.6440032262571));
#51278=CARTESIAN_POINT('Ctrl Pts',(-4.3389177300236,-13.3610586997827,10.4870030989048));
#51279=CARTESIAN_POINT('Ctrl Pts',(-6.06537817248458,-15.8314493561443,
10.3300029715526));
#51280=CARTESIAN_POINT('Ctrl Pts',(-9.07827297916059,-15.7542336780869,
10.1730028442003));
#51281=CARTESIAN_POINT('Ctrl Pts',(-10.6759177126423,-13.1986413310391,
10.0160027168481));
#51282=CARTESIAN_POINT('Ctrl Pts',(-9.42568531367393,-10.4563017907707,
9.85900258949582));
#51283=CARTESIAN_POINT('Ctrl Pts',(-6.44867305906919,-9.98629452313723,
9.70200246214357));
#51284=CARTESIAN_POINT('Ctrl Pts',(-4.41439543168378,-12.2100809381968,
9.54500233479132));
#51285=CARTESIAN_POINT('Ctrl Pts',(-5.14700918959101,-15.1335697162506,
9.38800220743905));
#51286=CARTESIAN_POINT('Ctrl Pts',(-7.98957229546242,-16.1352407847476,
9.23100208008682));
#51287=CARTESIAN_POINT('Ctrl Pts',(-10.3931312708367,-14.3168859022886,
9.07400195273454));
#51288=CARTESIAN_POINT('Ctrl Pts',(-10.2023916579342,-11.3090414308585,
8.91700182538231));
#51289=CARTESIAN_POINT('Ctrl Pts',(-7.58839153117158,-9.80887031570234,
8.76000169803004));
#51290=CARTESIAN_POINT('Ctrl Pts',(-4.89512986460196,-11.1615904124476,
8.6030015706778));
#51291=CARTESIAN_POINT('Ctrl Pts',(-4.53768024140768,-14.1542046202714,
8.44600144332553));
#51292=CARTESIAN_POINT('Ctrl Pts',(-6.83657116343421,-16.103207075751,8.28900131597329));
#51293=CARTESIAN_POINT('Ctrl Pts',(-9.730365088632,-15.2609085756139,8.13200118862103));
#51294=CARTESIAN_POINT('Ctrl Pts',(-10.6241692413057,-12.3826062677939,
7.97500106126879));
#51295=CARTESIAN_POINT('Ctrl Pts',(-8.71650086357571,-10.0493014429898,
7.81800093391652));
#51296=CARTESIAN_POINT('Ctrl Pts',(-5.7179844908027,-10.3532909248038,7.66100080656428));
#51297=CARTESIAN_POINT('Ctrl Pts',(-4.31741852104351,-13.0219844243168,
7.50400067921201));
#51298=CARTESIAN_POINT('Ctrl Pts',(-5.7707038957789,-15.6623388861897,7.34700055185977));
#51299=CARTESIAN_POINT('Ctrl Pts',(-8.77466567722613,-15.9067231186349,
7.19000042450751));
#51300=CARTESIAN_POINT('Ctrl Pts',(-10.635622517451,-13.5359954659799,7.03300029715527));
#51301=CARTESIAN_POINT('Ctrl Pts',(-9.68483656420267,-10.6760100992742,
6.87600016980299));
#51302=CARTESIAN_POINT('Ctrl Pts',(-6.77488670400349,-9.89134344938279,
6.71900004245076));
#51303=CARTESIAN_POINT('Ctrl Pts',(-4.51515289168187,-11.8856134038101,
6.56199991509849));
#51304=CARTESIAN_POINT('Ctrl Pts',(-4.93196011880019,-14.8705394029777,
6.40499978774625));
#51305=CARTESIAN_POINT('Ctrl Pts',(-7.65155333996934,-16.1695088048751,
6.24799966039398));
#51306=CARTESIAN_POINT('Ctrl Pts',(-10.2352472352362,-14.6177249729221,
6.09099953304175));
#51307=CARTESIAN_POINT('Ctrl Pts',(-10.366218678266,-11.6066840532695,5.93399940568948));
#51308=CARTESIAN_POINT('Ctrl Pts',(-7.92702436581964,-9.83642178932047,
5.77699927833724));
#51309=CARTESIAN_POINT('Ctrl Pts',(-5.10491314800829,-10.8943366860512,
5.61999915098497));
#51310=CARTESIAN_POINT('Ctrl Pts',(-4.43049940492298,-13.8318110627544,
5.46299902363273));
#51311=CARTESIAN_POINT('Ctrl Pts',(-6.50853606369215,-16.0147350170509,
5.30599889628046));
#51312=CARTESIAN_POINT('Ctrl Pts',(-9.47562839437195,-15.4857545091874,
5.14899876892823));
#51313=CARTESIAN_POINT('Ctrl Pts',(-10.6711549127493,-12.7190258889931,
4.99199864157595));
#51314=CARTESIAN_POINT('Ctrl Pts',(-9.02307811531067,-10.1958643671286,
4.83499851422372));
#51315=CARTESIAN_POINT('Ctrl Pts',(-6.00923920635987,-10.1781024551261,
4.67799838687145));
#51316=CARTESIAN_POINT('Ctrl Pts',(-4.33218629439574,-12.6830583529922,
4.52099825951921));
#51317=CARTESIAN_POINT('Ctrl Pts',(-5.49573039231789,-15.4617896185815,
4.36399813216695));
#51318=CARTESIAN_POINT('Ctrl Pts',(-8.45653727388165,-16.027939294998,4.2069980048147));
#51319=CARTESIAN_POINT('Ctrl Pts',(-10.5596684670228,-13.8630664240827,
4.04999787746245));
#51320=CARTESIAN_POINT('Ctrl Pts',(-10.1318798475343,-11.9094616477065,
3.94533112589428));
#51321=CARTESIAN_POINT('Ctrl Pts',(-9.55433155034205,-11.2339557355397,
3.89299775011019));
#51322=CARTESIAN_POINT('Ctrl Pts',(-8.15019999797519,-15.4224678588016,
12.3210067496694));
#51323=CARTESIAN_POINT('Ctrl Pts',(-8.94991950449986,-15.2086689018368,
12.2686733738853));
#51324=CARTESIAN_POINT('Ctrl Pts',(-10.3090102212882,-13.934796573633,12.1640066223172));
#51325=CARTESIAN_POINT('Ctrl Pts',(-9.83684911929144,-11.1634414640457,
12.0070064949649));
#51326=CARTESIAN_POINT('Ctrl Pts',(-7.26545279971217,-10.0358906485204,
11.8500063676127));
#51327=CARTESIAN_POINT('Ctrl Pts',(-4.90626390376006,-11.5549394763523,
11.6930062402604));
#51328=CARTESIAN_POINT('Ctrl Pts',(-4.87194217881263,-14.3625408681667,
11.5360061129082));
#51329=CARTESIAN_POINT('Ctrl Pts',(-7.19471581082501,-15.9390101656796,
11.3790059855559));
#51330=CARTESIAN_POINT('Ctrl Pts',(-9.7909899911706,-14.871774694629,11.2220058582037));
#51331=CARTESIAN_POINT('Ctrl Pts',(-10.3330395766588,-12.1172919401552,
11.0650057308514));
#51332=CARTESIAN_POINT('Ctrl Pts',(-8.334609932745,-10.1458103684135,10.9080056034992));
#51333=CARTESIAN_POINT('Ctrl Pts',(-5.587811005632,-10.7250346939262,10.7510054761469));
#51334=CARTESIAN_POINT('Ctrl Pts',(-4.55567320170231,-13.3356413267153,
10.5940053487946));
#51335=CARTESIAN_POINT('Ctrl Pts',(-6.16375021862117,-15.6366372485469,
10.4370052214424));
#51336=CARTESIAN_POINT('Ctrl Pts',(-8.97005077080969,-15.5647162510099,
10.2800050940901));
#51337=CARTESIAN_POINT('Ctrl Pts',(-10.4581449743764,-13.1843609200512,
10.1230049667379));
#51338=CARTESIAN_POINT('Ctrl Pts',(-9.29364103490441,-10.6300636544808,
9.96600483938564));
#51339=CARTESIAN_POINT('Ctrl Pts',(-6.52076256750571,-10.1922847941736,
9.80900471203337));
#51340=CARTESIAN_POINT('Ctrl Pts',(-4.62597539591685,-12.2635861322432,
9.65200458468114));
#51341=CARTESIAN_POINT('Ctrl Pts',(-5.30835381443992,-14.9866112289011,
9.49500445732886));
#51342=CARTESIAN_POINT('Ctrl Pts',(-7.95600231380402,-15.9195976930836,
9.33800432997663));
#51343=CARTESIAN_POINT('Ctrl Pts',(-10.1947492042911,-14.2259274396741,
9.18100420262435));
#51344=CARTESIAN_POINT('Ctrl Pts',(-10.0170886102914,-11.424330921147,9.02400407527213));
#51345=CARTESIAN_POINT('Ctrl Pts',(-7.58233052218947,-10.0270265680341,
8.86700394791983));
#51346=CARTESIAN_POINT('Ctrl Pts',(-5.07374585958023,-11.2869906218872,
8.71000382056763));
#51347=CARTESIAN_POINT('Ctrl Pts',(-4.7408065638813,-14.0744012162745,8.55300369321533));
#51348=CARTESIAN_POINT('Ctrl Pts',(-6.88206249143947,-15.8897605361253,
8.39600356586311));
#51349=CARTESIAN_POINT('Ctrl Pts',(-9.57742891186941,-15.1052184602437,
8.23900343851083));
#51350=CARTESIAN_POINT('Ctrl Pts',(-10.4099448967086,-12.4242813966918,
8.0820033111586));
#51351=CARTESIAN_POINT('Ctrl Pts',(-8.633085376106,-10.2509713283274,7.92500318380633));
#51352=CARTESIAN_POINT('Ctrl Pts',(-5.84017732833291,-10.5341162455624,
7.7680030564541));
#51353=CARTESIAN_POINT('Ctrl Pts',(-4.53564819389297,-13.0198173807997,
7.61100292910182));
#51354=CARTESIAN_POINT('Ctrl Pts',(-5.88928176270212,-15.4791226867497,
7.45400280174959));
#51355=CARTESIAN_POINT('Ctrl Pts',(-8.68726182737255,-15.7067494877046,
7.29700267439731));
#51356=CARTESIAN_POINT('Ctrl Pts',(-10.4206128214897,-13.4985826755103,
7.14000254704508));
#51357=CARTESIAN_POINT('Ctrl Pts',(-9.53502227923051,-10.8347065600703,
6.9830024196928));
#51358=CARTESIAN_POINT('Ctrl Pts',(-6.82460773657105,-10.1038445173615,
6.82600229234058));
#51359=CARTESIAN_POINT('Ctrl Pts',(-4.71982391495681,-11.9613673428918,
6.66900216498829));
#51360=CARTESIAN_POINT('Ctrl Pts',(-5.10805066254405,-14.7416169092374,
6.51200203763607));
#51361=CARTESIAN_POINT('Ctrl Pts',(-7.64116132455058,-15.9515159544159,
6.35500191028379));
#51362=CARTESIAN_POINT('Ctrl Pts',(-10.0476912800297,-14.5061379694834,
6.19800178293156));
#51363=CARTESIAN_POINT('Ctrl Pts',(-10.1696820087074,-11.7015641832497,
6.04100165557928));
#51364=CARTESIAN_POINT('Ctrl Pts',(-7.8977432968925,-10.0526888365795,5.88400152822706));
#51365=CARTESIAN_POINT('Ctrl Pts',(-5.26914429923322,-11.0380624886186,
5.72700140087478));
#51366=CARTESIAN_POINT('Ctrl Pts',(-4.6409751194032,-13.7741141911592,5.57000127352254));
#51367=CARTESIAN_POINT('Ctrl Pts',(-6.57652076475734,-15.8073550081814,
5.41300114617028));
#51368=CARTESIAN_POINT('Ctrl Pts',(-9.34015951760427,-15.314646703854,5.25600101881803));
#51369=CARTESIAN_POINT('Ctrl Pts',(-10.4537087597631,-12.7376327180345,
5.09900089146577));
#51370=CARTESIAN_POINT('Ctrl Pts',(-8.91864061982905,-10.3874844299563,
4.94200076411353));
#51371=CARTESIAN_POINT('Ctrl Pts',(-6.11146070247677,-10.3709404525994,
4.78500063676126));
#51372=CARTESIAN_POINT('Ctrl Pts',(-4.54940334074414,-12.7041314766647,
4.62800050940902));
#51373=CARTESIAN_POINT('Ctrl Pts',(-5.63316319762975,-15.2923250862551,
4.47100038205676));
#51374=CARTESIAN_POINT('Ctrl Pts',(-8.39094749472666,-15.8196538685372,
4.31400025470451));
#51375=CARTESIAN_POINT('Ctrl Pts',(-10.3498669417512,-13.8032263717638,
4.15700012735226));
#51376=CARTESIAN_POINT('Ctrl Pts',(-9.95141179607851,-11.9835803122483,
4.05233337578409));
#51377=CARTESIAN_POINT('Ctrl Pts',(-9.41346599666503,-11.3543938533916,
4.));
#51378=CARTESIAN_POINT('Ctrl Pts',(-10.0159021674261,-12.9883695445715,
11.112583302492));
#51379=CARTESIAN_POINT('Ctrl Pts',(-10.0178571377502,-12.737164469747,11.0967241119451));
#51380=CARTESIAN_POINT('Ctrl Pts',(-9.98318366513377,-12.4864861117061,
11.0808649213983));
#51381=CARTESIAN_POINT('Ctrl Pts',(-9.90962637175846,-12.2477921372772,
11.0650057308514));
#51382=CARTESIAN_POINT('Ctrl Pts',(-9.66689636202086,-11.4601314162413,
11.0126723550673));
#51383=CARTESIAN_POINT('Ctrl Pts',(-9.00075314738293,-10.8029708923274,
10.9603389792832));
#51384=CARTESIAN_POINT('Ctrl Pts',(-8.20988171887847,-10.5709280179559,
10.9080056034991));
#51385=CARTESIAN_POINT('Ctrl Pts',(-7.419010290374,-10.3388851435844,10.8556722277151));
#51386=CARTESIAN_POINT('Ctrl Pts',(-6.503410648003,-10.5319599187553,10.803338851931));
#51387=CARTESIAN_POINT('Ctrl Pts',(-5.87358785949589,-11.0635984118056,
10.7510054761469));
#51388=CARTESIAN_POINT('Ctrl Pts',(-5.24376507098877,-11.5952369048559,
10.6986721003628));
#51389=CARTESIAN_POINT('Ctrl Pts',(-4.89971913634554,-12.4654391157856,
10.6463387245787));
#51390=CARTESIAN_POINT('Ctrl Pts',(-4.99570900517707,-13.2840395415557,
10.5940053487946));
#51391=CARTESIAN_POINT('Ctrl Pts',(-5.0916988740086,-14.1026399673258,10.5416719730106));
#51392=CARTESIAN_POINT('Ctrl Pts',(-5.62772454631489,-14.8696386079364,
10.4893385972265));
#51393=CARTESIAN_POINT('Ctrl Pts',(-6.36345414116612,-15.2411510953188,
10.4370052214424));
#51394=CARTESIAN_POINT('Ctrl Pts',(-7.09918373601734,-15.6126635827012,
10.3846718456583));
#51395=CARTESIAN_POINT('Ctrl Pts',(-8.03461725341351,-15.5886899168556,
10.3323384698742));
#51396=CARTESIAN_POINT('Ctrl Pts',(-8.75034971270605,-15.1799771954396,
10.2800050940901));
#51397=CARTESIAN_POINT('Ctrl Pts',(-9.46608217199859,-14.7712644740237,
10.2276717183061));
#51398=CARTESIAN_POINT('Ctrl Pts',(-9.96211357318751,-13.9778126970374,
10.175338342522));
#51399=CARTESIAN_POINT('Ctrl Pts',(-10.01604528387,-13.1553705976159,10.1230049667379));
#51400=CARTESIAN_POINT('Ctrl Pts',(-10.0196252693796,-13.1007769130985,
10.1195310786559));
#51401=CARTESIAN_POINT('Ctrl Pts',(-10.0212572306508,-13.0460554884989,
10.1160571905739));
#51402=CARTESIAN_POINT('Ctrl Pts',(-10.0209920718673,-12.9913179799917,
10.112583302492));
#51403=CARTESIAN_POINT('Ctrl Pts',(-8.29379928253297,-15.9596040105122,
12.));
#51404=CARTESIAN_POINT('Ctrl Pts',(-8.38688146826619,-15.9255541311756,
12.));
#51405=CARTESIAN_POINT('Ctrl Pts',(-8.47790052796864,-15.8867414890058,
12.));
#51406=CARTESIAN_POINT('Ctrl Pts',(-8.56664663605253,-15.843492548424,12.));
#51407=CARTESIAN_POINT('Ctrl Pts',(-8.65733876929825,-15.7992952448277,
12.));
#51408=CARTESIAN_POINT('Ctrl Pts',(-8.74565784480789,-15.750464336337,12.));
#51409=CARTESIAN_POINT('Ctrl Pts',(-8.83135101694567,-15.6973027457218,
12.));
#51410=CARTESIAN_POINT('Ctrl Pts',(-8.91318960012018,-15.6465324317433,
12.));
#51411=CARTESIAN_POINT('Ctrl Pts',(-8.99263343720554,-15.5918113841942,
12.));
#51412=CARTESIAN_POINT('Ctrl Pts',(-9.069430157416,-15.533374159028,12.));
#51413=CARTESIAN_POINT('Ctrl Pts',(-9.13662728760015,-15.4822415870076,
12.));
#51414=CARTESIAN_POINT('Ctrl Pts',(-9.20179743619592,-15.4282631425356,
12.));
#51415=CARTESIAN_POINT('Ctrl Pts',(-9.26474763112753,-15.3715835638146,
12.));
#51416=CARTESIAN_POINT('Ctrl Pts',(-9.27985611388604,-15.3579800723751,
12.));
#51417=CARTESIAN_POINT('Ctrl Pts',(-9.29484029179697,-15.3442173582628,
12.));
#51418=CARTESIAN_POINT('Ctrl Pts',(-9.30967505138841,-15.3303185989115,
12.));
#51419=CARTESIAN_POINT('Ctrl Pts',(-9.38210503428163,-15.26245859108,12.));
#51420=CARTESIAN_POINT('Ctrl Pts',(-9.45106917065939,-15.1912779029607,
12.));
#51421=CARTESIAN_POINT('Ctrl Pts',(-9.51632647275336,-15.1170649381822,
12.));
#51422=CARTESIAN_POINT('Ctrl Pts',(-9.58121888012541,-15.0432669448824,
12.));
#51423=CARTESIAN_POINT('Ctrl Pts',(-9.64244627908667,-14.9664696982533,
12.));
#51424=CARTESIAN_POINT('Ctrl Pts',(-9.69972810245665,-14.8869300127004,
12.));
#51425=CARTESIAN_POINT('Ctrl Pts',(-9.75408287639578,-14.81145473323,12.));
#51426=CARTESIAN_POINT('Ctrl Pts',(-9.80488505097158,-14.7335093955071,
12.));
#51427=CARTESIAN_POINT('Ctrl Pts',(-9.85185230919616,-14.6533004074739,
12.));
#51428=CARTESIAN_POINT('Ctrl Pts',(-9.8892295724543,-14.5894688666365,12.));
#51429=CARTESIAN_POINT('Ctrl Pts',(-9.92417736747258,-14.5242033609892,
12.));
#51430=CARTESIAN_POINT('Ctrl Pts',(-9.95653206305223,-14.4576058296606,
12.));
#51431=CARTESIAN_POINT('Ctrl Pts',(-9.96243497650182,-14.4454555233034,
12.));
#51432=CARTESIAN_POINT('Ctrl Pts',(-9.9682498087257,-14.4332643188572,12.));
#51433=CARTESIAN_POINT('Ctrl Pts',(-9.97397236800321,-14.4210401757467,
12.));
#51434=CARTESIAN_POINT('Ctrl Pts',(-10.014548795905,-14.3343635617469,12.));
#51435=CARTESIAN_POINT('Ctrl Pts',(-10.0505434398104,-14.2459232997935,
12.));
#51436=CARTESIAN_POINT('Ctrl Pts',(-10.0816927676552,-14.1559630239742,
12.));
#51437=CARTESIAN_POINT('Ctrl Pts',(-10.1128420955,-14.0660027481548,12.));
#51438=CARTESIAN_POINT('Ctrl Pts',(-10.1391465733587,-13.9745217251954,
12.));
#51439=CARTESIAN_POINT('Ctrl Pts',(-10.1602864633442,-13.8817537764296,
12.));
#51440=CARTESIAN_POINT('Ctrl Pts',(-10.1814515048034,-13.7888754557256,
12.));
#51441=CARTESIAN_POINT('Ctrl Pts',(-10.1974388881398,-13.6947059611701,
12.));
#51442=CARTESIAN_POINT('Ctrl Pts',(-10.2083240537505,-13.5996534977197,
12.));
#51443=CARTESIAN_POINT('Ctrl Pts',(-10.2138911337605,-13.5510401198348,
12.));
#51444=CARTESIAN_POINT('Ctrl Pts',(-10.2181228103627,-13.5021959582282,
12.));
#51445=CARTESIAN_POINT('Ctrl Pts',(-10.221024235662,-13.4531774228974,12.));
#51446=CARTESIAN_POINT('Ctrl Pts',(-10.2218608104944,-13.4390437924411,
12.));
#51447=CARTESIAN_POINT('Ctrl Pts',(-10.2225867738812,-13.4248956759012,
12.));
#51448=CARTESIAN_POINT('Ctrl Pts',(-10.2232022007112,-13.410734453067,12.));
#51449=CARTESIAN_POINT('Ctrl Pts',(-10.2238234019696,-13.3964403582763,
12.));
#51450=CARTESIAN_POINT('Ctrl Pts',(-10.2243315800161,-13.3821418174545,
12.));
#51451=CARTESIAN_POINT('Ctrl Pts',(-10.2247271750585,-13.3678432915664,
12.));
#51452=CARTESIAN_POINT('Ctrl Pts',(-10.2273082491492,-13.2745520448321,
12.));
#51453=CARTESIAN_POINT('Ctrl Pts',(-10.2251029799825,-13.1812181718667,
12.));
#51454=CARTESIAN_POINT('Ctrl Pts',(-10.2182398910409,-13.0882187710056,
12.));
#51455=CARTESIAN_POINT('Ctrl Pts',(-10.2113725866781,-12.9951622483964,
12.));
#51456=CARTESIAN_POINT('Ctrl Pts',(-10.1998413619504,-12.902439631583,12.));
#51457=CARTESIAN_POINT('Ctrl Pts',(-10.1837244231874,-12.810441427736,12.));
#51458=CARTESIAN_POINT('Ctrl Pts',(-10.1678505565058,-12.7198307203121,
12.));
#51459=CARTESIAN_POINT('Ctrl Pts',(-10.1475277985646,-12.629921903999,12.));
#51460=CARTESIAN_POINT('Ctrl Pts',(-10.1227882064871,-12.5411137713789,
12.));
#51461=CARTESIAN_POINT('Ctrl Pts',(-10.1129089207081,-12.5056499319226,
12.));
#51462=CARTESIAN_POINT('Ctrl Pts',(-10.1023248586868,-12.4703619714101,
12.));
#51463=CARTESIAN_POINT('Ctrl Pts',(-10.0910363601597,-12.435276902831,12.));
#51464=CARTESIAN_POINT('Ctrl Pts',(-10.0850884600019,-12.4167906103951,
12.));
#51465=CARTESIAN_POINT('Ctrl Pts',(-10.0789449767355,-12.398360662607,12.));
#51466=CARTESIAN_POINT('Ctrl Pts',(-10.0726058589696,-12.3799911333697,
12.));
#51467=CARTESIAN_POINT('Ctrl Pts',(-10.0672510463096,-12.3644739287129,
12.));
#51468=CARTESIAN_POINT('Ctrl Pts',(-10.0617592067699,-12.349007385008,12.));
#51469=CARTESIAN_POINT('Ctrl Pts',(-10.0561325433239,-12.3335987119335,
12.));
#51470=CARTESIAN_POINT('Ctrl Pts',(-10.0253173441252,-12.2492109864665,
12.));
#51471=CARTESIAN_POINT('Ctrl Pts',(-9.99044488561477,-12.166508346864,12.));
#51472=CARTESIAN_POINT('Ctrl Pts',(-9.95156719631022,-12.0858609769308,
12.));
#51473=CARTESIAN_POINT('Ctrl Pts',(-9.92246136851044,-12.0254842286268,
12.));
#51474=CARTESIAN_POINT('Ctrl Pts',(-9.89110980665403,-11.9662598549223,
12.));
#51475=CARTESIAN_POINT('Ctrl Pts',(-9.85752076592995,-11.9083564676894,
12.));
#51476=CARTESIAN_POINT('Ctrl Pts',(-9.84460179101728,-11.8860857391751,
12.));
#51477=CARTESIAN_POINT('Ctrl Pts',(-9.83135170784992,-11.8640105638195,
12.));
#51478=CARTESIAN_POINT('Ctrl Pts',(-9.81777057146904,-11.8421410854707,
12.));
#51479=CARTESIAN_POINT('Ctrl Pts',(-9.80600924137691,-11.8232020109641,
12.));
#51480=CARTESIAN_POINT('Ctrl Pts',(-9.79399765022805,-11.8044144459084,
12.));
#51481=CARTESIAN_POINT('Ctrl Pts',(-9.78175006557354,-11.7858062660097,
12.));
#51482=CARTESIAN_POINT('Ctrl Pts',(-9.73447815410214,-11.7139844123438,
12.));
#51483=CARTESIAN_POINT('Ctrl Pts',(-9.68365479534874,-11.6447676019631,
12.));
#51484=CARTESIAN_POINT('Ctrl Pts',(-9.62930896131935,-11.578509745124,12.));
#51485=CARTESIAN_POINT('Ctrl Pts',(-9.58717521523442,-11.5271407346737,
12.));
#51486=CARTESIAN_POINT('Ctrl Pts',(-9.54292346973057,-11.477550842089,12.));
#51487=CARTESIAN_POINT('Ctrl Pts',(-9.49655480089338,-11.4299227460007,
12.));
#51488=CARTESIAN_POINT('Ctrl Pts',(-9.47068894114788,-11.4033543392671,
12.));
#51489=CARTESIAN_POINT('Ctrl Pts',(-9.44416412664311,-11.377396721654,12.));
#51490=CARTESIAN_POINT('Ctrl Pts',(-9.41700750114215,-11.3520617378123,
12.));
#51491=CARTESIAN_POINT('Origin',(-7.50000000000001,-12.9903810567666,7.5));
#51492=CARTESIAN_POINT('Origin',(-7.5,12.9903810567666,3.));
#51493=CARTESIAN_POINT('Origin',(15.,0.,3.));
#51494=CARTESIAN_POINT('Origin',(-7.50000000000001,-12.9903810567666,3.));
#51495=CARTESIAN_POINT('Origin',(5.55111512312578E-16,0.,14.));
#51496=CARTESIAN_POINT('',(-5.65685424949238,-6.92764844988394E-16,12.));
#51497=CARTESIAN_POINT('Origin',(5.55111512312578E-16,0.,12.));
#51498=CARTESIAN_POINT('',(1.87717472568372E-16,-4.49927934798557E-32,8.));
#51499=CARTESIAN_POINT('Origin',(5.55111512312578E-16,0.,14.));
#51500=CARTESIAN_POINT('Origin',(0.,0.,0.));
#51501=CARTESIAN_POINT('',(-30.,-3.67394039744206E-15,12.));
#51502=CARTESIAN_POINT('Origin',(0.,0.,12.));
#51503=CARTESIAN_POINT('',(-30.,-3.67394039744206E-15,0.));
#51504=CARTESIAN_POINT('',(-30.,-3.67394039744206E-15,0.));
#51505=CARTESIAN_POINT('Origin',(0.,0.,0.));
#51506=CARTESIAN_POINT('Origin',(0.,0.,12.));
#51507=CARTESIAN_POINT('Origin',(0.,0.,0.));
#63728=UNCERTAINTY_MEASURE_WITH_UNIT(LENGTH_MEASURE(0.01),#63756,
'DISTANCE_ACCURACY_VALUE',
'Maximum model space distance between geometric entities at asserted c
onnectivities');
#63735=UNCERTAINTY_MEASURE_WITH_UNIT(LENGTH_MEASURE(0.01),#63756,
'DISTANCE_ACCURACY_VALUE',
'Maximum model space distance between geometric entities at asserted c
onnectivities');
#63748=(
GEOMETRIC_REPRESENTATION_CONTEXT(3)
GLOBAL_UNCERTAINTY_ASSIGNED_CONTEXT((#63728))
GLOBAL_UNIT_ASSIGNED_CONTEXT((#63756,#63758,#63759))
REPRESENTATION_CONTEXT('','3D')
);
#63755=(
GEOMETRIC_REPRESENTATION_CONTEXT(3)
GLOBAL_UNCERTAINTY_ASSIGNED_CONTEXT((#63735))
GLOBAL_UNIT_ASSIGNED_CONTEXT((#63756,#63758,#63759))
REPRESENTATION_CONTEXT('','3D')
);
#63756=(
LENGTH_UNIT()
NAMED_UNIT(*)
SI_UNIT(.MILLI.,.METRE.)
);
#63758=(
NAMED_UNIT(*)
PLANE_ANGLE_UNIT()
SI_UNIT($,.RADIAN.)
);
#63759=(
NAMED_UNIT(*)
SI_UNIT($,.STERADIAN.)
SOLID_ANGLE_UNIT()
);
#63772=SHAPE_DEFINITION_REPRESENTATION(#63831,#63870);
#63831=PRODUCT_DEFINITION_SHAPE('',$,#63890);
#63870=SHAPE_REPRESENTATION('',(#15145),#63748);
#63877=PRODUCT_DEFINITION_CONTEXT('part definition',#63936,'design');
#63890=PRODUCT_DEFINITION('Swivel pad','Swivel pad',#63909,#63877);
#63909=PRODUCT_DEFINITION_FORMATION('',$,#63950);
#63936=APPLICATION_CONTEXT(
'Core Data for Automotive Mechanical Design Process');
#63937=PRODUCT_CONTEXT('part definition',#63936,'mechanical');
#63950=PRODUCT('Swivel pad','Swivel pad',$,(#63937));
#63962=PRESENTATION_STYLE_ASSIGNMENT((#63969));
#63969=SURFACE_STYLE_USAGE(.BOTH.,#63976);
#63976=SURFACE_SIDE_STYLE('',(#63983));
#63983=SURFACE_STYLE_FILL_AREA(#63990);
#63990=FILL_AREA_STYLE('Gray',(#63997));
#63997=FILL_AREA_STYLE_COLOUR('Gray',#64004);
#64004=COLOUR_RGB('Gray',0.407843137254902,0.447058823529412,0.498039215686275);
ENDSEC;
END-ISO-10303-21;
